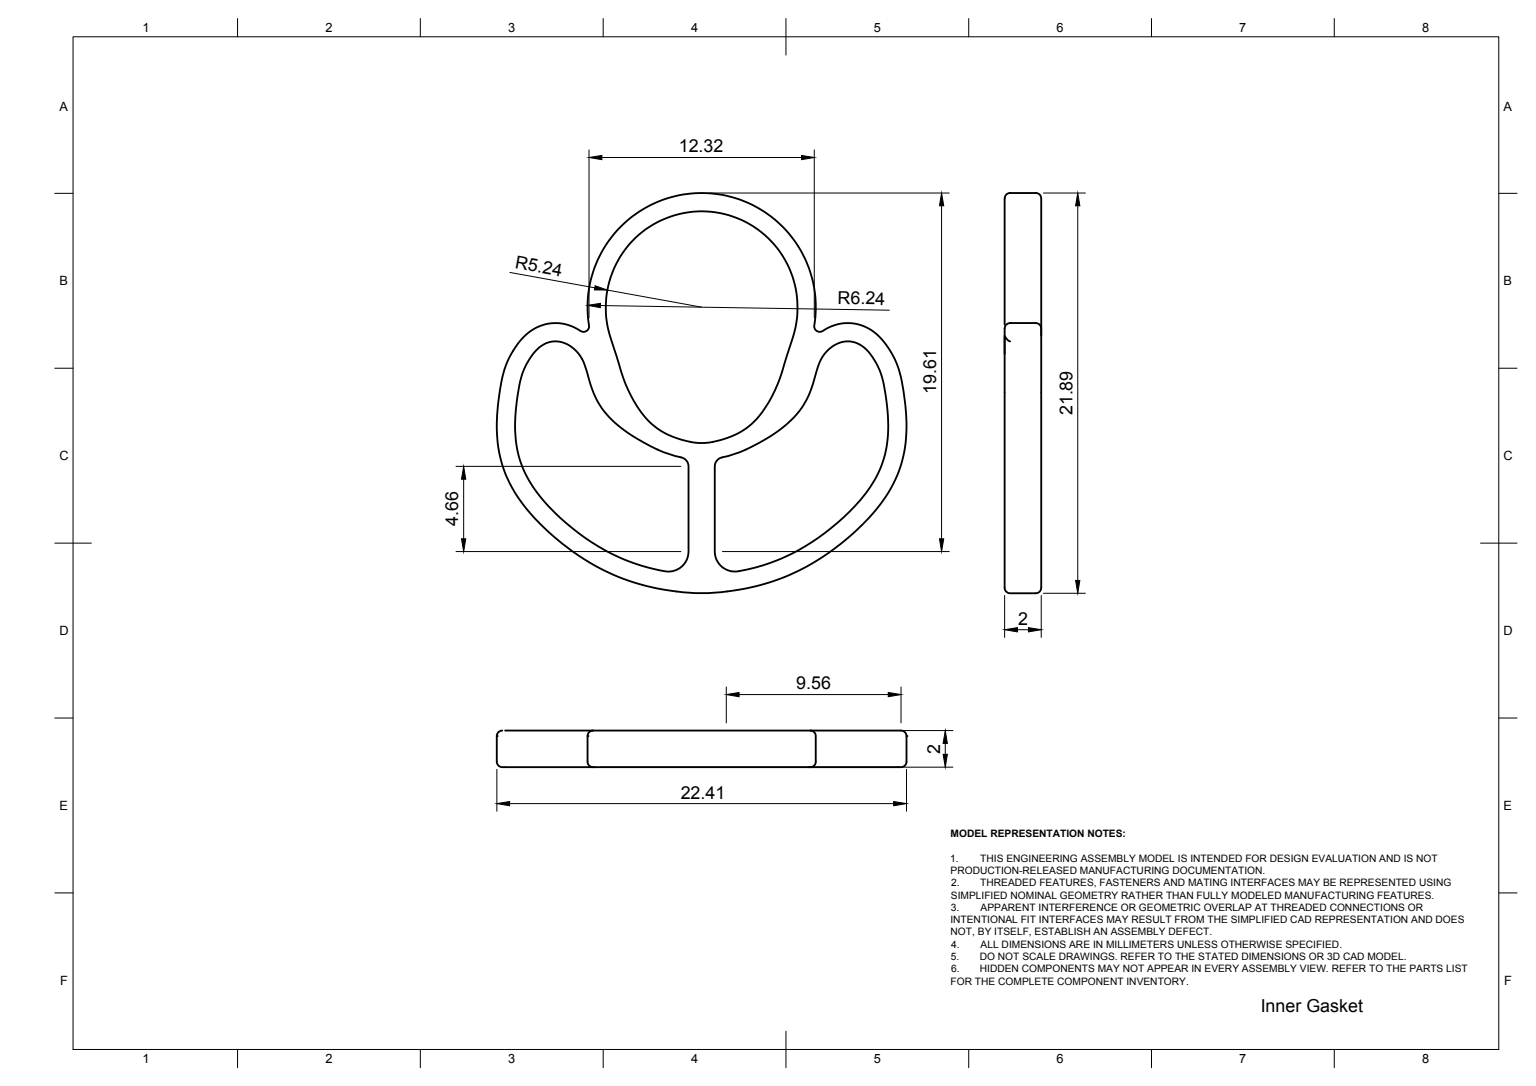
ISO-10303-21;
HEADER;
/* Generated by software containing ST-Developer
 * from STEP Tools, Inc. (www.steptools.com) 
 */

FILE_DESCRIPTION(
/* description */ ('STEP AP214'),
/* implementation_level */ '2;1');

FILE_NAME(
/* name */ 'Inner Gasket.step',
/* time_stamp */ '2026-10-06T00:19:40-07:00',
/* author */ (''),
/* organization */ (''),
/* preprocessor_version */ 'ST-DEVELOPER v20.2',
/* originating_system */ 'Autodesk Translation Framework v15.15.0.0',
/* authorisation */ '');

FILE_SCHEMA (('AUTOMOTIVE_DESIGN { 1 0 10303 214 3 1 1 }'));
ENDSEC;

DATA;
#10=MECHANICAL_DESIGN_GEOMETRIC_PRESENTATION_REPRESENTATION('',(#2065),#98302);
#483=ELLIPSE('',#34825,8.3799208131191,7.21545183497513);
#484=ELLIPSE('',#34826,4.63750951971154,3.97939150633538);
#485=ELLIPSE('',#34827,0.279111750317682,0.0287889222318791);
#486=ELLIPSE('',#34828,0.279155849620574,0.0287979766923596);
#487=ELLIPSE('',#34829,4.63750644581462,3.97938959050038);
#488=ELLIPSE('',#34830,2.90419978119635,2.54008245675797);
#489=ELLIPSE('',#34832,8.37996203818539,7.2155054701837);
#490=ELLIPSE('',#34833,4.6362036535388,3.97712799641558);
#491=ELLIPSE('',#34834,4.63620357301174,3.97712785757339);
#492=ELLIPSE('',#34835,2.90476620332758,2.54108275826229);
#493=ELLIPSE('',#34836,0.298848921430035,0.296905429574988);
#494=ELLIPSE('',#34837,0.298848915091874,0.296905425010623);
#495=ELLIPSE('',#34838,2.60097379562585,2.25500631930886);
#496=ELLIPSE('',#34839,0.298848922240667,0.296905431566661);
#497=ELLIPSE('',#34840,2.60096854257791,2.25499721056391);
#498=ELLIPSE('',#34841,0.298849077415496,0.296905613510738);
#499=ELLIPSE('',#34843,0.298848945791595,0.296905486595381);
#500=ELLIPSE('',#34844,0.298848920821335,0.296905428111335);
#501=ELLIPSE('',#34845,0.298848930247292,0.29690545026939);
#502=ELLIPSE('',#34846,0.29884892225185,0.296905431603897);
#503=ELLIPSE('',#34847,0.298848926446922,0.296905441346893);
#504=ELLIPSE('',#34848,0.298848931059905,0.296905452258441);
#505=ELLIPSE('',#34849,0.298848921910928,0.296905430717524);
#506=ELLIPSE('',#34850,0.298848923110476,0.2969054336145);
#507=ELLIPSE('',#34851,0.298848920968869,0.296905428505602);
#508=ELLIPSE('',#34852,4.93548202851956,4.27020424069084);
#509=ELLIPSE('',#34853,4.93548202854622,4.27020424073721);
#510=ELLIPSE('',#34854,0.298848930560778,0.296905451093701);
#511=ELLIPSE('',#34855,0.298848867142046,0.29690533520481);
#512=ELLIPSE('',#34856,0.29884889306055,0.296905361405062);
#513=ELLIPSE('',#34860,0.298848921989232,0.296905430886302);
#514=ELLIPSE('',#34861,0.298848931849281,0.29690545410484);
#515=ELLIPSE('',#34862,0.298848907172553,0.296905413572369);
#516=ELLIPSE('',#34863,0.298848917642298,0.296905420688533);
#517=ELLIPSE('',#34864,0.298848921443323,0.296905430437503);
#518=ELLIPSE('',#34865,0.298848921699928,0.296905431123917);
#519=ELLIPSE('',#34866,0.298848934453035,0.296905460108951);
#520=ELLIPSE('',#34867,0.298848929099766,0.296905447642822);
#521=ELLIPSE('',#34868,0.298848923421217,0.296905434233442);
#522=ELLIPSE('',#34869,2.60895186279743,2.25339178646564);
#523=ELLIPSE('',#34870,2.60895186279368,2.25339178645907);
#524=ELLIPSE('',#34871,0.298848908378948,0.296905399041772);
#525=ELLIPSE('',#34872,0.298848920956384,0.296905429882047);
#526=ELLIPSE('',#34873,0.298848920542523,0.29690542750572);
#527=ELLIPSE('',#34874,0.298848922234712,0.296905431547994);
#528=ELLIPSE('',#34875,0.298848922247508,0.296905431596198);
#529=ELLIPSE('',#34876,0.298848920242847,0.296905428747462);
#530=ELLIPSE('',#34877,0.298848966327266,0.296905496668989);
#531=ELLIPSE('',#34878,0.298849039002102,0.296905705367311);
#532=ELLIPSE('',#34879,0.29884891584007,0.296905416549116);
#533=ELLIPSE('',#34880,0.29884892201266,0.296905430947192);
#534=ELLIPSE('',#34881,2.60146235146488,2.25585351865204);
#535=ELLIPSE('',#34882,2.60146235146488,2.25585351865204);
#536=ELLIPSE('',#34883,0.298848922283708,0.296905431682282);
#537=ELLIPSE('',#34886,0.298848921993761,0.296905430900167);
#538=ELLIPSE('',#34888,0.298848922246914,0.296905431583466);
#539=ELLIPSE('',#34890,0.298848844698996,0.29690524961801);
#540=ELLIPSE('',#34891,0.298848922270607,0.296905431629623);
#541=ELLIPSE('',#34892,0.298848920959998,0.296905428481053);
#542=ELLIPSE('',#34893,4.93548202854677,4.27020424073817);
#543=ELLIPSE('',#34894,4.93548202854677,4.27020424073817);
#544=ELLIPSE('',#34895,0.298848930553665,0.29690545107324);
#545=ELLIPSE('',#34896,0.298848903185399,0.296905386777569);
#546=ELLIPSE('',#34897,0.298848895686848,0.296905369235784);
#547=ELLIPSE('',#34898,0.298848888559201,0.296905352560715);
#548=ELLIPSE('',#34899,0.298848922192621,0.296905431506102);
#549=ELLIPSE('',#34900,0.298848921998645,0.296905430922456);
#550=ELLIPSE('',#34901,0.298848922257891,0.296905431618786);
#551=ELLIPSE('',#34902,0.298848922085066,0.296905431050029);
#552=ELLIPSE('',#34903,0.298848921299427,0.296905430686572);
#553=ELLIPSE('',#34904,0.298848903202731,0.296905386834583);
#554=ELLIPSE('',#34905,0.298848888580021,0.296905352625924);
#555=ELLIPSE('',#34906,0.298848921981868,0.296905430864804);
#556=ELLIPSE('',#34907,0.298848909286409,0.296905401179665);
#557=ELLIPSE('',#34908,0.298848920591055,0.296905427635518);
#558=ELLIPSE('',#34909,0.298848922344033,0.296905431832649);
#559=ELLIPSE('',#34910,0.298848921961888,0.296905430820688);
#560=ELLIPSE('',#34911,0.298848922215141,0.296905431504259);
#561=ELLIPSE('',#34912,0.298848922001989,0.296905430644444);
#562=ELLIPSE('',#34913,0.298848941683903,0.296905477135918);
#563=ELLIPSE('',#34914,0.29884892196829,0.296905430801925);
#564=ELLIPSE('',#34915,8.67731949920772,7.50537904899086);
#565=ELLIPSE('',#34916,0.298848909045585,0.29690540101209);
#566=ELLIPSE('',#34917,8.67731949917931,7.50537904894157);
#567=ELLIPSE('',#34918,0.298848902335981,0.296905383066002);
#568=ELLIPSE('',#34919,0.298848920767452,0.296905427460604);
#976=B_SPLINE_SURFACE_WITH_KNOTS('',5,5,((#63396,#63397,#63398,#63399,#63400,
#63401),(#63402,#63403,#63404,#63405,#63406,#63407),(#63408,#63409,#63410,
#63411,#63412,#63413),(#63414,#63415,#63416,#63417,#63418,#63419),(#63420,
#63421,#63422,#63423,#63424,#63425),(#63426,#63427,#63428,#63429,#63430,
#63431),(#63432,#63433,#63434,#63435,#63436,#63437),(#63438,#63439,#63440,
#63441,#63442,#63443),(#63444,#63445,#63446,#63447,#63448,#63449)),
 .UNSPECIFIED.,.F.,.F.,.F.,(6,3,6),(6,6),(0.168109267782,0.19381333378,
0.219517399778),(0.,0.3),.UNSPECIFIED.);
#977=B_SPLINE_SURFACE_WITH_KNOTS('',5,5,((#63455,#63456,#63457,#63458,#63459,
#63460),(#63461,#63462,#63463,#63464,#63465,#63466),(#63467,#63468,#63469,
#63470,#63471,#63472),(#63473,#63474,#63475,#63476,#63477,#63478),(#63479,
#63480,#63481,#63482,#63483,#63484),(#63485,#63486,#63487,#63488,#63489,
#63490)),.UNSPECIFIED.,.F.,.F.,.F.,(6,6),(6,6),(0.167763693398,0.219167536347),
(0.,0.3),.UNSPECIFIED.);
#978=B_SPLINE_SURFACE_WITH_KNOTS('',5,5,((#63499,#63500,#63501,#63502,#63503,
#63504),(#63505,#63506,#63507,#63508,#63509,#63510),(#63511,#63512,#63513,
#63514,#63515,#63516),(#63517,#63518,#63519,#63520,#63521,#63522),(#63523,
#63524,#63525,#63526,#63527,#63528),(#63529,#63530,#63531,#63532,#63533,
#63534),(#63535,#63536,#63537,#63538,#63539,#63540),(#63541,#63542,#63543,
#63544,#63545,#63546),(#63547,#63548,#63549,#63550,#63551,#63552),(#63553,
#63554,#63555,#63556,#63557,#63558),(#63559,#63560,#63561,#63562,#63563,
#63564),(#63565,#63566,#63567,#63568,#63569,#63570),(#63571,#63572,#63573,
#63574,#63575,#63576),(#63577,#63578,#63579,#63580,#63581,#63582),(#63583,
#63584,#63585,#63586,#63587,#63588),(#63589,#63590,#63591,#63592,#63593,
#63594),(#63595,#63596,#63597,#63598,#63599,#63600),(#63601,#63602,#63603,
#63604,#63605,#63606)),.UNSPECIFIED.,.F.,.F.,.F.,(6,3,3,3,3,6),(6,6),(16.6199171728,
22.5384106111,30.5763256225,36.3852909182,40.8836102145,50.0065308028),
(0.,0.3),.UNSPECIFIED.);
#979=B_SPLINE_SURFACE_WITH_KNOTS('',5,5,((#63633,#63634,#63635,#63636,#63637,
#63638),(#63639,#63640,#63641,#63642,#63643,#63644),(#63645,#63646,#63647,
#63648,#63649,#63650),(#63651,#63652,#63653,#63654,#63655,#63656),(#63657,
#63658,#63659,#63660,#63661,#63662),(#63663,#63664,#63665,#63666,#63667,
#63668),(#63669,#63670,#63671,#63672,#63673,#63674),(#63675,#63676,#63677,
#63678,#63679,#63680),(#63681,#63682,#63683,#63684,#63685,#63686),(#63687,
#63688,#63689,#63690,#63691,#63692),(#63693,#63694,#63695,#63696,#63697,
#63698),(#63699,#63700,#63701,#63702,#63703,#63704),(#63705,#63706,#63707,
#63708,#63709,#63710),(#63711,#63712,#63713,#63714,#63715,#63716),(#63717,
#63718,#63719,#63720,#63721,#63722),(#63723,#63724,#63725,#63726,#63727,
#63728),(#63729,#63730,#63731,#63732,#63733,#63734),(#63735,#63736,#63737,
#63738,#63739,#63740)),.UNSPECIFIED.,.F.,.F.,.F.,(6,3,3,3,3,6),(6,6),(12.5665153309,
21.1100928391,29.3112279304,33.9967366188,38.6616814006,45.9550550567),
(0.,0.3),.UNSPECIFIED.);
#980=B_SPLINE_SURFACE_WITH_KNOTS('',5,1,((#63864,#63865),(#63866,#63867),
(#63868,#63869),(#63870,#63871),(#63872,#63873),(#63874,#63875),(#63876,
#63877),(#63878,#63879),(#63880,#63881),(#63882,#63883),(#63884,#63885),
(#63886,#63887),(#63888,#63889),(#63890,#63891),(#63892,#63893),(#63894,
#63895),(#63896,#63897),(#63898,#63899),(#63900,#63901),(#63902,#63903),
(#63904,#63905),(#63906,#63907),(#63908,#63909),(#63910,#63911)),
 .UNSPECIFIED.,.F.,.F.,.F.,(6,3,3,3,3,3,3,6),(2,2),(7.96998083279,14.7982954236,
17.0693303053,21.6304346192,24.5117412112,26.3698077055,28.2289298688,30.7490985197),
(0.,0.168000000000001),.UNSPECIFIED.);
#981=B_SPLINE_SURFACE_WITH_KNOTS('',5,5,((#63913,#63914,#63915,#63916,#63917,
#63918),(#63919,#63920,#63921,#63922,#63923,#63924),(#63925,#63926,#63927,
#63928,#63929,#63930),(#63931,#63932,#63933,#63934,#63935,#63936),(#63937,
#63938,#63939,#63940,#63941,#63942),(#63943,#63944,#63945,#63946,#63947,
#63948),(#63949,#63950,#63951,#63952,#63953,#63954),(#63955,#63956,#63957,
#63958,#63959,#63960),(#63961,#63962,#63963,#63964,#63965,#63966)),
 .UNSPECIFIED.,.F.,.F.,.F.,(6,3,6),(6,6),(2.81282962644,5.03686033438,7.40331879449),
(0.,0.3),.UNSPECIFIED.);
#982=B_SPLINE_SURFACE_WITH_KNOTS('',5,5,((#64024,#64025,#64026,#64027,#64028,
#64029),(#64030,#64031,#64032,#64033,#64034,#64035),(#64036,#64037,#64038,
#64039,#64040,#64041),(#64042,#64043,#64044,#64045,#64046,#64047),(#64048,
#64049,#64050,#64051,#64052,#64053),(#64054,#64055,#64056,#64057,#64058,
#64059),(#64060,#64061,#64062,#64063,#64064,#64065),(#64066,#64067,#64068,
#64069,#64070,#64071),(#64072,#64073,#64074,#64075,#64076,#64077)),
 .UNSPECIFIED.,.F.,.F.,.F.,(6,3,6),(6,6),(2.10740882,4.45303692778,6.6978412202),
(0.,0.3),.UNSPECIFIED.);
#983=B_SPLINE_SURFACE_WITH_KNOTS('',5,1,((#64089,#64090),(#64091,#64092),
(#64093,#64094),(#64095,#64096),(#64097,#64098),(#64099,#64100),(#64101,
#64102),(#64103,#64104),(#64105,#64106),(#64107,#64108),(#64109,#64110),
(#64111,#64112)),.UNSPECIFIED.,.F.,.F.,.F.,(6,3,3,6),(2,2),(1.44955812073,
3.05666068068,3.70866677692,4.6795923245),(0.,0.168000000000001),
 .UNSPECIFIED.);
#984=B_SPLINE_SURFACE_WITH_KNOTS('',5,5,((#64114,#64115,#64116,#64117,#64118,
#64119),(#64120,#64121,#64122,#64123,#64124,#64125),(#64126,#64127,#64128,
#64129,#64130,#64131),(#64132,#64133,#64134,#64135,#64136,#64137),(#64138,
#64139,#64140,#64141,#64142,#64143),(#64144,#64145,#64146,#64147,#64148,
#64149),(#64150,#64151,#64152,#64153,#64154,#64155),(#64156,#64157,#64158,
#64159,#64160,#64161),(#64162,#64163,#64164,#64165,#64166,#64167),(#64168,
#64169,#64170,#64171,#64172,#64173),(#64174,#64175,#64176,#64177,#64178,
#64179),(#64180,#64181,#64182,#64183,#64184,#64185),(#64186,#64187,#64188,
#64189,#64190,#64191),(#64192,#64193,#64194,#64195,#64196,#64197),(#64198,
#64199,#64200,#64201,#64202,#64203)),.UNSPECIFIED.,.F.,.F.,.F.,(6,3,3,3,
6),(6,6),(2.88912209896,5.1429678095,7.13061874999,9.13254225469,11.2103678193),
(0.,0.3),.UNSPECIFIED.);
#985=B_SPLINE_SURFACE_WITH_KNOTS('',5,5,((#64315,#64316,#64317,#64318,#64319,
#64320),(#64321,#64322,#64323,#64324,#64325,#64326),(#64327,#64328,#64329,
#64330,#64331,#64332),(#64333,#64334,#64335,#64336,#64337,#64338),(#64339,
#64340,#64341,#64342,#64343,#64344),(#64345,#64346,#64347,#64348,#64349,
#64350),(#64351,#64352,#64353,#64354,#64355,#64356),(#64357,#64358,#64359,
#64360,#64361,#64362),(#64363,#64364,#64365,#64366,#64367,#64368),(#64369,
#64370,#64371,#64372,#64373,#64374),(#64375,#64376,#64377,#64378,#64379,
#64380),(#64381,#64382,#64383,#64384,#64385,#64386),(#64387,#64388,#64389,
#64390,#64391,#64392),(#64393,#64394,#64395,#64396,#64397,#64398),(#64399,
#64400,#64401,#64402,#64403,#64404)),.UNSPECIFIED.,.F.,.F.,.F.,(6,3,3,3,
6),(6,6),(3.85983652914,5.49553262739,7.77935654812,9.92881869084,12.1812673196),
(0.,0.3),.UNSPECIFIED.);
#986=B_SPLINE_SURFACE_WITH_KNOTS('',5,1,((#64422,#64423),(#64424,#64425),
(#64426,#64427),(#64428,#64429),(#64430,#64431),(#64432,#64433),(#64434,
#64435),(#64436,#64437),(#64438,#64439),(#64440,#64441),(#64442,#64443),
(#64444,#64445),(#64446,#64447),(#64448,#64449),(#64450,#64451),(#64452,
#64453),(#64454,#64455),(#64456,#64457),(#64458,#64459),(#64460,#64461),
(#64462,#64463),(#64464,#64465),(#64466,#64467),(#64468,#64469)),
 .UNSPECIFIED.,.F.,.F.,.F.,(6,3,3,3,3,3,3,6),(2,2),(1.38821963106,1.92901664016,
2.47239764086,3.02881582981,3.59314912291,4.73969819441,5.30964375821,6.97732526363),
(0.,0.168000000000001),.UNSPECIFIED.);
#987=B_SPLINE_SURFACE_WITH_KNOTS('',5,5,((#64471,#64472,#64473,#64474,#64475,
#64476),(#64477,#64478,#64479,#64480,#64481,#64482),(#64483,#64484,#64485,
#64486,#64487,#64488),(#64489,#64490,#64491,#64492,#64493,#64494),(#64495,
#64496,#64497,#64498,#64499,#64500),(#64501,#64502,#64503,#64504,#64505,
#64506),(#64507,#64508,#64509,#64510,#64511,#64512),(#64513,#64514,#64515,
#64516,#64517,#64518),(#64519,#64520,#64521,#64522,#64523,#64524),(#64525,
#64526,#64527,#64528,#64529,#64530),(#64531,#64532,#64533,#64534,#64535,
#64536),(#64537,#64538,#64539,#64540,#64541,#64542),(#64543,#64544,#64545,
#64546,#64547,#64548),(#64549,#64550,#64551,#64552,#64553,#64554),(#64555,
#64556,#64557,#64558,#64559,#64560),(#64561,#64562,#64563,#64564,#64565,
#64566),(#64567,#64568,#64569,#64570,#64571,#64572),(#64573,#64574,#64575,
#64576,#64577,#64578),(#64579,#64580,#64581,#64582,#64583,#64584),(#64585,
#64586,#64587,#64588,#64589,#64590),(#64591,#64592,#64593,#64594,#64595,
#64596),(#64597,#64598,#64599,#64600,#64601,#64602),(#64603,#64604,#64605,
#64606,#64607,#64608),(#64609,#64610,#64611,#64612,#64613,#64614)),
 .UNSPECIFIED.,.F.,.F.,.F.,(6,3,3,3,3,3,3,6),(6,6),(2.49496263694,3.75614411414,
4.32934465344,5.25874047989,6.18762608197,8.03803358836,9.88322107258,15.7678954384),
(0.,0.3),.UNSPECIFIED.);
#988=B_SPLINE_SURFACE_WITH_KNOTS('',5,5,((#64753,#64754,#64755,#64756,#64757,
#64758),(#64759,#64760,#64761,#64762,#64763,#64764),(#64765,#64766,#64767,
#64768,#64769,#64770),(#64771,#64772,#64773,#64774,#64775,#64776),(#64777,
#64778,#64779,#64780,#64781,#64782),(#64783,#64784,#64785,#64786,#64787,
#64788),(#64789,#64790,#64791,#64792,#64793,#64794),(#64795,#64796,#64797,
#64798,#64799,#64800),(#64801,#64802,#64803,#64804,#64805,#64806),(#64807,
#64808,#64809,#64810,#64811,#64812),(#64813,#64814,#64815,#64816,#64817,
#64818),(#64819,#64820,#64821,#64822,#64823,#64824),(#64825,#64826,#64827,
#64828,#64829,#64830),(#64831,#64832,#64833,#64834,#64835,#64836),(#64837,
#64838,#64839,#64840,#64841,#64842),(#64843,#64844,#64845,#64846,#64847,
#64848),(#64849,#64850,#64851,#64852,#64853,#64854),(#64855,#64856,#64857,
#64858,#64859,#64860)),.UNSPECIFIED.,.F.,.F.,.F.,(6,3,3,3,3,6),(6,6),(4.00115394842,
11.4721831186,13.451526058,14.4455167529,15.8981054324,17.2738332784),(0.,
0.3),.UNSPECIFIED.);
#989=B_SPLINE_SURFACE_WITH_KNOTS('',5,1,((#64881,#64882),(#64883,#64884),
(#64885,#64886),(#64887,#64888),(#64889,#64890),(#64891,#64892),(#64893,
#64894),(#64895,#64896),(#64897,#64898),(#64899,#64900),(#64901,#64902),
(#64903,#64904),(#64905,#64906),(#64907,#64908),(#64909,#64910),(#64911,
#64912),(#64913,#64914),(#64915,#64916)),.UNSPECIFIED.,.F.,.F.,.F.,(6,3,
3,3,3,6),(2,2),(2.30144058436,3.21523268549,4.17948834992,7.86941426972,
10.6293166988,11.5241632533),(0.,0.168000000000001),.UNSPECIFIED.);
#990=B_SPLINE_SURFACE_WITH_KNOTS('',5,5,((#64918,#64919,#64920,#64921,#64922,
#64923),(#64924,#64925,#64926,#64927,#64928,#64929),(#64930,#64931,#64932,
#64933,#64934,#64935),(#64936,#64937,#64938,#64939,#64940,#64941),(#64942,
#64943,#64944,#64945,#64946,#64947),(#64948,#64949,#64950,#64951,#64952,
#64953),(#64954,#64955,#64956,#64957,#64958,#64959),(#64960,#64961,#64962,
#64963,#64964,#64965),(#64966,#64967,#64968,#64969,#64970,#64971)),
 .UNSPECIFIED.,.F.,.F.,.F.,(6,3,6),(6,6),(1.35769229991,2.30681875984,3.25594521977),
(0.,0.3),.UNSPECIFIED.);
#991=B_SPLINE_SURFACE_WITH_KNOTS('',5,5,((#64975,#64976,#64977,#64978,#64979,
#64980),(#64981,#64982,#64983,#64984,#64985,#64986),(#64987,#64988,#64989,
#64990,#64991,#64992),(#64993,#64994,#64995,#64996,#64997,#64998),(#64999,
#65000,#65001,#65002,#65003,#65004),(#65005,#65006,#65007,#65008,#65009,
#65010),(#65011,#65012,#65013,#65014,#65015,#65016),(#65017,#65018,#65019,
#65020,#65021,#65022),(#65023,#65024,#65025,#65026,#65027,#65028)),
 .UNSPECIFIED.,.F.,.F.,.F.,(6,3,6),(6,6),(1.35799881012,2.30712712606,3.25625544201),
(0.,0.3),.UNSPECIFIED.);
#992=B_SPLINE_SURFACE_WITH_KNOTS('',5,1,((#65032,#65033),(#65034,#65035),
(#65036,#65037),(#65038,#65039),(#65040,#65041),(#65042,#65043)),
 .UNSPECIFIED.,.F.,.F.,.F.,(6,6),(2,2),(0.96552770951,2.34485300881),(0.,
0.168000000000001),.UNSPECIFIED.);
#993=B_SPLINE_SURFACE_WITH_KNOTS('',5,5,((#65045,#65046,#65047,#65048,#65049,
#65050),(#65051,#65052,#65053,#65054,#65055,#65056),(#65057,#65058,#65059,
#65060,#65061,#65062),(#65063,#65064,#65065,#65066,#65067,#65068),(#65069,
#65070,#65071,#65072,#65073,#65074),(#65075,#65076,#65077,#65078,#65079,
#65080),(#65081,#65082,#65083,#65084,#65085,#65086),(#65087,#65088,#65089,
#65090,#65091,#65092),(#65093,#65094,#65095,#65096,#65097,#65098)),
 .UNSPECIFIED.,.F.,.F.,.F.,(6,3,6),(6,6),(0.591273571839,1.32390886326,
1.88642093473),(0.,0.3),.UNSPECIFIED.);
#994=B_SPLINE_SURFACE_WITH_KNOTS('',5,5,((#65107,#65108,#65109,#65110,#65111,
#65112),(#65113,#65114,#65115,#65116,#65117,#65118),(#65119,#65120,#65121,
#65122,#65123,#65124),(#65125,#65126,#65127,#65128,#65129,#65130),(#65131,
#65132,#65133,#65134,#65135,#65136),(#65137,#65138,#65139,#65140,#65141,
#65142),(#65143,#65144,#65145,#65146,#65147,#65148),(#65149,#65150,#65151,
#65152,#65153,#65154),(#65155,#65156,#65157,#65158,#65159,#65160)),
 .UNSPECIFIED.,.F.,.F.,.F.,(6,3,6),(6,6),(0.591154687012,1.24895024918,
1.88603455695),(0.,0.3),.UNSPECIFIED.);
#995=B_SPLINE_SURFACE_WITH_KNOTS('',5,1,((#65172,#65173),(#65174,#65175),
(#65176,#65177),(#65178,#65179),(#65180,#65181),(#65182,#65183)),
 .UNSPECIFIED.,.F.,.F.,.F.,(6,6),(2,2),(0.493788369863,1.19920032681),(0.,
0.168000000000001),.UNSPECIFIED.);
#996=B_SPLINE_SURFACE_WITH_KNOTS('',5,5,((#65255,#65256,#65257,#65258,#65259,
#65260),(#65261,#65262,#65263,#65264,#65265,#65266),(#65267,#65268,#65269,
#65270,#65271,#65272),(#65273,#65274,#65275,#65276,#65277,#65278),(#65279,
#65280,#65281,#65282,#65283,#65284),(#65285,#65286,#65287,#65288,#65289,
#65290),(#65291,#65292,#65293,#65294,#65295,#65296),(#65297,#65298,#65299,
#65300,#65301,#65302),(#65303,#65304,#65305,#65306,#65307,#65308)),
 .UNSPECIFIED.,.F.,.F.,.F.,(6,3,6),(6,6),(1.56059358548,2.9568323585,4.75555213266),
(0.,0.3),.UNSPECIFIED.);
#997=B_SPLINE_SURFACE_WITH_KNOTS('',5,5,((#65361,#65362,#65363,#65364,#65365,
#65366),(#65367,#65368,#65369,#65370,#65371,#65372),(#65373,#65374,#65375,
#65376,#65377,#65378),(#65379,#65380,#65381,#65382,#65383,#65384),(#65385,
#65386,#65387,#65388,#65389,#65390),(#65391,#65392,#65393,#65394,#65395,
#65396),(#65397,#65398,#65399,#65400,#65401,#65402),(#65403,#65404,#65405,
#65406,#65407,#65408),(#65409,#65410,#65411,#65412,#65413,#65414)),
 .UNSPECIFIED.,.F.,.F.,.F.,(6,3,6),(6,6),(1.62520881516,3.23201031665,4.82017891154),
(0.,0.3),.UNSPECIFIED.);
#998=B_SPLINE_SURFACE_WITH_KNOTS('',5,1,((#65421,#65422),(#65423,#65424),
(#65425,#65426),(#65427,#65428),(#65429,#65430),(#65431,#65432)),
 .UNSPECIFIED.,.F.,.F.,.F.,(6,6),(2,2),(1.41662542015,3.44037602036),(0.,
0.168000000000001),.UNSPECIFIED.);
#999=B_SPLINE_SURFACE_WITH_KNOTS('',5,5,((#65433,#65434,#65435,#65436,#65437,
#65438),(#65439,#65440,#65441,#65442,#65443,#65444),(#65445,#65446,#65447,
#65448,#65449,#65450),(#65451,#65452,#65453,#65454,#65455,#65456),(#65457,
#65458,#65459,#65460,#65461,#65462),(#65463,#65464,#65465,#65466,#65467,
#65468),(#65469,#65470,#65471,#65472,#65473,#65474),(#65475,#65476,#65477,
#65478,#65479,#65480),(#65481,#65482,#65483,#65484,#65485,#65486)),
 .UNSPECIFIED.,.F.,.F.,.F.,(6,3,6),(6,6),(3.6079177031,7.76832519582,12.1678629797),
(0.,0.3),.UNSPECIFIED.);
#1000=B_SPLINE_SURFACE_WITH_KNOTS('',5,5,((#65508,#65509,#65510,#65511,
#65512,#65513),(#65514,#65515,#65516,#65517,#65518,#65519),(#65520,#65521,
#65522,#65523,#65524,#65525),(#65526,#65527,#65528,#65529,#65530,#65531),
(#65532,#65533,#65534,#65535,#65536,#65537),(#65538,#65539,#65540,#65541,
#65542,#65543),(#65544,#65545,#65546,#65547,#65548,#65549),(#65550,#65551,
#65552,#65553,#65554,#65555),(#65556,#65557,#65558,#65559,#65560,#65561)),
 .UNSPECIFIED.,.F.,.F.,.F.,(6,3,6),(6,6),(5.26262328413,9.35737491835,13.8219121669),
(0.,0.3),.UNSPECIFIED.);
#1001=B_SPLINE_SURFACE_WITH_KNOTS('',5,1,((#65583,#65584),(#65585,#65586),
(#65587,#65588),(#65589,#65590),(#65591,#65592),(#65593,#65594),(#65595,
#65596),(#65597,#65598),(#65599,#65600),(#65601,#65602),(#65603,#65604),
(#65605,#65606),(#65607,#65608),(#65609,#65610),(#65611,#65612),(#65613,
#65614),(#65615,#65616)),.UNSPECIFIED.,.F.,.F.,.F.,(6,5,3,3,6),(2,2),(1.81082989417716,
1.81130449228,3.02278054545,4.81654635721,7.83913682071),(0.,0.168000000000001),
 .UNSPECIFIED.);
#1002=B_SPLINE_SURFACE_WITH_KNOTS('',5,5,((#65619,#65620,#65621,#65622,
#65623,#65624),(#65625,#65626,#65627,#65628,#65629,#65630),(#65631,#65632,
#65633,#65634,#65635,#65636),(#65637,#65638,#65639,#65640,#65641,#65642),
(#65643,#65644,#65645,#65646,#65647,#65648),(#65649,#65650,#65651,#65652,
#65653,#65654),(#65655,#65656,#65657,#65658,#65659,#65660),(#65661,#65662,
#65663,#65664,#65665,#65666),(#65667,#65668,#65669,#65670,#65671,#65672)),
 .UNSPECIFIED.,.F.,.F.,.F.,(6,3,6),(6,6),(6.65601718416,11.623259991,18.3853430669),
(0.,0.3),.UNSPECIFIED.);
#1003=B_SPLINE_SURFACE_WITH_KNOTS('',5,5,((#65681,#65682,#65683,#65684,
#65685,#65686),(#65687,#65688,#65689,#65690,#65691,#65692),(#65693,#65694,
#65695,#65696,#65697,#65698),(#65699,#65700,#65701,#65702,#65703,#65704),
(#65705,#65706,#65707,#65708,#65709,#65710),(#65711,#65712,#65713,#65714,
#65715,#65716),(#65717,#65718,#65719,#65720,#65721,#65722),(#65723,#65724,
#65725,#65726,#65727,#65728),(#65729,#65730,#65731,#65732,#65733,#65734)),
 .UNSPECIFIED.,.F.,.F.,.F.,(6,3,6),(6,6),(6.65635355468,12.3414051375,18.3857494183),
(0.,0.3),.UNSPECIFIED.);
#1004=B_SPLINE_SURFACE_WITH_KNOTS('',5,1,((#65748,#65749),(#65750,#65751),
(#65752,#65753),(#65754,#65755),(#65756,#65757),(#65758,#65759)),
 .UNSPECIFIED.,.F.,.F.,.F.,(6,6),(2,2),(5.84195403358,14.187602653),(0.,
0.168000000000001),.UNSPECIFIED.);
#1005=B_SPLINE_SURFACE_WITH_KNOTS('',5,5,((#65761,#65762,#65763,#65764,
#65765,#65766),(#65767,#65768,#65769,#65770,#65771,#65772),(#65773,#65774,
#65775,#65776,#65777,#65778),(#65779,#65780,#65781,#65782,#65783,#65784),
(#65785,#65786,#65787,#65788,#65789,#65790),(#65791,#65792,#65793,#65794,
#65795,#65796),(#65797,#65798,#65799,#65800,#65801,#65802),(#65803,#65804,
#65805,#65806,#65807,#65808),(#65809,#65810,#65811,#65812,#65813,#65814)),
 .UNSPECIFIED.,.F.,.F.,.F.,(6,3,6),(6,6),(6.656059514,12.5206580023,18.3855563608),
(0.,0.3),.UNSPECIFIED.);
#1006=B_SPLINE_SURFACE_WITH_KNOTS('',5,5,((#65872,#65873,#65874,#65875,
#65876,#65877),(#65878,#65879,#65880,#65881,#65882,#65883),(#65884,#65885,
#65886,#65887,#65888,#65889),(#65890,#65891,#65892,#65893,#65894,#65895),
(#65896,#65897,#65898,#65899,#65900,#65901),(#65902,#65903,#65904,#65905,
#65906,#65907),(#65908,#65909,#65910,#65911,#65912,#65913),(#65914,#65915,
#65916,#65917,#65918,#65919),(#65920,#65921,#65922,#65923,#65924,#65925)),
 .UNSPECIFIED.,.F.,.F.,.F.,(6,3,6),(6,6),(6.65611545055,12.5207139017,18.3856123466),
(0.,0.3),.UNSPECIFIED.);
#1007=B_SPLINE_SURFACE_WITH_KNOTS('',5,1,((#65983,#65984),(#65985,#65986),
(#65987,#65988),(#65989,#65990),(#65991,#65992),(#65993,#65994)),
 .UNSPECIFIED.,.F.,.F.,.F.,(6,6),(2,2),(5.84195403358,14.187602653),(0.,
0.168000000000001),.UNSPECIFIED.);
#1008=B_SPLINE_SURFACE_WITH_KNOTS('',5,5,((#65996,#65997,#65998,#65999,
#66000,#66001),(#66002,#66003,#66004,#66005,#66006,#66007),(#66008,#66009,
#66010,#66011,#66012,#66013),(#66014,#66015,#66016,#66017,#66018,#66019),
(#66020,#66021,#66022,#66023,#66024,#66025),(#66026,#66027,#66028,#66029,
#66030,#66031),(#66032,#66033,#66034,#66035,#66036,#66037),(#66038,#66039,
#66040,#66041,#66042,#66043),(#66044,#66045,#66046,#66047,#66048,#66049),
(#66050,#66051,#66052,#66053,#66054,#66055),(#66056,#66057,#66058,#66059,
#66060,#66061),(#66062,#66063,#66064,#66065,#66066,#66067),(#66068,#66069,
#66070,#66071,#66072,#66073),(#66074,#66075,#66076,#66077,#66078,#66079)),
 .UNSPECIFIED.,.F.,.F.,.F.,(6,3,5,6),(6,6),(5.26516274934,9.50401785273,
13.8254388584,13.9110416194906),(0.,0.3),.UNSPECIFIED.);
#1009=B_SPLINE_SURFACE_WITH_KNOTS('',5,5,((#66094,#66095,#66096,#66097,
#66098,#66099),(#66100,#66101,#66102,#66103,#66104,#66105),(#66106,#66107,
#66108,#66109,#66110,#66111),(#66112,#66113,#66114,#66115,#66116,#66117),
(#66118,#66119,#66120,#66121,#66122,#66123),(#66124,#66125,#66126,#66127,
#66128,#66129),(#66130,#66131,#66132,#66133,#66134,#66135),(#66136,#66137,
#66138,#66139,#66140,#66141),(#66142,#66143,#66144,#66145,#66146,#66147)),
 .UNSPECIFIED.,.F.,.F.,.F.,(6,3,6),(6,6),(3.60712399577,7.99998279071,12.1666998724),
(0.,0.3),.UNSPECIFIED.);
#1010=B_SPLINE_SURFACE_WITH_KNOTS('',5,1,((#66225,#66226),(#66227,#66228),
(#66229,#66230),(#66231,#66232),(#66233,#66234),(#66235,#66236),(#66237,
#66238),(#66239,#66240),(#66241,#66242),(#66243,#66244),(#66245,#66246),
(#66247,#66248)),.UNSPECIFIED.,.F.,.F.,.F.,(6,3,3,6),(2,2),(2.71670313018,
5.73911718302,7.53277830329,8.74418364899),(0.,0.168000000000001),
 .UNSPECIFIED.);
#1011=B_SPLINE_SURFACE_WITH_KNOTS('',5,5,((#66250,#66251,#66252,#66253,
#66254,#66255),(#66256,#66257,#66258,#66259,#66260,#66261),(#66262,#66263,
#66264,#66265,#66266,#66267),(#66268,#66269,#66270,#66271,#66272,#66273),
(#66274,#66275,#66276,#66277,#66278,#66279),(#66280,#66281,#66282,#66283,
#66284,#66285),(#66286,#66287,#66288,#66289,#66290,#66291),(#66292,#66293,
#66294,#66295,#66296,#66297),(#66298,#66299,#66300,#66301,#66302,#66303),
(#66304,#66305,#66306,#66307,#66308,#66309),(#66310,#66311,#66312,#66313,
#66314,#66315),(#66316,#66317,#66318,#66319,#66320,#66321),(#66322,#66323,
#66324,#66325,#66326,#66327),(#66328,#66329,#66330,#66331,#66332,#66333),
(#66334,#66335,#66336,#66337,#66338,#66339)),.UNSPECIFIED.,.F.,.F.,.F.,
(6,3,3,3,6),(6,6),(5.22957298235,8.73373254507,11.36693316,14.9187174958,
17.8070761317),(0.,0.3),.UNSPECIFIED.);
#1012=B_SPLINE_SURFACE_WITH_KNOTS('',5,5,((#66427,#66428,#66429,#66430,
#66431,#66432),(#66433,#66434,#66435,#66436,#66437,#66438),(#66439,#66440,
#66441,#66442,#66443,#66444),(#66445,#66446,#66447,#66448,#66449,#66450),
(#66451,#66452,#66453,#66454,#66455,#66456),(#66457,#66458,#66459,#66460,
#66461,#66462),(#66463,#66464,#66465,#66466,#66467,#66468),(#66469,#66470,
#66471,#66472,#66473,#66474),(#66475,#66476,#66477,#66478,#66479,#66480),
(#66481,#66482,#66483,#66484,#66485,#66486),(#66487,#66488,#66489,#66490,
#66491,#66492),(#66493,#66494,#66495,#66496,#66497,#66498),(#66499,#66500,
#66501,#66502,#66503,#66504),(#66505,#66506,#66507,#66508,#66509,#66510),
(#66511,#66512,#66513,#66514,#66515,#66516)),.UNSPECIFIED.,.F.,.F.,.F.,
(6,3,3,3,6),(6,6),(5.19541482867,8.7224443269,11.7666783733,14.769293572,
17.772416875),(0.,0.3),.UNSPECIFIED.);
#1013=B_SPLINE_SURFACE_WITH_KNOTS('',5,1,((#66537,#66538),(#66539,#66540),
(#66541,#66542),(#66543,#66544),(#66545,#66546),(#66547,#66548),(#66549,
#66550),(#66551,#66552),(#66553,#66554),(#66555,#66556),(#66557,#66558),
(#66559,#66560),(#66561,#66562),(#66563,#66564),(#66565,#66566),(#66567,
#66568),(#66569,#66570),(#66571,#66572)),.UNSPECIFIED.,.F.,.F.,.F.,(6,3,
3,3,3,6),(2,2),(2.56814442563,4.26587753681,5.98143772792,6.84529958826,
9.44079904688,11.1645337758),(0.,0.168000000000001),.UNSPECIFIED.);
#1014=B_SPLINE_SURFACE_WITH_KNOTS('',5,5,((#66574,#66575,#66576,#66577,
#66578,#66579),(#66580,#66581,#66582,#66583,#66584,#66585),(#66586,#66587,
#66588,#66589,#66590,#66591),(#66592,#66593,#66594,#66595,#66596,#66597),
(#66598,#66599,#66600,#66601,#66602,#66603),(#66604,#66605,#66606,#66607,
#66608,#66609),(#66610,#66611,#66612,#66613,#66614,#66615),(#66616,#66617,
#66618,#66619,#66620,#66621),(#66622,#66623,#66624,#66625,#66626,#66627)),
 .UNSPECIFIED.,.F.,.F.,.F.,(6,3,6),(6,6),(1.00648613473,1.91246268912,2.81843924351),
(0.,0.3),.UNSPECIFIED.);
#1015=B_SPLINE_SURFACE_WITH_KNOTS('',5,5,((#66631,#66632,#66633,#66634,
#66635,#66636),(#66637,#66638,#66639,#66640,#66641,#66642),(#66643,#66644,
#66645,#66646,#66647,#66648),(#66649,#66650,#66651,#66652,#66653,#66654),
(#66655,#66656,#66657,#66658,#66659,#66660),(#66661,#66662,#66663,#66664,
#66665,#66666),(#66667,#66668,#66669,#66670,#66671,#66672),(#66673,#66674,
#66675,#66676,#66677,#66678),(#66679,#66680,#66681,#66682,#66683,#66684)),
 .UNSPECIFIED.,.F.,.F.,.F.,(6,3,6),(6,6),(1.00636935115,1.91235557727,2.81834180338),
(0.,0.3),.UNSPECIFIED.);
#1016=B_SPLINE_SURFACE_WITH_KNOTS('',5,1,((#66688,#66689),(#66690,#66691),
(#66692,#66693),(#66694,#66695),(#66696,#66697),(#66698,#66699)),
 .UNSPECIFIED.,.F.,.F.,.F.,(6,6),(2,2),(0.855391128886,2.07737845587),(0.,
0.168000000000001),.UNSPECIFIED.);
#1017=B_SPLINE_SURFACE_WITH_KNOTS('',5,5,((#66701,#66702,#66703,#66704,
#66705,#66706),(#66707,#66708,#66709,#66710,#66711,#66712),(#66713,#66714,
#66715,#66716,#66717,#66718),(#66719,#66720,#66721,#66722,#66723,#66724),
(#66725,#66726,#66727,#66728,#66729,#66730),(#66731,#66732,#66733,#66734,
#66735,#66736),(#66737,#66738,#66739,#66740,#66741,#66742),(#66743,#66744,
#66745,#66746,#66747,#66748),(#66749,#66750,#66751,#66752,#66753,#66754),
(#66755,#66756,#66757,#66758,#66759,#66760),(#66761,#66762,#66763,#66764,
#66765,#66766),(#66767,#66768,#66769,#66770,#66771,#66772),(#66773,#66774,
#66775,#66776,#66777,#66778),(#66779,#66780,#66781,#66782,#66783,#66784),
(#66785,#66786,#66787,#66788,#66789,#66790)),.UNSPECIFIED.,.F.,.F.,.F.,
(6,3,3,3,6),(6,6),(5.25334327713,8.78087326212,11.4506730327,14.9857329729,
17.830940375),(0.,0.3),.UNSPECIFIED.);
#1018=B_SPLINE_SURFACE_WITH_KNOTS('',5,5,((#66809,#66810,#66811,#66812,
#66813,#66814),(#66815,#66816,#66817,#66818,#66819,#66820),(#66821,#66822,
#66823,#66824,#66825,#66826),(#66827,#66828,#66829,#66830,#66831,#66832),
(#66833,#66834,#66835,#66836,#66837,#66838),(#66839,#66840,#66841,#66842,
#66843,#66844),(#66845,#66846,#66847,#66848,#66849,#66850),(#66851,#66852,
#66853,#66854,#66855,#66856),(#66857,#66858,#66859,#66860,#66861,#66862),
(#66863,#66864,#66865,#66866,#66867,#66868),(#66869,#66870,#66871,#66872,
#66873,#66874),(#66875,#66876,#66877,#66878,#66879,#66880),(#66881,#66882,
#66883,#66884,#66885,#66886),(#66887,#66888,#66889,#66890,#66891,#66892),
(#66893,#66894,#66895,#66896,#66897,#66898)),.UNSPECIFIED.,.F.,.F.,.F.,
(6,3,3,3,6),(6,6),(5.18156607379,7.64878179687,11.6904556298,14.7384492068,
17.7593366521),(0.,0.3),.UNSPECIFIED.);
#1019=B_SPLINE_SURFACE_WITH_KNOTS('',5,1,((#66917,#66918),(#66919,#66920),
(#66921,#66922),(#66923,#66924),(#66925,#66926),(#66927,#66928),(#66929,
#66930),(#66931,#66932),(#66933,#66934),(#66935,#66936),(#66937,#66938),
(#66939,#66940),(#66941,#66942),(#66943,#66944),(#66945,#66946),(#66947,
#66948),(#66949,#66950),(#66951,#66952)),.UNSPECIFIED.,.F.,.F.,.F.,(6,3,
3,3,3,6),(2,2),(2.58143959,4.30538111878,6.90119302094,7.76515862896,9.48090785315,
11.1787837181),(0.,0.168000000000001),.UNSPECIFIED.);
#1020=B_SPLINE_SURFACE_WITH_KNOTS('',5,5,((#66953,#66954,#66955,#66956,
#66957,#66958),(#66959,#66960,#66961,#66962,#66963,#66964),(#66965,#66966,
#66967,#66968,#66969,#66970),(#66971,#66972,#66973,#66974,#66975,#66976),
(#66977,#66978,#66979,#66980,#66981,#66982),(#66983,#66984,#66985,#66986,
#66987,#66988),(#66989,#66990,#66991,#66992,#66993,#66994),(#66995,#66996,
#66997,#66998,#66999,#67000),(#67001,#67002,#67003,#67004,#67005,#67006),
(#67007,#67008,#67009,#67010,#67011,#67012),(#67013,#67014,#67015,#67016,
#67017,#67018),(#67019,#67020,#67021,#67022,#67023,#67024),(#67025,#67026,
#67027,#67028,#67029,#67030),(#67031,#67032,#67033,#67034,#67035,#67036),
(#67037,#67038,#67039,#67040,#67041,#67042)),.UNSPECIFIED.,.F.,.F.,.F.,
(6,3,3,3,6),(6,6),(3.85962234114,6.1874356314,8.16908321302,10.1785749125,
12.1808522654),(0.,0.3),.UNSPECIFIED.);
#1021=B_SPLINE_SURFACE_WITH_KNOTS('',5,5,((#67071,#67072,#67073,#67074,
#67075,#67076),(#67077,#67078,#67079,#67080,#67081,#67082),(#67083,#67084,
#67085,#67086,#67087,#67088),(#67089,#67090,#67091,#67092,#67093,#67094),
(#67095,#67096,#67097,#67098,#67099,#67100),(#67101,#67102,#67103,#67104,
#67105,#67106),(#67107,#67108,#67109,#67110,#67111,#67112),(#67113,#67114,
#67115,#67116,#67117,#67118),(#67119,#67120,#67121,#67122,#67123,#67124),
(#67125,#67126,#67127,#67128,#67129,#67130),(#67131,#67132,#67133,#67134,
#67135,#67136),(#67137,#67138,#67139,#67140,#67141,#67142)),
 .UNSPECIFIED.,.F.,.F.,.F.,(6,3,3,6),(6,6),(2.76827068394,6.61192064383,
8.76054366777,11.0890194561),(0.,0.3),.UNSPECIFIED.);
#1022=B_SPLINE_SURFACE_WITH_KNOTS('',5,1,((#67159,#67160),(#67161,#67162),
(#67163,#67164),(#67165,#67166),(#67167,#67168),(#67169,#67170),(#67171,
#67172),(#67173,#67174),(#67175,#67176),(#67177,#67178),(#67179,#67180),
(#67181,#67182),(#67183,#67184),(#67185,#67186),(#67187,#67188),(#67189,
#67190),(#67191,#67192),(#67193,#67194),(#67195,#67196),(#67197,#67198),
(#67199,#67200),(#67201,#67202),(#67203,#67204),(#67205,#67206)),
 .UNSPECIFIED.,.F.,.F.,.F.,(6,3,3,3,3,3,3,6),(2,2),(1.95166187923,3.61934338467,
4.18928894847,5.33583801997,5.90017131307,6.45658950203,6.99997050268,7.54076751178),
(0.,0.168000000000001),.UNSPECIFIED.);
#1023=B_SPLINE_SURFACE_WITH_KNOTS('',5,5,((#67209,#67210,#67211,#67212,
#67213,#67214),(#67215,#67216,#67217,#67218,#67219,#67220),(#67221,#67222,
#67223,#67224,#67225,#67226),(#67227,#67228,#67229,#67230,#67231,#67232),
(#67233,#67234,#67235,#67236,#67237,#67238),(#67239,#67240,#67241,#67242,
#67243,#67244),(#67245,#67246,#67247,#67248,#67249,#67250),(#67251,#67252,
#67253,#67254,#67255,#67256),(#67257,#67258,#67259,#67260,#67261,#67262)),
 .UNSPECIFIED.,.F.,.F.,.F.,(6,3,6),(6,6),(2.24719882413,4.51381221186,6.83969663211),
(0.,0.3),.UNSPECIFIED.);
#1024=B_SPLINE_SURFACE_WITH_KNOTS('',5,5,((#67317,#67318,#67319,#67320,
#67321,#67322),(#67323,#67324,#67325,#67326,#67327,#67328),(#67329,#67330,
#67331,#67332,#67333,#67334),(#67335,#67336,#67337,#67338,#67339,#67340),
(#67341,#67342,#67343,#67344,#67345,#67346),(#67347,#67348,#67349,#67350,
#67351,#67352),(#67353,#67354,#67355,#67356,#67357,#67358),(#67359,#67360,
#67361,#67362,#67363,#67364),(#67365,#67366,#67367,#67368,#67369,#67370)),
 .UNSPECIFIED.,.F.,.F.,.F.,(6,3,6),(6,6),(2.81287993679,5.11582036754,7.40337618611),
(0.,0.3),.UNSPECIFIED.);
#1025=B_SPLINE_SURFACE_WITH_KNOTS('',5,1,((#67382,#67383),(#67384,#67385),
(#67386,#67387),(#67388,#67389),(#67390,#67391),(#67392,#67393),(#67394,
#67395),(#67396,#67397),(#67398,#67399),(#67400,#67401),(#67402,#67403),
(#67404,#67405)),.UNSPECIFIED.,.F.,.F.,.F.,(6,3,3,6),(2,2),(1.13146961455,
2.10239516213,2.75440125835,4.36150381835),(0.,0.168000000000001),
 .UNSPECIFIED.);
#1026=B_SPLINE_SURFACE_WITH_KNOTS('',5,5,((#67407,#67408,#67409,#67410,
#67411,#67412),(#67413,#67414,#67415,#67416,#67417,#67418),(#67419,#67420,
#67421,#67422,#67423,#67424),(#67425,#67426,#67427,#67428,#67429,#67430),
(#67431,#67432,#67433,#67434,#67435,#67436),(#67437,#67438,#67439,#67440,
#67441,#67442),(#67443,#67444,#67445,#67446,#67447,#67448),(#67449,#67450,
#67451,#67452,#67453,#67454),(#67455,#67456,#67457,#67458,#67459,#67460),
(#67461,#67462,#67463,#67464,#67465,#67466),(#67467,#67468,#67469,#67470,
#67471,#67472),(#67473,#67474,#67475,#67476,#67477,#67478),(#67479,#67480,
#67481,#67482,#67483,#67484),(#67485,#67486,#67487,#67488,#67489,#67490),
(#67491,#67492,#67493,#67494,#67495,#67496),(#67497,#67498,#67499,#67500,
#67501,#67502),(#67503,#67504,#67505,#67506,#67507,#67508),(#67509,#67510,
#67511,#67512,#67513,#67514)),.UNSPECIFIED.,.F.,.F.,.F.,(6,3,3,3,3,6),(6,
6),(12.5665153092,21.1100928175,29.3112276523,33.9967363407,38.6616811225,
45.9550547113),(0.,0.3),.UNSPECIFIED.);
#1027=B_SPLINE_SURFACE_WITH_KNOTS('',5,5,((#67647,#67648,#67649,#67650,
#67651,#67652),(#67653,#67654,#67655,#67656,#67657,#67658),(#67659,#67660,
#67661,#67662,#67663,#67664),(#67665,#67666,#67667,#67668,#67669,#67670),
(#67671,#67672,#67673,#67674,#67675,#67676),(#67677,#67678,#67679,#67680,
#67681,#67682),(#67683,#67684,#67685,#67686,#67687,#67688),(#67689,#67690,
#67691,#67692,#67693,#67694),(#67695,#67696,#67697,#67698,#67699,#67700),
(#67701,#67702,#67703,#67704,#67705,#67706),(#67707,#67708,#67709,#67710,
#67711,#67712),(#67713,#67714,#67715,#67716,#67717,#67718),(#67719,#67720,
#67721,#67722,#67723,#67724),(#67725,#67726,#67727,#67728,#67729,#67730),
(#67731,#67732,#67733,#67734,#67735,#67736),(#67737,#67738,#67739,#67740,
#67741,#67742),(#67743,#67744,#67745,#67746,#67747,#67748),(#67749,#67750,
#67751,#67752,#67753,#67754)),.UNSPECIFIED.,.F.,.F.,.F.,(6,3,3,3,3,6),(6,
6),(16.6199171729,22.5384104949,30.5763255063,36.3852905632,40.8836098595,
50.0065304478),(0.,0.3),.UNSPECIFIED.);
#1028=B_SPLINE_SURFACE_WITH_KNOTS('',5,1,((#67775,#67776),(#67777,#67778),
(#67779,#67780),(#67781,#67782),(#67783,#67784),(#67785,#67786),(#67787,
#67788),(#67789,#67790),(#67791,#67792),(#67793,#67794),(#67795,#67796),
(#67797,#67798),(#67799,#67800),(#67801,#67802),(#67803,#67804),(#67805,
#67806),(#67807,#67808),(#67809,#67810),(#67811,#67812),(#67813,#67814),
(#67815,#67816),(#67817,#67818),(#67819,#67820),(#67821,#67822)),
 .UNSPECIFIED.,.F.,.F.,.F.,(6,3,3,3,3,3,3,6),(2,2),(5.81590786279,8.33607651362,
10.1951986769,12.0532651712,14.9345717632,19.4956760771,21.7667109588,28.5950255496),
(0.,0.168000000000001),.UNSPECIFIED.);
#1029=B_SPLINE_SURFACE_WITH_KNOTS('',5,5,((#67824,#67825,#67826,#67827,
#67828,#67829),(#67830,#67831,#67832,#67833,#67834,#67835),(#67836,#67837,
#67838,#67839,#67840,#67841),(#67842,#67843,#67844,#67845,#67846,#67847),
(#67848,#67849,#67850,#67851,#67852,#67853),(#67854,#67855,#67856,#67857,
#67858,#67859),(#67860,#67861,#67862,#67863,#67864,#67865),(#67866,#67867,
#67868,#67869,#67870,#67871),(#67872,#67873,#67874,#67875,#67876,#67877)),
 .UNSPECIFIED.,.F.,.F.,.F.,(6,3,6),(6,6),(0.168109267782,0.193813333781,
0.219517399779),(0.,0.3),.UNSPECIFIED.);
#1030=B_SPLINE_SURFACE_WITH_KNOTS('',5,5,((#67881,#67882,#67883,#67884,
#67885,#67886),(#67887,#67888,#67889,#67890,#67891,#67892),(#67893,#67894,
#67895,#67896,#67897,#67898),(#67899,#67900,#67901,#67902,#67903,#67904),
(#67905,#67906,#67907,#67908,#67909,#67910),(#67911,#67912,#67913,#67914,
#67915,#67916)),.UNSPECIFIED.,.F.,.F.,.F.,(6,6),(6,6),(0.167763693388,0.219167536337),
(0.,0.3),.UNSPECIFIED.);
#1031=B_SPLINE_SURFACE_WITH_KNOTS('',5,5,((#67922,#67923,#67924,#67925,
#67926,#67927),(#67928,#67929,#67930,#67931,#67932,#67933),(#67934,#67935,
#67936,#67937,#67938,#67939),(#67940,#67941,#67942,#67943,#67944,#67945),
(#67946,#67947,#67948,#67949,#67950,#67951),(#67952,#67953,#67954,#67955,
#67956,#67957),(#67958,#67959,#67960,#67961,#67962,#67963),(#67964,#67965,
#67966,#67967,#67968,#67969),(#67970,#67971,#67972,#67973,#67974,#67975)),
 .UNSPECIFIED.,.F.,.F.,.F.,(6,3,6),(6,6),(1.62532205434,2.95680207855,4.76574024567),
(0.,0.3),.UNSPECIFIED.);
#1032=B_SPLINE_SURFACE_WITH_KNOTS('',5,5,((#68014,#68015,#68016,#68017,
#68018,#68019),(#68020,#68021,#68022,#68023,#68024,#68025),(#68026,#68027,
#68028,#68029,#68030,#68031),(#68032,#68033,#68034,#68035,#68036,#68037),
(#68038,#68039,#68040,#68041,#68042,#68043),(#68044,#68045,#68046,#68047,
#68048,#68049),(#68050,#68051,#68052,#68053,#68054,#68055),(#68056,#68057,
#68058,#68059,#68060,#68061),(#68062,#68063,#68064,#68065,#68066,#68067)),
 .UNSPECIFIED.,.F.,.F.,.F.,(6,3,6),(6,6),(1.62047643556,3.23201205664,4.75541642643),
(0.,0.3),.UNSPECIFIED.);
#1033=B_SPLINE_SURFACE_WITH_KNOTS('',5,1,((#68106,#68107),(#68108,#68109),
(#68110,#68111),(#68112,#68113),(#68114,#68115),(#68116,#68117)),
 .UNSPECIFIED.,.F.,.F.,.F.,(6,6),(2,2),(1.41662542015,3.44037602036),(0.,
0.168000000000001),.UNSPECIFIED.);
#1034=B_SPLINE_SURFACE_WITH_KNOTS('',5,5,((#68129,#68130,#68131,#68132,
#68133,#68134),(#68135,#68136,#68137,#68138,#68139,#68140),(#68141,#68142,
#68143,#68144,#68145,#68146),(#68147,#68148,#68149,#68150,#68151,#68152),
(#68153,#68154,#68155,#68156,#68157,#68158),(#68159,#68160,#68161,#68162,
#68163,#68164),(#68165,#68166,#68167,#68168,#68169,#68170),(#68171,#68172,
#68173,#68174,#68175,#68176),(#68177,#68178,#68179,#68180,#68181,#68182)),
 .UNSPECIFIED.,.F.,.F.,.F.,(6,3,6),(6,6),(0.591274134056,1.32390942548,
1.88642149695),(0.,0.3),.UNSPECIFIED.);
#1035=B_SPLINE_SURFACE_WITH_KNOTS('',5,5,((#68191,#68192,#68193,#68194,
#68195,#68196),(#68197,#68198,#68199,#68200,#68201,#68202),(#68203,#68204,
#68205,#68206,#68207,#68208),(#68209,#68210,#68211,#68212,#68213,#68214),
(#68215,#68216,#68217,#68218,#68219,#68220),(#68221,#68222,#68223,#68224,
#68225,#68226),(#68227,#68228,#68229,#68230,#68231,#68232),(#68233,#68234,
#68235,#68236,#68237,#68238),(#68239,#68240,#68241,#68242,#68243,#68244)),
 .UNSPECIFIED.,.F.,.F.,.F.,(6,3,6),(6,6),(0.591155709264,1.24895127143,
1.8860355782),(0.,0.3),.UNSPECIFIED.);
#1036=B_SPLINE_SURFACE_WITH_KNOTS('',5,1,((#68256,#68257),(#68258,#68259),
(#68260,#68261),(#68262,#68263),(#68264,#68265),(#68266,#68267)),
 .UNSPECIFIED.,.F.,.F.,.F.,(6,6),(2,2),(0.493788369863,1.19920032681),(0.,
0.168000000000001),.UNSPECIFIED.);
#1037=B_SPLINE_SURFACE_WITH_KNOTS('',5,5,((#68269,#68270,#68271,#68272,
#68273,#68274),(#68275,#68276,#68277,#68278,#68279,#68280),(#68281,#68282,
#68283,#68284,#68285,#68286),(#68287,#68288,#68289,#68290,#68291,#68292),
(#68293,#68294,#68295,#68296,#68297,#68298),(#68299,#68300,#68301,#68302,
#68303,#68304),(#68305,#68306,#68307,#68308,#68309,#68310),(#68311,#68312,
#68313,#68314,#68315,#68316),(#68317,#68318,#68319,#68320,#68321,#68322)),
 .UNSPECIFIED.,.F.,.F.,.F.,(6,3,6),(6,6),(1.35769229991,2.30681875985,3.25594521979),
(0.,0.3),.UNSPECIFIED.);
#1038=B_SPLINE_SURFACE_WITH_KNOTS('',5,5,((#68326,#68327,#68328,#68329,
#68330,#68331),(#68332,#68333,#68334,#68335,#68336,#68337),(#68338,#68339,
#68340,#68341,#68342,#68343),(#68344,#68345,#68346,#68347,#68348,#68349),
(#68350,#68351,#68352,#68353,#68354,#68355),(#68356,#68357,#68358,#68359,
#68360,#68361),(#68362,#68363,#68364,#68365,#68366,#68367),(#68368,#68369,
#68370,#68371,#68372,#68373),(#68374,#68375,#68376,#68377,#68378,#68379)),
 .UNSPECIFIED.,.F.,.F.,.F.,(6,3,6),(6,6),(1.35799881012,2.30712712606,3.25625544201),
(0.,0.3),.UNSPECIFIED.);
#1039=B_SPLINE_SURFACE_WITH_KNOTS('',5,1,((#68383,#68384),(#68385,#68386),
(#68387,#68388),(#68389,#68390),(#68391,#68392),(#68393,#68394)),
 .UNSPECIFIED.,.F.,.F.,.F.,(6,6),(2,2),(0.96552770951,2.34485300881),(0.,
0.168000000000001),.UNSPECIFIED.);
#1040=B_SPLINE_SURFACE_WITH_KNOTS('',5,5,((#68396,#68397,#68398,#68399,
#68400,#68401),(#68402,#68403,#68404,#68405,#68406,#68407),(#68408,#68409,
#68410,#68411,#68412,#68413),(#68414,#68415,#68416,#68417,#68418,#68419),
(#68420,#68421,#68422,#68423,#68424,#68425),(#68426,#68427,#68428,#68429,
#68430,#68431),(#68432,#68433,#68434,#68435,#68436,#68437),(#68438,#68439,
#68440,#68441,#68442,#68443),(#68444,#68445,#68446,#68447,#68448,#68449),
(#68450,#68451,#68452,#68453,#68454,#68455),(#68456,#68457,#68458,#68459,
#68460,#68461),(#68462,#68463,#68464,#68465,#68466,#68467),(#68468,#68469,
#68470,#68471,#68472,#68473),(#68474,#68475,#68476,#68477,#68478,#68479),
(#68480,#68481,#68482,#68483,#68484,#68485),(#68486,#68487,#68488,#68489,
#68490,#68491),(#68492,#68493,#68494,#68495,#68496,#68497),(#68498,#68499,
#68500,#68501,#68502,#68503),(#68504,#68505,#68506,#68507,#68508,#68509),
(#68510,#68511,#68512,#68513,#68514,#68515),(#68516,#68517,#68518,#68519,
#68520,#68521)),.UNSPECIFIED.,.F.,.F.,.F.,(6,3,3,3,3,3,6),(6,6),(4.50366397293,
11.9396101613,13.7854271296,14.9414943029,15.6351526747,16.3253424406,17.7760995894),
(0.,0.3),.UNSPECIFIED.);
#1041=B_SPLINE_SURFACE_WITH_KNOTS('',5,5,((#68540,#68541,#68542,#68543,
#68544,#68545),(#68546,#68547,#68548,#68549,#68550,#68551),(#68552,#68553,
#68554,#68555,#68556,#68557),(#68558,#68559,#68560,#68561,#68562,#68563),
(#68564,#68565,#68566,#68567,#68568,#68569),(#68570,#68571,#68572,#68573,
#68574,#68575),(#68576,#68577,#68578,#68579,#68580,#68581),(#68582,#68583,
#68584,#68585,#68586,#68587),(#68588,#68589,#68590,#68591,#68592,#68593),
(#68594,#68595,#68596,#68597,#68598,#68599),(#68600,#68601,#68602,#68603,
#68604,#68605),(#68606,#68607,#68608,#68609,#68610,#68611),(#68612,#68613,
#68614,#68615,#68616,#68617),(#68618,#68619,#68620,#68621,#68622,#68623),
(#68624,#68625,#68626,#68627,#68628,#68629),(#68630,#68631,#68632,#68633,
#68634,#68635),(#68636,#68637,#68638,#68639,#68640,#68641),(#68642,#68643,
#68644,#68645,#68646,#68647),(#68648,#68649,#68650,#68651,#68652,#68653),
(#68654,#68655,#68656,#68657,#68658,#68659),(#68660,#68661,#68662,#68663,
#68664,#68665)),.UNSPECIFIED.,.F.,.F.,.F.,(6,3,3,3,3,3,6),(6,6),(4.57396017214,
5.92885717573,7.41888220249,8.65504128479,9.89120036709,11.8754981945,17.8472140382),
(0.,0.3),.UNSPECIFIED.);
#1042=B_SPLINE_SURFACE_WITH_KNOTS('',5,1,((#68687,#68688),(#68689,#68690),
(#68691,#68692),(#68693,#68694),(#68695,#68696),(#68697,#68698),(#68699,
#68700),(#68701,#68702),(#68703,#68704),(#68705,#68706),(#68707,#68708),
(#68709,#68710),(#68711,#68712),(#68713,#68714),(#68715,#68716),(#68717,
#68718),(#68719,#68720),(#68721,#68722)),.UNSPECIFIED.,.F.,.F.,.F.,(6,3,
3,3,3,6),(2,2),(2.29196781189,3.18681436572,5.94671679294,9.63664271035,
10.6008983863,11.5146904868),(0.,0.168000000000001),.UNSPECIFIED.);
#1043=B_SPLINE_SURFACE_WITH_KNOTS('',5,5,((#68723,#68724,#68725,#68726,
#68727,#68728),(#68729,#68730,#68731,#68732,#68733,#68734),(#68735,#68736,
#68737,#68738,#68739,#68740),(#68741,#68742,#68743,#68744,#68745,#68746),
(#68747,#68748,#68749,#68750,#68751,#68752),(#68753,#68754,#68755,#68756,
#68757,#68758),(#68759,#68760,#68761,#68762,#68763,#68764),(#68765,#68766,
#68767,#68768,#68769,#68770),(#68771,#68772,#68773,#68774,#68775,#68776),
(#68777,#68778,#68779,#68780,#68781,#68782),(#68783,#68784,#68785,#68786,
#68787,#68788),(#68789,#68790,#68791,#68792,#68793,#68794)),
 .UNSPECIFIED.,.F.,.F.,.F.,(6,3,3,6),(6,6),(3.96957835788,8.52280966994,
10.8013830785,13.2112648606),(0.,0.3),.UNSPECIFIED.);
#1044=B_SPLINE_SURFACE_WITH_KNOTS('',5,5,((#68811,#68812,#68813,#68814,
#68815,#68816),(#68817,#68818,#68819,#68820,#68821,#68822),(#68823,#68824,
#68825,#68826,#68827,#68828),(#68829,#68830,#68831,#68832,#68833,#68834),
(#68835,#68836,#68837,#68838,#68839,#68840),(#68841,#68842,#68843,#68844,
#68845,#68846),(#68847,#68848,#68849,#68850,#68851,#68852),(#68853,#68854,
#68855,#68856,#68857,#68858),(#68859,#68860,#68861,#68862,#68863,#68864),
(#68865,#68866,#68867,#68868,#68869,#68870),(#68871,#68872,#68873,#68874,
#68875,#68876),(#68877,#68878,#68879,#68880,#68881,#68882)),
 .UNSPECIFIED.,.F.,.F.,.F.,(6,3,3,6),(6,6),(3.98723768815,6.53884477084,
8.77115009928,13.2289036984),(0.,0.3),.UNSPECIFIED.);
#1045=B_SPLINE_SURFACE_WITH_KNOTS('',5,1,((#68908,#68909),(#68910,#68911),
(#68912,#68913),(#68914,#68915),(#68916,#68917),(#68918,#68919),(#68920,
#68921),(#68922,#68923),(#68924,#68925),(#68926,#68927),(#68928,#68929),
(#68930,#68931),(#68932,#68933),(#68934,#68935),(#68936,#68937),(#68938,
#68939),(#68940,#68941),(#68942,#68943),(#68944,#68945),(#68946,#68947),
(#68948,#68949)),.UNSPECIFIED.,.F.,.F.,.F.,(6,3,3,3,3,3,6),(2,2),(1.95811472427,
3.23566574513,3.88589710876,5.21424414623,6.55599923652,7.22663415565,8.5548107935),
(0.,0.168000000000001),.UNSPECIFIED.);
#1046=B_SPLINE_SURFACE_WITH_KNOTS('',5,5,((#68952,#68953,#68954,#68955,
#68956,#68957),(#68958,#68959,#68960,#68961,#68962,#68963),(#68964,#68965,
#68966,#68967,#68968,#68969),(#68970,#68971,#68972,#68973,#68974,#68975),
(#68976,#68977,#68978,#68979,#68980,#68981),(#68982,#68983,#68984,#68985,
#68986,#68987),(#68988,#68989,#68990,#68991,#68992,#68993),(#68994,#68995,
#68996,#68997,#68998,#68999),(#69000,#69001,#69002,#69003,#69004,#69005)),
 .UNSPECIFIED.,.F.,.F.,.F.,(6,3,6),(6,6),(0.620886007027,1.29421436741,
2.17771162296),(0.,0.3),.UNSPECIFIED.);
#1047=B_SPLINE_SURFACE_WITH_KNOTS('',5,5,((#69014,#69015,#69016,#69017,
#69018,#69019),(#69020,#69021,#69022,#69023,#69024,#69025),(#69026,#69027,
#69028,#69029,#69030,#69031),(#69032,#69033,#69034,#69035,#69036,#69037),
(#69038,#69039,#69040,#69041,#69042,#69043),(#69044,#69045,#69046,#69047,
#69048,#69049),(#69050,#69051,#69052,#69053,#69054,#69055),(#69056,#69057,
#69058,#69059,#69060,#69061),(#69062,#69063,#69064,#69065,#69066,#69067)),
 .UNSPECIFIED.,.F.,.F.,.F.,(6,3,6),(6,6),(0.620875478398,1.40616268126,
2.17764450768),(0.,0.3),.UNSPECIFIED.);
#1048=B_SPLINE_SURFACE_WITH_KNOTS('',5,1,((#69113,#69114),(#69115,#69116),
(#69117,#69118),(#69119,#69120),(#69121,#69122),(#69123,#69124)),
 .UNSPECIFIED.,.F.,.F.,.F.,(6,6),(2,2),(0.52702168644,1.27990980993),(0.,
0.168000000000001),.UNSPECIFIED.);
#1049=B_SPLINE_SURFACE_WITH_KNOTS('',5,5,((#69126,#69127,#69128,#69129,
#69130,#69131),(#69132,#69133,#69134,#69135,#69136,#69137),(#69138,#69139,
#69140,#69141,#69142,#69143),(#69144,#69145,#69146,#69147,#69148,#69149),
(#69150,#69151,#69152,#69153,#69154,#69155),(#69156,#69157,#69158,#69159,
#69160,#69161),(#69162,#69163,#69164,#69165,#69166,#69167),(#69168,#69169,
#69170,#69171,#69172,#69173),(#69174,#69175,#69176,#69177,#69178,#69179)),
 .UNSPECIFIED.,.F.,.F.,.F.,(6,3,6),(6,6),(8.8689446919,17.3139944292,23.7989023215),
(0.,0.3),.UNSPECIFIED.);
#1050=B_SPLINE_SURFACE_WITH_KNOTS('',5,5,((#69191,#69192,#69193,#69194,
#69195,#69196),(#69197,#69198,#69199,#69200,#69201,#69202),(#69203,#69204,
#69205,#69206,#69207,#69208),(#69209,#69210,#69211,#69212,#69213,#69214),
(#69215,#69216,#69217,#69218,#69219,#69220),(#69221,#69222,#69223,#69224,
#69225,#69226),(#69227,#69228,#69229,#69230,#69231,#69232),(#69233,#69234,
#69235,#69236,#69237,#69238),(#69239,#69240,#69241,#69242,#69243,#69244)),
 .UNSPECIFIED.,.F.,.F.,.F.,(6,3,6),(6,6),(8.86843301073,15.565351162,23.7990765439),
(0.,0.3),.UNSPECIFIED.);
#1051=B_SPLINE_SURFACE_WITH_KNOTS('',5,1,((#69253,#69254),(#69255,#69256),
(#69257,#69258),(#69259,#69260),(#69261,#69262),(#69263,#69264)),
 .UNSPECIFIED.,.F.,.F.,.F.,(6,6),(2,2),(7.91037074022,19.2109003691),(0.,
0.168000000000001),.UNSPECIFIED.);
#1052=B_SPLINE_SURFACE_WITH_KNOTS('',5,5,((#69266,#69267,#69268,#69269,
#69270,#69271),(#69272,#69273,#69274,#69275,#69276,#69277),(#69278,#69279,
#69280,#69281,#69282,#69283),(#69284,#69285,#69286,#69287,#69288,#69289),
(#69290,#69291,#69292,#69293,#69294,#69295),(#69296,#69297,#69298,#69299,
#69300,#69301),(#69302,#69303,#69304,#69305,#69306,#69307),(#69308,#69309,
#69310,#69311,#69312,#69313),(#69314,#69315,#69316,#69317,#69318,#69319)),
 .UNSPECIFIED.,.F.,.F.,.F.,(6,3,6),(6,6),(8.86873667877,17.3137864161,23.7986943084),
(0.,0.3),.UNSPECIFIED.);
#1053=B_SPLINE_SURFACE_WITH_KNOTS('',5,5,((#69331,#69332,#69333,#69334,
#69335,#69336),(#69337,#69338,#69339,#69340,#69341,#69342),(#69343,#69344,
#69345,#69346,#69347,#69348),(#69349,#69350,#69351,#69352,#69353,#69354),
(#69355,#69356,#69357,#69358,#69359,#69360),(#69361,#69362,#69363,#69364,
#69365,#69366),(#69367,#69368,#69369,#69370,#69371,#69372),(#69373,#69374,
#69375,#69376,#69377,#69378),(#69379,#69380,#69381,#69382,#69383,#69384)),
 .UNSPECIFIED.,.F.,.F.,.F.,(6,3,6),(6,6),(8.86829015303,15.5652083044,23.7989336863),
(0.,0.3),.UNSPECIFIED.);
#1054=B_SPLINE_SURFACE_WITH_KNOTS('',5,1,((#69393,#69394),(#69395,#69396),
(#69397,#69398),(#69399,#69400),(#69401,#69402),(#69403,#69404)),
 .UNSPECIFIED.,.F.,.F.,.F.,(6,6),(2,2),(7.91037074022,19.2109003691),(0.,
0.168000000000001),.UNSPECIFIED.);
#1055=B_SPLINE_SURFACE_WITH_KNOTS('',5,5,((#69406,#69407,#69408,#69409,
#69410,#69411),(#69412,#69413,#69414,#69415,#69416,#69417),(#69418,#69419,
#69420,#69421,#69422,#69423),(#69424,#69425,#69426,#69427,#69428,#69429),
(#69430,#69431,#69432,#69433,#69434,#69435),(#69436,#69437,#69438,#69439,
#69440,#69441),(#69442,#69443,#69444,#69445,#69446,#69447),(#69448,#69449,
#69450,#69451,#69452,#69453),(#69454,#69455,#69456,#69457,#69458,#69459)),
 .UNSPECIFIED.,.F.,.F.,.F.,(6,3,6),(6,6),(0.620884089829,1.29421245021,
2.17770970576),(0.,0.3),.UNSPECIFIED.);
#1056=B_SPLINE_SURFACE_WITH_KNOTS('',5,5,((#69468,#69469,#69470,#69471,
#69472,#69473),(#69474,#69475,#69476,#69477,#69478,#69479),(#69480,#69481,
#69482,#69483,#69484,#69485),(#69486,#69487,#69488,#69489,#69490,#69491),
(#69492,#69493,#69494,#69495,#69496,#69497),(#69498,#69499,#69500,#69501,
#69502,#69503),(#69504,#69505,#69506,#69507,#69508,#69509),(#69510,#69511,
#69512,#69513,#69514,#69515),(#69516,#69517,#69518,#69519,#69520,#69521)),
 .UNSPECIFIED.,.F.,.F.,.F.,(6,3,6),(6,6),(0.620866600281,1.40615380315,
2.1776356295),(0.,0.3),.UNSPECIFIED.);
#1057=B_SPLINE_SURFACE_WITH_KNOTS('',5,1,((#69567,#69568),(#69569,#69570),
(#69571,#69572),(#69573,#69574),(#69575,#69576),(#69577,#69578)),
 .UNSPECIFIED.,.F.,.F.,.F.,(6,6),(2,2),(0.52702168644,1.27990980993),(0.,
0.168000000000001),.UNSPECIFIED.);
#1058=B_SPLINE_SURFACE_WITH_KNOTS('',5,5,((#69580,#69581,#69582,#69583,
#69584,#69585),(#69586,#69587,#69588,#69589,#69590,#69591),(#69592,#69593,
#69594,#69595,#69596,#69597),(#69598,#69599,#69600,#69601,#69602,#69603),
(#69604,#69605,#69606,#69607,#69608,#69609),(#69610,#69611,#69612,#69613,
#69614,#69615),(#69616,#69617,#69618,#69619,#69620,#69621),(#69622,#69623,
#69624,#69625,#69626,#69627),(#69628,#69629,#69630,#69631,#69632,#69633),
(#69634,#69635,#69636,#69637,#69638,#69639),(#69640,#69641,#69642,#69643,
#69644,#69645),(#69646,#69647,#69648,#69649,#69650,#69651)),
 .UNSPECIFIED.,.F.,.F.,.F.,(6,3,3,6),(6,6),(3.98757792105,6.5613910649,
8.51083290938,13.2292989355),(0.,0.3),.UNSPECIFIED.);
#1059=B_SPLINE_SURFACE_WITH_KNOTS('',5,5,((#69675,#69676,#69677,#69678,
#69679,#69680),(#69681,#69682,#69683,#69684,#69685,#69686),(#69687,#69688,
#69689,#69690,#69691,#69692),(#69693,#69694,#69695,#69696,#69697,#69698),
(#69699,#69700,#69701,#69702,#69703,#69704),(#69705,#69706,#69707,#69708,
#69709,#69710),(#69711,#69712,#69713,#69714,#69715,#69716),(#69717,#69718,
#69719,#69720,#69721,#69722),(#69723,#69724,#69725,#69726,#69727,#69728),
(#69729,#69730,#69731,#69732,#69733,#69734),(#69735,#69736,#69737,#69738,
#69739,#69740),(#69741,#69742,#69743,#69744,#69745,#69746)),
 .UNSPECIFIED.,.F.,.F.,.F.,(6,3,3,6),(6,6),(3.96959709723,8.41545051994,
10.641451928,13.2113291298),(0.,0.3),.UNSPECIFIED.);
#1060=B_SPLINE_SURFACE_WITH_KNOTS('',5,1,((#69770,#69771),(#69772,#69773),
(#69774,#69775),(#69776,#69777),(#69778,#69779),(#69780,#69781),(#69782,
#69783),(#69784,#69785),(#69786,#69787),(#69788,#69789),(#69790,#69791),
(#69792,#69793),(#69794,#69795),(#69796,#69797),(#69798,#69799),(#69800,
#69801),(#69802,#69803),(#69804,#69805),(#69806,#69807),(#69808,#69809),
(#69810,#69811)),.UNSPECIFIED.,.F.,.F.,.F.,(6,3,3,3,3,3,6),(2,2),(1.98342753277,
3.31160417062,3.98223908975,5.32399418003,6.6523412175,7.30257258114,8.58012360199),
(0.,0.168000000000001),.UNSPECIFIED.);
#1061=B_SPLINE_SURFACE_WITH_KNOTS('',5,5,((#69813,#69814,#69815,#69816,
#69817,#69818),(#69819,#69820,#69821,#69822,#69823,#69824),(#69825,#69826,
#69827,#69828,#69829,#69830),(#69831,#69832,#69833,#69834,#69835,#69836),
(#69837,#69838,#69839,#69840,#69841,#69842),(#69843,#69844,#69845,#69846,
#69847,#69848),(#69849,#69850,#69851,#69852,#69853,#69854),(#69855,#69856,
#69857,#69858,#69859,#69860),(#69861,#69862,#69863,#69864,#69865,#69866),
(#69867,#69868,#69869,#69870,#69871,#69872),(#69873,#69874,#69875,#69876,
#69877,#69878),(#69879,#69880,#69881,#69882,#69883,#69884),(#69885,#69886,
#69887,#69888,#69889,#69890),(#69891,#69892,#69893,#69894,#69895,#69896),
(#69897,#69898,#69899,#69900,#69901,#69902)),.UNSPECIFIED.,.F.,.F.,.F.,
(6,3,3,3,6),(6,6),(1.97579103232,2.74141165766,3.51110670868,5.05016737922,
7.48619339243),(0.,0.3),.UNSPECIFIED.);
#1062=B_SPLINE_SURFACE_WITH_KNOTS('',5,5,((#69920,#69921,#69922,#69923,
#69924,#69925),(#69926,#69927,#69928,#69929,#69930,#69931),(#69932,#69933,
#69934,#69935,#69936,#69937),(#69938,#69939,#69940,#69941,#69942,#69943),
(#69944,#69945,#69946,#69947,#69948,#69949),(#69950,#69951,#69952,#69953,
#69954,#69955),(#69956,#69957,#69958,#69959,#69960,#69961),(#69962,#69963,
#69964,#69965,#69966,#69967),(#69968,#69969,#69970,#69971,#69972,#69973),
(#69974,#69975,#69976,#69977,#69978,#69979),(#69980,#69981,#69982,#69983,
#69984,#69985),(#69986,#69987,#69988,#69989,#69990,#69991),(#69992,#69993,
#69994,#69995,#69996,#69997),(#69998,#69999,#70000,#70001,#70002,#70003),
(#70004,#70005,#70006,#70007,#70008,#70009)),.UNSPECIFIED.,.F.,.F.,.F.,
(6,3,3,3,6),(6,6),(2.79838908821,5.60075527683,6.50571033408,7.18248685409,
8.30480917216),(0.,0.3),.UNSPECIFIED.);
#1063=B_SPLINE_SURFACE_WITH_KNOTS('',5,1,((#70103,#70104),(#70105,#70106),
(#70107,#70108),(#70109,#70110),(#70111,#70112),(#70113,#70114),(#70115,
#70116),(#70117,#70118),(#70119,#70120),(#70121,#70122),(#70123,#70124),
(#70125,#70126),(#70127,#70128),(#70129,#70130),(#70131,#70132)),
 .UNSPECIFIED.,.F.,.F.,.F.,(6,3,3,3,6),(2,2),(1.35736905211,2.5282953222,
3.70557211292,4.48067762876,5.21689863741),(0.,0.168000000000001),
 .UNSPECIFIED.);
#1064=B_SPLINE_SURFACE_WITH_KNOTS('',5,5,((#70134,#70135,#70136,#70137,
#70138,#70139),(#70140,#70141,#70142,#70143,#70144,#70145),(#70146,#70147,
#70148,#70149,#70150,#70151),(#70152,#70153,#70154,#70155,#70156,#70157),
(#70158,#70159,#70160,#70161,#70162,#70163),(#70164,#70165,#70166,#70167,
#70168,#70169),(#70170,#70171,#70172,#70173,#70174,#70175),(#70176,#70177,
#70178,#70179,#70180,#70181),(#70182,#70183,#70184,#70185,#70186,#70187),
(#70188,#70189,#70190,#70191,#70192,#70193),(#70194,#70195,#70196,#70197,
#70198,#70199),(#70200,#70201,#70202,#70203,#70204,#70205),(#70206,#70207,
#70208,#70209,#70210,#70211),(#70212,#70213,#70214,#70215,#70216,#70217),
(#70218,#70219,#70220,#70221,#70222,#70223),(#70224,#70225,#70226,#70227,
#70228,#70229),(#70230,#70231,#70232,#70233,#70234,#70235),(#70236,#70237,
#70238,#70239,#70240,#70241),(#70242,#70243,#70244,#70245,#70246,#70247),
(#70248,#70249,#70250,#70251,#70252,#70253),(#70254,#70255,#70256,#70257,
#70258,#70259),(#70260,#70261,#70262,#70263,#70264,#70265),(#70266,#70267,
#70268,#70269,#70270,#70271),(#70272,#70273,#70274,#70275,#70276,#70277),
(#70278,#70279,#70280,#70281,#70282,#70283),(#70284,#70285,#70286,#70287,
#70288,#70289),(#70290,#70291,#70292,#70293,#70294,#70295),(#70296,#70297,
#70298,#70299,#70300,#70301),(#70302,#70303,#70304,#70305,#70306,#70307),
(#70308,#70309,#70310,#70311,#70312,#70313)),.UNSPECIFIED.,.F.,.F.,.F.,
(6,3,3,3,3,3,3,3,3,6),(6,6),(13.0484209298,14.3771824271,15.7058202332,
19.4329797586,22.2257607493,27.8279202183,33.4574539385,41.6679674559,47.6452295392,
53.2420797137),(0.,0.3),.UNSPECIFIED.);
#1065=B_SPLINE_SURFACE_WITH_KNOTS('',5,5,((#70355,#70356,#70357,#70358,
#70359,#70360),(#70361,#70362,#70363,#70364,#70365,#70366),(#70367,#70368,
#70369,#70370,#70371,#70372),(#70373,#70374,#70375,#70376,#70377,#70378),
(#70379,#70380,#70381,#70382,#70383,#70384),(#70385,#70386,#70387,#70388,
#70389,#70390),(#70391,#70392,#70393,#70394,#70395,#70396),(#70397,#70398,
#70399,#70400,#70401,#70402),(#70403,#70404,#70405,#70406,#70407,#70408),
(#70409,#70410,#70411,#70412,#70413,#70414),(#70415,#70416,#70417,#70418,
#70419,#70420),(#70421,#70422,#70423,#70424,#70425,#70426),(#70427,#70428,
#70429,#70430,#70431,#70432),(#70433,#70434,#70435,#70436,#70437,#70438),
(#70439,#70440,#70441,#70442,#70443,#70444),(#70445,#70446,#70447,#70448,
#70449,#70450),(#70451,#70452,#70453,#70454,#70455,#70456),(#70457,#70458,
#70459,#70460,#70461,#70462),(#70463,#70464,#70465,#70466,#70467,#70468),
(#70469,#70470,#70471,#70472,#70473,#70474),(#70475,#70476,#70477,#70478,
#70479,#70480),(#70481,#70482,#70483,#70484,#70485,#70486),(#70487,#70488,
#70489,#70490,#70491,#70492),(#70493,#70494,#70495,#70496,#70497,#70498),
(#70499,#70500,#70501,#70502,#70503,#70504),(#70505,#70506,#70507,#70508,
#70509,#70510),(#70511,#70512,#70513,#70514,#70515,#70516),(#70517,#70518,
#70519,#70520,#70521,#70522),(#70523,#70524,#70525,#70526,#70527,#70528),
(#70529,#70530,#70531,#70532,#70533,#70534)),.UNSPECIFIED.,.F.,.F.,.F.,
(6,3,3,3,3,3,3,3,3,6),(6,6),(13.30850513,22.9473682995,26.1445609307,32.8906058289,
38.6549810462,44.3241190945,47.1169000853,50.8440596107,52.1726974168,53.5008998895),
(0.,0.3),.UNSPECIFIED.);
#1066=B_SPLINE_SURFACE_WITH_KNOTS('',5,1,((#70576,#70577),(#70578,#70579),
(#70580,#70581),(#70582,#70583),(#70584,#70585),(#70586,#70587),(#70588,
#70589),(#70590,#70591),(#70592,#70593),(#70594,#70595),(#70596,#70597),
(#70598,#70599),(#70600,#70601),(#70602,#70603),(#70604,#70605),(#70606,
#70607),(#70608,#70609),(#70610,#70611),(#70612,#70613),(#70614,#70615),
(#70616,#70617),(#70618,#70619),(#70620,#70621),(#70622,#70623),(#70624,
#70625),(#70626,#70627),(#70628,#70629),(#70630,#70631),(#70632,#70633),
(#70634,#70635),(#70636,#70637),(#70638,#70639),(#70640,#70641),(#70642,
#70643),(#70644,#70645),(#70646,#70647),(#70648,#70649),(#70650,#70651),
(#70652,#70653)),.UNSPECIFIED.,.F.,.F.,.F.,(6,3,3,3,3,3,3,3,3,3,3,3,6),
(2,2),(5.58814360433,6.30725257391,8.49590865562,13.7853920845,17.0993514659,
21.0213468886,22.3238009285,24.9287160587,27.5338438134,29.43694187,30.0730233774,
30.7075742798,31.7310892021),(0.,0.168000000000001),.UNSPECIFIED.);
#1067=B_SPLINE_SURFACE_WITH_KNOTS('',5,5,((#70655,#70656,#70657,#70658,
#70659,#70660),(#70661,#70662,#70663,#70664,#70665,#70666),(#70667,#70668,
#70669,#70670,#70671,#70672),(#70673,#70674,#70675,#70676,#70677,#70678),
(#70679,#70680,#70681,#70682,#70683,#70684),(#70685,#70686,#70687,#70688,
#70689,#70690),(#70691,#70692,#70693,#70694,#70695,#70696),(#70697,#70698,
#70699,#70700,#70701,#70702),(#70703,#70704,#70705,#70706,#70707,#70708)),
 .UNSPECIFIED.,.F.,.F.,.F.,(6,3,6),(6,6),(2.27369288769,4.21221438122,6.15073587476),
(0.,0.3),.UNSPECIFIED.);
#1068=B_SPLINE_SURFACE_WITH_KNOTS('',5,5,((#70712,#70713,#70714,#70715,
#70716,#70717),(#70718,#70719,#70720,#70721,#70722,#70723),(#70724,#70725,
#70726,#70727,#70728,#70729),(#70730,#70731,#70732,#70733,#70734,#70735),
(#70736,#70737,#70738,#70739,#70740,#70741),(#70742,#70743,#70744,#70745,
#70746,#70747),(#70748,#70749,#70750,#70751,#70752,#70753),(#70754,#70755,
#70756,#70757,#70758,#70759),(#70760,#70761,#70762,#70763,#70764,#70765)),
 .UNSPECIFIED.,.F.,.F.,.F.,(6,3,6),(6,6),(2.27401419165,4.2125468931,6.15107959455),
(0.,0.3),.UNSPECIFIED.);
#1069=B_SPLINE_SURFACE_WITH_KNOTS('',5,1,((#70769,#70770),(#70771,#70772),
(#70773,#70774),(#70775,#70776),(#70777,#70778),(#70779,#70780)),
 .UNSPECIFIED.,.F.,.F.,.F.,(6,6),(2,2),(1.9503302649,4.73651635762),(0.,
0.168000000000001),.UNSPECIFIED.);
#1070=B_SPLINE_SURFACE_WITH_KNOTS('',5,5,((#70782,#70783,#70784,#70785,
#70786,#70787),(#70788,#70789,#70790,#70791,#70792,#70793),(#70794,#70795,
#70796,#70797,#70798,#70799),(#70800,#70801,#70802,#70803,#70804,#70805),
(#70806,#70807,#70808,#70809,#70810,#70811),(#70812,#70813,#70814,#70815,
#70816,#70817),(#70818,#70819,#70820,#70821,#70822,#70823),(#70824,#70825,
#70826,#70827,#70828,#70829),(#70830,#70831,#70832,#70833,#70834,#70835),
(#70836,#70837,#70838,#70839,#70840,#70841),(#70842,#70843,#70844,#70845,
#70846,#70847),(#70848,#70849,#70850,#70851,#70852,#70853),(#70854,#70855,
#70856,#70857,#70858,#70859),(#70860,#70861,#70862,#70863,#70864,#70865),
(#70866,#70867,#70868,#70869,#70870,#70871),(#70872,#70873,#70874,#70875,
#70876,#70877),(#70878,#70879,#70880,#70881,#70882,#70883),(#70884,#70885,
#70886,#70887,#70888,#70889),(#70890,#70891,#70892,#70893,#70894,#70895),
(#70896,#70897,#70898,#70899,#70900,#70901),(#70902,#70903,#70904,#70905,
#70906,#70907),(#70908,#70909,#70910,#70911,#70912,#70913),(#70914,#70915,
#70916,#70917,#70918,#70919),(#70920,#70921,#70922,#70923,#70924,#70925),
(#70926,#70927,#70928,#70929,#70930,#70931),(#70932,#70933,#70934,#70935,
#70936,#70937),(#70938,#70939,#70940,#70941,#70942,#70943),(#70944,#70945,
#70946,#70947,#70948,#70949),(#70950,#70951,#70952,#70953,#70954,#70955),
(#70956,#70957,#70958,#70959,#70960,#70961)),.UNSPECIFIED.,.F.,.F.,.F.,
(6,3,3,3,3,3,3,3,3,6),(6,6),(13.309352184,22.6115369711,27.6548280379,33.4130337529,
39.0575237739,44.6786014526,47.4881463874,50.2976913221,51.8585343078,53.4991626515),
(0.,0.3),.UNSPECIFIED.);
#1071=B_SPLINE_SURFACE_WITH_KNOTS('',5,5,((#71003,#71004,#71005,#71006,
#71007,#71008),(#71009,#71010,#71011,#71012,#71013,#71014),(#71015,#71016,
#71017,#71018,#71019,#71020),(#71021,#71022,#71023,#71024,#71025,#71026),
(#71027,#71028,#71029,#71030,#71031,#71032),(#71033,#71034,#71035,#71036,
#71037,#71038),(#71039,#71040,#71041,#71042,#71043,#71044),(#71045,#71046,
#71047,#71048,#71049,#71050),(#71051,#71052,#71053,#71054,#71055,#71056),
(#71057,#71058,#71059,#71060,#71061,#71062),(#71063,#71064,#71065,#71066,
#71067,#71068),(#71069,#71070,#71071,#71072,#71073,#71074),(#71075,#71076,
#71077,#71078,#71079,#71080),(#71081,#71082,#71083,#71084,#71085,#71086),
(#71087,#71088,#71089,#71090,#71091,#71092),(#71093,#71094,#71095,#71096,
#71097,#71098),(#71099,#71100,#71101,#71102,#71103,#71104),(#71105,#71106,
#71107,#71108,#71109,#71110),(#71111,#71112,#71113,#71114,#71115,#71116),
(#71117,#71118,#71119,#71120,#71121,#71122),(#71123,#71124,#71125,#71126,
#71127,#71128),(#71129,#71130,#71131,#71132,#71133,#71134),(#71135,#71136,
#71137,#71138,#71139,#71140),(#71141,#71142,#71143,#71144,#71145,#71146),
(#71147,#71148,#71149,#71150,#71151,#71152),(#71153,#71154,#71155,#71156,
#71157,#71158),(#71159,#71160,#71161,#71162,#71163,#71164)),
 .UNSPECIFIED.,.F.,.F.,.F.,(6,3,3,3,3,3,3,3,6),(6,6),(13.1529830415,14.6756170516,
15.9546703779,18.8316459182,24.5861173859,33.242662653,37.0047521746,43.9231881457,
53.3460404053),(0.,0.3),.UNSPECIFIED.);
#1072=B_SPLINE_SURFACE_WITH_KNOTS('',5,1,((#71372,#71373),(#71374,#71375),
(#71376,#71377),(#71378,#71379),(#71380,#71381),(#71382,#71383),(#71384,
#71385),(#71386,#71387),(#71388,#71389),(#71390,#71391),(#71392,#71393),
(#71394,#71395),(#71396,#71397),(#71398,#71399),(#71400,#71401),(#71402,
#71403),(#71404,#71405),(#71406,#71407),(#71408,#71409),(#71410,#71411),
(#71412,#71413),(#71414,#71415),(#71416,#71417),(#71418,#71419),(#71420,
#71421),(#71422,#71423),(#71424,#71425),(#71426,#71427),(#71428,#71429),
(#71430,#71431),(#71432,#71433),(#71434,#71435),(#71436,#71437),(#71438,
#71439),(#71440,#71441),(#71442,#71443),(#71444,#71445),(#71446,#71447),
(#71448,#71449)),.UNSPECIFIED.,.F.,.F.,.F.,(6,3,3,3,3,3,3,3,3,3,3,3,6),
(2,2),(5.7403465807,6.76386150304,7.39841240531,8.03449391269,9.9375919693,
12.5427197241,15.1476348542,16.4500888941,20.3720843168,23.6860436982,28.9755271271,
31.1641832088,31.8832921784),(0.,0.168000000000001),.UNSPECIFIED.);
#1073=B_SPLINE_SURFACE_WITH_KNOTS('',5,5,((#71451,#71452,#71453,#71454,
#71455,#71456),(#71457,#71458,#71459,#71460,#71461,#71462),(#71463,#71464,
#71465,#71466,#71467,#71468),(#71469,#71470,#71471,#71472,#71473,#71474),
(#71475,#71476,#71477,#71478,#71479,#71480),(#71481,#71482,#71483,#71484,
#71485,#71486),(#71487,#71488,#71489,#71490,#71491,#71492),(#71493,#71494,
#71495,#71496,#71497,#71498),(#71499,#71500,#71501,#71502,#71503,#71504),
(#71505,#71506,#71507,#71508,#71509,#71510),(#71511,#71512,#71513,#71514,
#71515,#71516),(#71517,#71518,#71519,#71520,#71521,#71522),(#71523,#71524,
#71525,#71526,#71527,#71528),(#71529,#71530,#71531,#71532,#71533,#71534),
(#71535,#71536,#71537,#71538,#71539,#71540)),.UNSPECIFIED.,.F.,.F.,.F.,
(6,3,3,3,6),(6,6),(2.79870510475,4.34415602331,5.89253492006,7.24045509522,
8.30631830913),(0.,0.3),.UNSPECIFIED.);
#1074=B_SPLINE_SURFACE_WITH_KNOTS('',5,5,((#71556,#71557,#71558,#71559,
#71560,#71561),(#71562,#71563,#71564,#71565,#71566,#71567),(#71568,#71569,
#71570,#71571,#71572,#71573),(#71574,#71575,#71576,#71577,#71578,#71579),
(#71580,#71581,#71582,#71583,#71584,#71585),(#71586,#71587,#71588,#71589,
#71590,#71591),(#71592,#71593,#71594,#71595,#71596,#71597),(#71598,#71599,
#71600,#71601,#71602,#71603),(#71604,#71605,#71606,#71607,#71608,#71609),
(#71610,#71611,#71612,#71613,#71614,#71615),(#71616,#71617,#71618,#71619,
#71620,#71621),(#71622,#71623,#71624,#71625,#71626,#71627)),
 .UNSPECIFIED.,.F.,.F.,.F.,(6,3,3,6),(6,6),(2.28525111063,3.36176031805,
5.06337143522,7.79281869645),(0.,0.3),.UNSPECIFIED.);
#1075=B_SPLINE_SURFACE_WITH_KNOTS('',5,1,((#71710,#71711),(#71712,#71713),
(#71714,#71715),(#71716,#71717),(#71718,#71719),(#71720,#71721),(#71722,
#71723),(#71724,#71725),(#71726,#71727),(#71728,#71729),(#71730,#71731),
(#71732,#71733),(#71734,#71735),(#71736,#71737),(#71738,#71739)),
 .UNSPECIFIED.,.F.,.F.,.F.,(6,3,3,3,6),(2,2),(1.14001641713,1.87623741919,
2.65134293549,3.82861972691,4.99954599766),(0.,0.168000000000001),
 .UNSPECIFIED.);
#1262=FACE_BOUND('',#5724,.T.);
#1263=FACE_BOUND('',#5725,.T.);
#1264=FACE_BOUND('',#5726,.T.);
#1265=FACE_BOUND('',#5728,.T.);
#1266=FACE_BOUND('',#5729,.T.);
#1267=FACE_BOUND('',#5730,.T.);
#1469=B_SPLINE_CURVE_WITH_KNOTS('',3,(#57910,#57911,#57912,#57913,#57914,
#57915,#57916,#57917,#57918,#57919,#57920,#57921,#57922,#57923,#57924,#57925,
#57926,#57927,#57928,#57929,#57930,#57931,#57932,#57933,#57934,#57935,#57936,
#57937,#57938,#57939,#57940,#57941,#57942,#57943,#57944,#57945,#57946,#57947,
#57948,#57949,#57950,#57951,#57952,#57953,#57954,#57955,#57956,#57957,#57958,
#57959,#57960,#57961,#57962,#57963,#57964,#57965,#57966,#57967,#57968,#57969,
#57970,#57971,#57972,#57973,#57974,#57975,#57976,#57977,#57978,#57979,#57980,
#57981,#57982,#57983,#57984,#57985,#57986,#57987,#57988,#57989,#57990,#57991,
#57992,#57993,#57994,#57995,#57996,#57997,#57998,#57999,#58000,#58001,#58002,
#58003,#58004,#58005,#58006,#58007,#58008,#58009,#58010,#58011,#58012,#58013,
#58014,#58015,#58016,#58017,#58018,#58019,#58020,#58021,#58022,#58023,#58024,
#58025,#58026,#58027,#58028,#58029,#58030,#58031,#58032,#58033,#58034,#58035,
#58036,#58037,#58038,#58039,#58040,#58041,#58042,#58043,#58044,#58045,#58046,
#58047,#58048,#58049,#58050,#58051,#58052,#58053,#58054,#58055,#58056,#58057,
#58058,#58059,#58060,#58061,#58062,#58063,#58064,#58065,#58066,#58067,#58068,
#58069,#58070,#58071,#58072,#58073,#58074,#58075,#58076,#58077,#58078,#58079,
#58080,#58081,#58082,#58083,#58084,#58085,#58086,#58087,#58088,#58089,#58090,
#58091,#58092,#58093,#58094,#58095,#58096,#58097,#58098,#58099,#58100,#58101,
#58102,#58103,#58104,#58105,#58106,#58107,#58108,#58109,#58110,#58111,#58112,
#58113,#58114),.UNSPECIFIED.,.F.,.F.,(4,3,3,3,3,3,3,3,3,3,3,3,3,3,3,3,3,
3,3,3,3,3,3,3,3,3,3,3,3,3,3,3,3,3,3,3,3,3,3,3,3,3,3,3,3,3,3,3,3,3,3,3,3,
3,3,3,3,3,3,3,3,3,3,3,3,3,3,3,4),(13.309352184,13.323137025,13.3863594433,
14.12420843155,14.8856731093313,15.6888539595427,15.9597639966,16.8873511174641,
17.1203737742,18.1372619540516,18.2809835519,19.3636219067,20.2587429271837,
21.0960175022786,21.871126775755,22.6115369711,23.3438450692561,24.1167746190937,
24.9325083938468,25.7482421686,26.5792532013888,26.7015351032,27.4472809428227,
27.6548280379,28.374603752275,29.127256650775,29.8622469410304,30.8120080950777,
31.5487524214573,32.4808930871787,33.2657987908602,33.4130337529,34.437297417812,
35.4455607682181,36.2352334697,37.0820276885765,37.6463786218,38.4082532030519,
39.0575237739,40.2132927109806,41.3296198963854,42.1466787398524,43.4466846508938,
44.6786014526,46.0833739199895,47.3981772916748,47.4881463873789,48.0675133951128,
49.1826023586064,49.7401468403532,50.2346525230349,50.2976913221,50.6043371871572,
50.9220054878,51.2478630104204,51.5463196535,51.8055359260692,51.8585343078,
51.9934642813463,52.1351368654365,52.1707489621,52.3315300267018,52.511597748187,
52.7592184635403,52.9463039716658,53.1109033767957,53.2581518689432,53.4032370372,
53.4991626515),.UNSPECIFIED.);
#1470=B_SPLINE_CURVE_WITH_KNOTS('',3,(#58118,#58119,#58120,#58121,#58122,
#58123,#58124,#58125,#58126,#58127,#58128,#58129,#58130,#58131,#58132,#58133,
#58134,#58135,#58136,#58137,#58138,#58139,#58140,#58141,#58142,#58143,#58144,
#58145,#58146,#58147,#58148,#58149,#58150,#58151,#58152,#58153,#58154,#58155,
#58156,#58157,#58158,#58159,#58160,#58161,#58162,#58163,#58164,#58165,#58166,
#58167,#58168,#58169,#58170,#58171,#58172,#58173,#58174,#58175,#58176,#58177,
#58178,#58179,#58180,#58181,#58182,#58183,#58184,#58185,#58186,#58187,#58188,
#58189,#58190,#58191,#58192,#58193,#58194,#58195,#58196,#58197,#58198,#58199,
#58200,#58201,#58202,#58203,#58204,#58205,#58206,#58207,#58208,#58209,#58210,
#58211,#58212,#58213,#58214,#58215,#58216,#58217,#58218,#58219,#58220,#58221,
#58222,#58223,#58224,#58225,#58226,#58227,#58228,#58229,#58230,#58231,#58232,
#58233,#58234,#58235,#58236,#58237,#58238,#58239,#58240,#58241,#58242,#58243,
#58244,#58245,#58246,#58247,#58248,#58249,#58250,#58251,#58252,#58253,#58254,
#58255,#58256,#58257,#58258,#58259,#58260,#58261,#58262,#58263,#58264,#58265,
#58266,#58267,#58268,#58269,#58270,#58271,#58272,#58273,#58274,#58275,#58276,
#58277,#58278,#58279,#58280,#58281,#58282,#58283,#58284,#58285,#58286,#58287,
#58288,#58289,#58290,#58291,#58292,#58293,#58294,#58295,#58296,#58297,#58298,
#58299,#58300,#58301,#58302,#58303,#58304,#58305,#58306,#58307),
 .UNSPECIFIED.,.F.,.F.,(4,3,3,3,3,3,3,3,3,3,3,3,3,3,3,3,3,3,3,3,3,3,3,3,
3,3,3,3,3,3,3,3,3,3,3,3,3,3,3,3,3,3,3,3,3,3,3,3,3,3,3,3,3,3,3,3,3,3,3,3,
3,3,3,4),(13.0484209298,13.1985929592139,13.3595276799308,13.5385979322865,
13.7128016785,13.9893591774131,14.1906327377194,14.3771824271,14.54326308795,
14.7093437488,14.8963499782689,15.0415050705,15.2816537737298,15.5279902136833,
15.7058202332,16.5863775357757,17.5955458670479,18.9061966866262,19.4329797586,
20.311266855424,21.4702806672064,22.2257607493,23.6221512447,24.8448189225224,
25.0185417401,26.1279357243721,26.4232309792,27.450845739338,27.8279202183,
28.6310179366367,29.2326020624,30.0907997879616,30.6372839066,31.5630151799466,
32.5503655253306,33.4574539385,34.2879035210213,35.1589507142178,36.1110388869914,
36.2776239705,37.3654001731742,38.3930371789532,39.2955654086294,40.0450320001,
40.856499728,41.6679674559,42.4694699238593,43.2917945237491,44.136915507971,
45.0204388110303,45.9236134063345,46.84816360524,47.6452295392,48.4005579590137,
48.7814448095,49.8245939850343,49.9176600797,50.7203463862896,51.4551652964948,
52.1093626235535,52.1899842067,52.795745757086,53.2289587759,53.2420797137),
 .UNSPECIFIED.);
#1471=B_SPLINE_CURVE_WITH_KNOTS('',3,(#58309,#58310,#58311,#58312,#58313,
#58314,#58315,#58316,#58317,#58318,#58319,#58320,#58321,#58322,#58323,#58324,
#58325,#58326,#58327,#58328,#58329,#58330,#58331,#58332,#58333,#58334,#58335,
#58336,#58337,#58338,#58339,#58340,#58341,#58342,#58343,#58344,#58345,#58346,
#58347,#58348,#58349,#58350,#58351,#58352,#58353,#58354,#58355,#58356,#58357,
#58358,#58359,#58360,#58361,#58362,#58363,#58364,#58365,#58366,#58367,#58368,
#58369,#58370,#58371,#58372,#58373,#58374,#58375,#58376,#58377,#58378,#58379,
#58380,#58381,#58382,#58383,#58384,#58385,#58386,#58387,#58388,#58389,#58390,
#58391,#58392,#58393,#58394,#58395,#58396,#58397,#58398,#58399),
 .UNSPECIFIED.,.F.,.F.,(4,3,3,3,3,3,3,3,3,3,3,3,3,3,3,3,3,3,3,3,3,3,3,3,
3,3,3,3,3,3,4),(1.97579103232,2.07828074772114,2.18503422566924,2.30151093703245,
2.35860134499,2.50402104555128,2.68267531807239,2.74141165766,2.9137457614164,
2.93383581469,3.09971901414853,3.12625997171,3.28520678839759,3.44068202460021,
3.51110670868,3.93194807809976,4.27919611191,4.63210924602733,4.95850770531841,
5.05016737922,5.36028985569995,5.73870525373494,5.82385208673,6.211020287495,
6.51428680619734,6.59818848826,6.86631471668985,7.1224741520835,7.36521342880379,
7.47414519692,7.48619339243),.UNSPECIFIED.);
#1472=B_SPLINE_CURVE_WITH_KNOTS('',3,(#58401,#58402,#58403,#58404,#58405,
#58406,#58407,#58408,#58409,#58410,#58411,#58412,#58413,#58414,#58415,#58416,
#58417,#58418,#58419,#58420,#58421,#58422,#58423,#58424,#58425,#58426,#58427,
#58428,#58429,#58430,#58431,#58432,#58433,#58434,#58435,#58436,#58437,#58438,
#58439,#58440,#58441,#58442,#58443,#58444,#58445,#58446,#58447,#58448,#58449,
#58450,#58451,#58452,#58453,#58454,#58455,#58456,#58457,#58458,#58459,#58460,
#58461,#58462,#58463,#58464,#58465,#58466,#58467,#58468,#58469,#58470,#58471,
#58472,#58473,#58474,#58475,#58476,#58477,#58478,#58479,#58480,#58481,#58482,
#58483,#58484,#58485,#58486,#58487,#58488),.UNSPECIFIED.,.F.,.F.,(4,3,3,
3,3,3,3,3,3,3,3,3,3,3,3,3,3,3,3,3,3,3,3,3,3,3,3,3,3,4),(3.98757792105,4.37296381107402,
4.83010470053207,5.42700834471868,5.7540471061,5.91552193819,6.24545979117289,
6.5613910649,6.72371295995,6.886034855,7.21067302107,7.63677556282134,8.032077392405,
8.37387398489675,8.51083290938,8.83623063238,9.16162835537,9.58330595607059,
9.81286749338,10.1385220868,10.4641766803,10.8560732769984,11.1157021879,
11.4414966369,11.7672910859,12.2101021764744,12.6468293861861,13.074381154517,
13.1814695027,13.2292989355),.UNSPECIFIED.);
#1473=B_SPLINE_CURVE_WITH_KNOTS('',3,(#58490,#58491,#58492,#58493,#58494,
#58495,#58496,#58497,#58498,#58499,#58500,#58501,#58502,#58503,#58504,#58505,
#58506,#58507,#58508,#58509,#58510,#58511,#58512,#58513,#58514,#58515,#58516,
#58517,#58518,#58519,#58520,#58521,#58522,#58523,#58524,#58525,#58526,#58527,
#58528,#58529,#58530,#58531,#58532,#58533,#58534,#58535,#58536,#58537,#58538,
#58539,#58540,#58541,#58542,#58543,#58544,#58545,#58546,#58547,#58548,#58549,
#58550,#58551,#58552,#58553,#58554,#58555,#58556),.UNSPECIFIED.,.F.,.F.,
(4,3,3,3,3,3,3,3,3,3,3,3,3,3,3,3,3,3,3,3,3,3,4),(0.620884089829,0.716822013874948,
0.814811640695407,0.84119531409,0.940509199950627,1.04043228231547,1.06766803527,
1.16714488691394,1.26514484762101,1.29421245021,1.39419772064502,1.49551599200885,
1.52004026842,1.62238868361275,1.72429183399409,1.7458581253,1.84548984945833,
1.94348709363021,1.972411509,2.0695360714935,2.14245735488,2.17079617383,
2.17770970576),.UNSPECIFIED.);
#1474=B_SPLINE_CURVE_WITH_KNOTS('',3,(#58558,#58559,#58560,#58561,#58562,
#58563,#58564,#58565,#58566,#58567,#58568,#58569,#58570,#58571,#58572,#58573,
#58574,#58575,#58576,#58577,#58578,#58579,#58580,#58581,#58582,#58583,#58584,
#58585,#58586,#58587,#58588,#58589,#58590,#58591,#58592,#58593,#58594,#58595,
#58596,#58597,#58598,#58599,#58600,#58601,#58602,#58603,#58604,#58605,#58606,
#58607,#58608,#58609,#58610,#58611,#58612,#58613,#58614,#58615,#58616,#58617,
#58618,#58619,#58620,#58621,#58622,#58623,#58624),.UNSPECIFIED.,.F.,.F.,
(4,3,3,3,3,3,3,3,3,3,3,3,3,3,3,3,3,3,3,3,3,3,4),(8.86873667877,9.56765456322511,
10.2729436861767,10.9878758752376,11.7077824777404,12.4350615145002,13.0838534898,
13.8192347398744,14.5574383601605,15.2977913928285,16.0381171761183,16.7766041138207,
17.3137864161,18.0504471780062,18.7845067021332,19.5160468171481,20.2444500253411,
20.9691816021643,21.6873308194927,22.4015170165044,23.1087844511325,23.7914150129,
23.7986943084),.UNSPECIFIED.);
#1475=B_SPLINE_CURVE_WITH_KNOTS('',3,(#58626,#58627,#58628,#58629,#58630,
#58631,#58632,#58633,#58634,#58635,#58636,#58637,#58638,#58639,#58640,#58641,
#58642,#58643,#58644,#58645,#58646,#58647,#58648,#58649,#58650,#58651,#58652,
#58653,#58654,#58655,#58656,#58657,#58658,#58659,#58660,#58661,#58662,#58663,
#58664,#58665,#58666,#58667,#58668,#58669,#58670,#58671,#58672,#58673,#58674,
#58675,#58676,#58677,#58678,#58679,#58680,#58681,#58682,#58683,#58684,#58685,
#58686,#58687,#58688,#58689,#58690,#58691,#58692),.UNSPECIFIED.,.F.,.F.,
(4,3,3,3,3,3,3,3,3,3,3,3,3,3,3,3,3,3,3,3,3,3,4),(8.86900274924736,9.56791953010357,
10.2732073750769,10.9881379920343,11.7080429074792,12.4353200096991,13.0840615029,
13.8194427527924,14.5576463730041,15.2979994057468,16.0383251891797,16.7768121271005,
17.3139944292,18.0506551916125,18.7847147159344,19.5162548309688,20.2446580390238,
20.9693896155684,21.6875388324433,22.401725028926,23.1089924629253,23.7916230261,
23.7989023215),.UNSPECIFIED.);
#1476=B_SPLINE_CURVE_WITH_KNOTS('',3,(#58694,#58695,#58696,#58697,#58698,
#58699,#58700,#58701,#58702,#58703,#58704,#58705,#58706,#58707,#58708,#58709,
#58710,#58711,#58712,#58713,#58714,#58715,#58716,#58717,#58718,#58719,#58720,
#58721,#58722,#58723,#58724,#58725,#58726,#58727,#58728,#58729,#58730,#58731,
#58732,#58733,#58734,#58735,#58736,#58737,#58738,#58739,#58740,#58741,#58742,
#58743,#58744,#58745,#58746,#58747,#58748,#58749,#58750,#58751,#58752,#58753,
#58754,#58755,#58756,#58757,#58758,#58759,#58760),.UNSPECIFIED.,.F.,.F.,
(4,3,3,3,3,3,3,3,3,3,3,3,3,3,3,3,3,3,3,3,3,3,4),(0.620886007027,0.716872155729975,
0.814917720645,0.84119723129,0.940511117480007,1.04043420022721,1.06766995247,
1.16714680417379,1.26514676496046,1.29421436741,1.39419963807593,1.49551790965784,
1.52004218562,1.62239060093022,1.72429375142684,1.7458600425,1.84549176711273,
1.94348901169251,1.97241342619,2.06953798933515,2.14245927208,2.17079809103,
2.17771162296),.UNSPECIFIED.);
#1477=B_SPLINE_CURVE_WITH_KNOTS('',3,(#58762,#58763,#58764,#58765,#58766,
#58767,#58768,#58769,#58770,#58771,#58772,#58773,#58774,#58775,#58776,#58777,
#58778,#58779,#58780,#58781,#58782,#58783,#58784,#58785,#58786,#58787,#58788,
#58789,#58790,#58791,#58792,#58793,#58794,#58795,#58796,#58797,#58798,#58799,
#58800,#58801,#58802,#58803,#58804,#58805,#58806,#58807,#58808,#58809,#58810,
#58811,#58812,#58813,#58814,#58815,#58816,#58817,#58818,#58819,#58820,#58821,
#58822,#58823,#58824,#58825,#58826,#58827,#58828,#58829,#58830,#58831,#58832,
#58833,#58834,#58835,#58836,#58837,#58838,#58839,#58840,#58841,#58842,#58843,
#58844,#58845,#58846,#58847,#58848,#58849,#58850,#58851,#58852,#58853,#58854,
#58855,#58856,#58857,#58858),.UNSPECIFIED.,.F.,.F.,(4,3,3,3,3,3,3,3,3,3,
3,3,3,3,3,3,3,3,3,3,3,3,3,3,3,3,3,3,3,3,3,3,4),(3.96957835788,4.39597160341197,
4.83142631025598,5.2668810171,5.57677617355175,5.86532271174004,6.02614087237832,
6.40225920003408,6.59503115748336,6.95548992077255,7.25795107039535,7.67923093688714,
7.87144621262,8.29346059413677,8.52280966994,8.93355714097029,9.17417312726,
9.58477382996718,9.97944876858222,10.3091559889411,10.4557118199803,10.571368793377,
10.6388632093,10.8013830785,11.1075435152645,11.126417564,11.3027365160323,
11.4514500011,11.9118977470061,12.4712067694839,12.8675106802888,13.1811526769,
13.2112648606),.UNSPECIFIED.);
#1478=B_SPLINE_CURVE_WITH_KNOTS('',3,(#58859,#58860,#58861,#58862,#58863,
#58864,#58865,#58866,#58867,#58868,#58869,#58870,#58871,#58872,#58873,#58874,
#58875,#58876,#58877,#58878,#58879,#58880,#58881,#58882,#58883,#58884,#58885,
#58886,#58887,#58888,#58889,#58890,#58891,#58892,#58893,#58894,#58895,#58896,
#58897,#58898,#58899,#58900,#58901,#58902,#58903,#58904,#58905,#58906,#58907,
#58908,#58909,#58910,#58911,#58912,#58913,#58914,#58915,#58916,#58917,#58918,
#58919,#58920,#58921,#58922,#58923,#58924,#58925,#58926,#58927,#58928,#58929,
#58930,#58931,#58932,#58933,#58934,#58935,#58936,#58937,#58938,#58939,#58940,
#58941,#58942,#58943,#58944,#58945,#58946,#58947,#58948,#58949),
 .UNSPECIFIED.,.F.,.F.,(4,3,3,3,3,3,3,3,3,3,3,3,3,3,3,3,3,3,3,3,3,3,3,3,
3,3,3,3,3,3,4),(2.79870510475,3.04393466036784,3.30656708431892,3.56919950827,
3.86702674427847,4.2250471626441,4.34415602331,4.63129409529021,4.73138788155,
5.07553416287892,5.11861973979,5.505577329925,5.82824217543653,5.89253492006,
6.12297607298855,6.2782762368,6.62203670021294,6.66401755354,6.8891214006705,
7.08746626879966,7.24045509522,7.33801757407394,7.43260181799,7.54635634529559,
7.67608056663181,7.84610920044259,7.96861479261622,8.07891483464399,8.17911016106332,
8.26392367279,8.30631830913),.UNSPECIFIED.);
#1479=B_SPLINE_CURVE_WITH_KNOTS('',3,(#58952,#58953,#58954,#58955,#58956,
#58957,#58958,#58959,#58960,#58961,#58962,#58963,#58964,#58965,#58966,#58967,
#58968,#58969,#58970,#58971,#58972,#58973,#58974,#58975,#58976,#58977,#58978,
#58979,#58980,#58981,#58982,#58983,#58984,#58985,#58986,#58987,#58988,#58989,
#58990,#58991,#58992,#58993,#58994,#58995,#58996,#58997,#58998,#58999,#59000,
#59001,#59002,#59003,#59004,#59005,#59006,#59007,#59008,#59009,#59010,#59011,
#59012,#59013,#59014,#59015),.UNSPECIFIED.,.F.,.F.,(4,3,3,3,3,3,3,3,3,3,
3,3,3,3,3,3,3,3,3,3,3,4),(2.24719882413,2.47950959664509,2.7181592241886,
2.88911799452,3.14833691195321,3.42802670540373,3.53895765179,3.70165384248,
3.86435003317,4.18973836725,4.51381221186,4.79860489658347,4.83788605646,
5.12465109548868,5.4094896631728,5.69059563897099,5.96386594048412,6.23240174493241,
6.4936877081412,6.75497367135,6.83535944365,6.83969663211),
 .UNSPECIFIED.);
#1480=B_SPLINE_CURVE_WITH_KNOTS('',3,(#59017,#59018,#59019,#59020,#59021,
#59022,#59023,#59024,#59025,#59026,#59027,#59028,#59029,#59030,#59031,#59032,
#59033,#59034,#59035,#59036,#59037,#59038,#59039,#59040,#59041,#59042,#59043,
#59044,#59045,#59046,#59047,#59048,#59049,#59050,#59051,#59052,#59053,#59054,
#59055,#59056,#59057,#59058,#59059,#59060,#59061,#59062,#59063,#59064,#59065,
#59066,#59067,#59068,#59069,#59070,#59071,#59072,#59073,#59074,#59075,#59076,
#59077,#59078,#59079,#59080,#59081,#59082,#59083,#59084,#59085,#59086,#59087,
#59088,#59089,#59090,#59091,#59092,#59093,#59094,#59095,#59096,#59097,#59098,
#59099,#59100,#59101,#59102,#59103,#59104,#59105,#59106,#59107,#59108,#59109,
#59110,#59111,#59112,#59113,#59114,#59115,#59116,#59117,#59118,#59119,#59120,
#59121,#59122,#59123,#59124,#59125,#59126,#59127,#59128,#59129,#59130,#59131,
#59132,#59133,#59134,#59135,#59136,#59137),.UNSPECIFIED.,.F.,.F.,(4,3,3,
3,3,3,3,3,3,3,3,3,3,3,3,3,3,3,3,3,3,3,3,3,3,3,3,3,3,3,3,3,3,3,3,3,3,3,3,
3,4),(3.85962234114,4.19972391890181,4.53697841171985,4.869784285439,5.02187433899,
5.35760123169367,5.6906544867354,6.02105657040899,6.1874356314,6.45638966870391,
6.48278728797,6.74353369413089,6.90031644081217,7.10197837175744,7.30053328201393,
7.48704833849445,7.75167375530052,8.00411859419973,8.16908321302,8.40987017981997,
8.57068233883,8.77146651417,8.9722506895,9.22816232252967,9.48818563062432,
9.76109275858924,9.87702506481,10.1302745068855,10.1785749125,10.4351702200345,
10.4731717655,10.6204752146,10.7677786637,11.0253091767098,11.2837011973151,
11.3568793877,11.4511218437,11.7091168167062,11.9603884154845,12.1758537261,
12.1808522654),.UNSPECIFIED.);
#1481=B_SPLINE_CURVE_WITH_KNOTS('',3,(#59139,#59140,#59141,#59142,#59143,
#59144,#59145,#59146,#59147,#59148,#59149,#59150,#59151,#59152,#59153,#59154,
#59155,#59156,#59157,#59158,#59159,#59160,#59161,#59162,#59163,#59164,#59165,
#59166,#59167,#59168,#59169,#59170,#59171,#59172,#59173,#59174,#59175,#59176,
#59177,#59178,#59179,#59180,#59181,#59182,#59183,#59184,#59185,#59186,#59187,
#59188,#59189,#59190,#59191,#59192,#59193,#59194,#59195,#59196,#59197,#59198,
#59199,#59200,#59201,#59202,#59203,#59204,#59205,#59206,#59207,#59208,#59209,
#59210,#59211,#59212,#59213,#59214,#59215,#59216,#59217,#59218,#59219,#59220,
#59221,#59222,#59223,#59224,#59225,#59226,#59227,#59228,#59229,#59230,#59231,
#59232,#59233,#59234,#59235,#59236,#59237,#59238,#59239,#59240,#59241,#59242,
#59243,#59244,#59245,#59246,#59247,#59248,#59249,#59250,#59251,#59252,#59253,
#59254,#59255,#59256,#59257,#59258,#59259,#59260,#59261,#59262,#59263,#59264,
#59265,#59266,#59267,#59268,#59269,#59270,#59271,#59272,#59273,#59274,#59275,
#59276,#59277,#59278,#59279,#59280),.UNSPECIFIED.,.F.,.F.,(4,3,3,3,3,3,
3,3,3,3,3,3,3,3,3,3,3,3,3,3,3,3,3,3,3,3,3,3,3,3,3,3,3,3,3,3,3,3,3,3,3,3,
3,3,3,3,3,4),(4.50366397293,4.99124165569177,5.43037471844,5.89373484028,
6.35709496212,6.90400455685533,7.47912691149025,8.11630634984611,8.22021331127,
9.00207087590175,9.73645569725131,10.0610358316502,10.3759242294803,10.9668836400114,
11.5102521272997,11.9396101613,12.4394822515178,12.8992348856666,13.3423310076333,
13.7422758054098,13.7854271296,14.0100730382075,14.3250384976331,14.562738268668,
14.7102740046,14.9084134032829,14.9414943029,15.0571045639,15.1727148249,
15.3067326045136,15.4308105599538,15.5448300326044,15.6351526747,15.8376558220379,
15.9751983688068,16.095274225,16.2103083328,16.3187818774064,16.3253424406,
16.4403769587,16.6325985794226,16.8436821336366,17.1067596509336,17.3700673761745,
17.5731317933866,17.7244288223,17.7659084738,17.7760995894),
 .UNSPECIFIED.);
#1482=B_SPLINE_CURVE_WITH_KNOTS('',3,(#59284,#59285,#59286,#59287,#59288,
#59289,#59290,#59291,#59292,#59293,#59294,#59295,#59296,#59297,#59298,#59299,
#59300,#59301,#59302,#59303,#59304,#59305,#59306,#59307,#59308,#59309,#59310,
#59311,#59312,#59313,#59314,#59315,#59316,#59317,#59318,#59319,#59320,#59321,
#59322,#59323),.UNSPECIFIED.,.F.,.F.,(4,3,3,3,3,3,3,3,3,3,3,3,3,4),(0.591274134056,
0.737771024646977,0.884305624855233,1.0207914158492,1.15221742139287,1.27912445533491,
1.32390942548,1.45709767839612,1.50719219233,1.64441133416022,1.6904452675,
1.83867829106087,1.87380304476,1.88642149695),.UNSPECIFIED.);
#1483=B_SPLINE_CURVE_WITH_KNOTS('',3,(#59327,#59328,#59329,#59330,#59331,
#59332,#59333,#59334,#59335,#59336,#59337,#59338,#59339,#59340,#59341,#59342,
#59343,#59344,#59345,#59346,#59347,#59348,#59349,#59350,#59351,#59352,#59353,
#59354,#59355,#59356,#59357,#59358,#59359,#59360,#59361,#59362,#59363,#59364,
#59365,#59366,#59367,#59368,#59369,#59370,#59371,#59372,#59373,#59374,#59375,
#59376,#59377,#59378,#59379,#59380,#59381),.UNSPECIFIED.,.F.,.F.,(4,3,3,
3,3,3,3,3,3,3,3,3,3,3,3,3,3,3,4),(1.62532205434,1.8292510625355,2.03769001760317,
2.06608094185,2.288761226025,2.50697787928773,2.73188997891886,2.95680207855,
3.18629283499015,3.41149746017445,3.63033389632304,3.84717522696,4.06984785891,
4.27735501742918,4.29252049086,4.52218882627,4.73290113316675,4.75185716168,
4.7566717002),.UNSPECIFIED.);
#1484=B_SPLINE_CURVE_WITH_KNOTS('',3,(#59384,#59385,#59386,#59387,#59388,
#59389,#59390,#59391,#59392,#59393,#59394,#59395,#59396,#59397,#59398,#59399,
#59400,#59401,#59402,#59403,#59404,#59405,#59406,#59407,#59408,#59409,#59410,
#59411,#59412,#59413,#59414,#59415,#59416,#59417,#59418,#59419,#59420,#59421,
#59422,#59423,#59424,#59425,#59426,#59427,#59428,#59429,#59430,#59431,#59432,
#59433,#59434,#59435,#59436,#59437,#59438,#59439,#59440,#59441,#59442,#59443,
#59444,#59445,#59446,#59447,#59448,#59449,#59450,#59451,#59452,#59453,#59454,
#59455,#59456,#59457,#59458,#59459,#59460,#59461,#59462,#59463,#59464,#59465,
#59466,#59467,#59468,#59469,#59470,#59471,#59472,#59473,#59474,#59475,#59476,
#59477,#59478,#59479,#59480,#59481,#59482,#59483,#59484,#59485,#59486,#59487,
#59488,#59489,#59490,#59491,#59492,#59493,#59494,#59495,#59496,#59497,#59498,
#59499,#59500,#59501,#59502,#59503,#59504,#59505,#59506,#59507,#59508,#59509,
#59510,#59511,#59512,#59513,#59514,#59515,#59516,#59517,#59518,#59519,#59520,
#59521,#59522,#59523,#59524,#59525,#59526,#59527,#59528,#59529,#59530,#59531,
#59532,#59533,#59534),.UNSPECIFIED.,.F.,.F.,(4,3,3,3,3,3,3,3,3,3,3,3,3,
3,3,3,3,3,3,3,3,3,3,3,3,3,3,3,3,3,3,3,3,3,3,3,3,3,3,3,3,3,3,3,3,3,3,3,3,
3,4),(12.5665153092,12.69009921,13.2174016095,13.8698869846695,14.5642289168119,
15.3151925132145,16.0388958,16.8581279061159,17.6625886056314,17.9101510626,
18.6238243777442,18.8458744215,19.5096373001485,19.7815977804,20.44584529895,
21.059648595772,21.1100928175,21.7276111632648,22.3653169829574,22.4385878545,
23.124225370433,23.8648590976465,24.6494567737865,25.5236748237381,25.7297732797,
26.6264022970681,27.4702545905334,27.520500466,28.2933349196177,29.0051511936574,
29.3112276523,30.1086473503047,30.901548854693,31.6539457983,32.4171630493237,
32.8253410695,33.5504490487425,33.9967363407,34.9585356035503,36.0043997832878,
37.2106334827439,38.3142574004481,38.6616811225,39.8017790454581,40.9619707819579,
42.1851664159684,43.362585886113,44.531567646397,45.6794320868491,45.854753318,
45.9550547113),.UNSPECIFIED.);
#1485=B_SPLINE_CURVE_WITH_KNOTS('',3,(#59539,#59540,#59541,#59542,#59543,
#59544,#59545,#59546,#59547,#59548,#59549,#59550,#59551,#59552,#59553,#59554,
#59555,#59556,#59557,#59558,#59559,#59560,#59561,#59562,#59563,#59564,#59565,
#59566,#59567,#59568,#59569,#59570,#59571,#59572,#59573,#59574,#59575,#59576,
#59577,#59578,#59579,#59580,#59581,#59582,#59583,#59584,#59585,#59586,#59587,
#59588,#59589,#59590),.UNSPECIFIED.,.F.,.F.,(4,3,3,3,3,3,3,3,3,3,3,3,3,
3,3,3,3,4),(1.6242031795,1.7641955129598,1.91480668054345,2.07466312403716,
2.24808422551421,2.44933142681594,2.68661595806518,2.86896453197481,2.95435751105114,
3.20515307109064,3.44947321600323,3.68472165312646,3.91086811604638,4.12470379479479,
4.33276956159462,4.54416084712731,4.74069692760198,4.75555213266),
 .UNSPECIFIED.);
#1486=B_SPLINE_CURVE_WITH_KNOTS('',3,(#59594,#59595,#59596,#59597,#59598,
#59599,#59600,#59601,#59602,#59603,#59604,#59605,#59606,#59607,#59608,#59609,
#59610,#59611,#59612,#59613,#59614,#59615,#59616,#59617,#59618,#59619,#59620,
#59621,#59622,#59623,#59624,#59625,#59626,#59627,#59628,#59629,#59630,#59631,
#59632,#59633),.UNSPECIFIED.,.F.,.F.,(4,3,3,3,3,3,3,3,3,3,3,3,3,4),(0.591273571839,
0.737752285807162,0.879766304409762,0.957377792997,1.09086433302759,1.21862527059374,
1.32390886326,1.4570971165661,1.50719163011,1.64441077088749,1.69044470528,
1.83867772392408,1.87380248254,1.88642093473),.UNSPECIFIED.);
#1487=B_SPLINE_CURVE_WITH_KNOTS('',3,(#59637,#59638,#59639,#59640,#59641,
#59642,#59643,#59644,#59645,#59646,#59647,#59648,#59649,#59650,#59651,#59652,
#59653,#59654,#59655,#59656,#59657,#59658,#59659,#59660,#59661,#59662,#59663,
#59664,#59665,#59666,#59667,#59668,#59669,#59670,#59671,#59672,#59673,#59674,
#59675,#59676,#59677,#59678,#59679,#59680,#59681,#59682,#59683,#59684,#59685,
#59686,#59687,#59688,#59689,#59690,#59691,#59692,#59693,#59694,#59695,#59696,
#59697,#59698,#59699,#59700,#59701,#59702,#59703,#59704,#59705,#59706,#59707,
#59708,#59709,#59710,#59711,#59712,#59713,#59714,#59715,#59716,#59717,#59718,
#59719,#59720,#59721,#59722,#59723,#59724,#59725,#59726,#59727,#59728,#59729,
#59730,#59731,#59732,#59733,#59734,#59735,#59736,#59737,#59738,#59739,#59740,
#59741,#59742,#59743,#59744,#59745,#59746,#59747,#59748,#59749,#59750,#59751,
#59752,#59753,#59754,#59755,#59756,#59757,#59758,#59759,#59760,#59761,#59762,
#59763,#59764,#59765,#59766,#59767,#59768,#59769,#59770,#59771,#59772,#59773,
#59774,#59775,#59776,#59777,#59778,#59779,#59780,#59781),.UNSPECIFIED.,
 .F.,.F.,(4,3,3,3,3,3,3,3,3,3,3,3,3,3,3,3,3,3,3,3,3,3,3,3,3,3,3,3,3,3,3,
3,3,3,3,3,3,3,3,3,3,3,3,3,3,3,3,3,4),(2.49496263694,2.84179514601607,3.12358351517951,
3.37468226753677,3.6010877740917,3.75614411414,3.87078619317,4.03758016375783,
4.16768516830925,4.28156554397569,4.32934465344,4.49463348465464,4.68595286679397,
4.83083072763417,4.95658124471608,5.02650835018,5.14262441503,5.25238358605751,
5.25874047989,5.43431138791523,5.63242977425596,5.91002792811298,6.11508550569381,
6.18762608197,6.60014373032483,7.02708053772435,7.46356052808173,7.91555826554562,
8.03803358836,8.52379534643387,9.02744534056375,9.56874664025437,9.88322107258,
10.5307262920464,11.2570348591899,11.7377621928,12.397963307906,12.999665458703,
13.561841112136,13.6013676095,14.0675025336,14.3117517759605,14.5073368468212,
14.6122016308443,15.1160041712998,15.4419498048499,15.6049226216249,15.712383115035,
15.7678954384),.UNSPECIFIED.);
#1488=B_SPLINE_CURVE_WITH_KNOTS('',3,(#59783,#59784,#59785,#59786,#59787,
#59788,#59789,#59790,#59791,#59792,#59793,#59794,#59795,#59796,#59797,#59798,
#59799,#59800,#59801,#59802,#59803,#59804,#59805,#59806,#59807,#59808,#59809,
#59810,#59811,#59812,#59813,#59814,#59815,#59816,#59817,#59818,#59819,#59820,
#59821,#59822,#59823,#59824,#59825,#59826,#59827,#59828,#59829,#59830,#59831,
#59832,#59833,#59834,#59835,#59836,#59837,#59838,#59839,#59840,#59841,#59842,
#59843,#59844,#59845,#59846,#59847,#59848,#59849,#59850,#59851,#59852,#59853,
#59854,#59855,#59856,#59857,#59858,#59859,#59860,#59861,#59862,#59863,#59864,
#59865,#59866,#59867,#59868,#59869,#59870,#59871,#59872,#59873,#59874,#59875,
#59876,#59877,#59878,#59879,#59880,#59881,#59882,#59883,#59884,#59885,#59886,
#59887,#59888,#59889,#59890,#59891,#59892,#59893,#59894,#59895,#59896,#59897,
#59898,#59899,#59900,#59901,#59902,#59903,#59904,#59905,#59906,#59907,#59908,
#59909),.UNSPECIFIED.,.F.,.F.,(4,3,3,3,3,3,3,3,3,3,3,3,3,3,3,3,3,3,3,3,
3,3,3,3,3,3,3,3,3,3,3,3,3,3,3,3,3,3,3,3,3,3,4),(2.88912209896,3.13700724824184,
3.39458825543722,3.58392021798,3.72289252211,3.98628880886521,4.24665707065334,
4.28631003767,4.42907507566,4.57184011365,4.83048284543661,5.08100409555486,
5.1429678095,5.36927285077939,5.43868431146,5.67536287733583,5.73440081343,
5.98070533974942,6.0301432909,6.26817267571413,6.32588576837,6.57212979076101,
6.81101010914043,7.0391502779825,7.13061874999,7.36901534116979,7.53178369956,
7.73235096583,7.93291823211,8.20849768691155,8.4752234065794,8.6827158645,
8.83266433909,9.06554834733526,9.13254225469,9.45814484322078,9.78753654370285,
10.1215100985116,10.3109706634,10.6593104900296,10.8934901241,11.1848266494,
11.2103678193),.UNSPECIFIED.);
#1489=B_SPLINE_CURVE_WITH_KNOTS('',3,(#59911,#59912,#59913,#59914,#59915,
#59916,#59917,#59918,#59919,#59920,#59921,#59922,#59923,#59924,#59925,#59926,
#59927,#59928,#59929,#59930,#59931,#59932,#59933,#59934,#59935,#59936,#59937,
#59938,#59939,#59940,#59941,#59942,#59943,#59944,#59945,#59946,#59947,#59948,
#59949,#59950,#59951,#59952,#59953,#59954,#59955,#59956,#59957,#59958,#59959,
#59960,#59961,#59962,#59963,#59964,#59965,#59966,#59967,#59968,#59969,#59970,
#59971,#59972,#59973,#59974),.UNSPECIFIED.,.F.,.F.,(4,3,3,3,3,3,3,3,3,3,
3,3,3,3,3,3,3,3,3,3,3,4),(2.81282962644,3.06266228398076,3.32119792530808,
3.58514609404833,3.85885745601186,4.07803759972,4.36500988289161,4.66065264609048,
4.7151922635,5.01780193227688,5.03686033438,5.35852840527,5.72349096169794,
6.00613333041,6.30142940367959,6.33150425152,6.59883338343208,6.65687517263,
6.90228693396595,7.14631107564298,7.39033521732,7.40331879449),
 .UNSPECIFIED.);
#1490=B_SPLINE_CURVE_WITH_KNOTS('',3,(#59975,#59976,#59977,#59978,#59979,
#59980,#59981,#59982,#59983,#59984,#59985,#59986,#59987,#59988,#59989,#59990,
#59991,#59992,#59993,#59994,#59995,#59996,#59997,#59998,#59999,#60000,#60001,
#60002,#60003,#60004,#60005,#60006,#60007,#60008,#60009,#60010,#60011,#60012,
#60013,#60014,#60015,#60016,#60017,#60018,#60019,#60020,#60021,#60022,#60023,
#60024,#60025,#60026,#60027,#60028,#60029,#60030,#60031,#60032,#60033,#60034,
#60035,#60036,#60037,#60038,#60039,#60040,#60041,#60042,#60043,#60044,#60045,
#60046,#60047,#60048,#60049,#60050,#60051,#60052,#60053,#60054,#60055,#60056,
#60057,#60058,#60059,#60060,#60061,#60062,#60063,#60064,#60065,#60066,#60067,
#60068,#60069,#60070,#60071,#60072,#60073,#60074,#60075,#60076,#60077,#60078,
#60079,#60080,#60081,#60082,#60083,#60084,#60085,#60086,#60087,#60088,#60089,
#60090,#60091,#60092,#60093,#60094,#60095,#60096,#60097,#60098,#60099,#60100,
#60101,#60102,#60103,#60104,#60105,#60106,#60107,#60108,#60109,#60110,#60111,
#60112,#60113,#60114,#60115,#60116,#60117,#60118,#60119,#60120,#60121,#60122,
#60123,#60124,#60125),.UNSPECIFIED.,.F.,.F.,(4,3,3,3,3,3,3,3,3,3,3,3,3,
3,3,3,3,3,3,3,3,3,3,3,3,3,3,3,3,3,3,3,3,3,3,3,3,3,3,3,3,3,3,3,3,3,3,3,3,
3,4),(16.6199171728,16.7882414123,17.9571804763784,19.1237946395419,20.2651542998124,
21.4017824554562,22.4644640733447,22.5384106111,23.4876282272095,24.5248259815948,
25.1714775997893,25.8107789701635,26.8801413971835,27.8895685818,28.7828705984889,
29.2329471021,30.0685598834645,30.5763256225,31.5241408975413,32.4512947133434,
33.3589016805661,34.2400216773601,35.1072373135586,35.9553836369951,36.3852909182,
37.285084787083,37.9200729430749,38.3484054249084,39.078033259152,39.5193311416,
40.20147067805,40.8380785346705,40.8836102145,41.4881989858837,42.1149173319422,
42.2478892874,42.8850357315601,43.1836089333,43.8722843016629,44.1193285792,
44.8873595773554,45.7031826219889,45.990554775,46.7786481307242,47.5045421777594,
48.0421465447,48.7044889746508,49.3350094515254,49.827696459021,49.9655299284,
50.0065308028),.UNSPECIFIED.);
#1491=B_SPLINE_CURVE_WITH_KNOTS('',3,(#60128,#60129,#60130,#60131,#60132,
#60133,#60134,#60135,#60136,#60137,#60138,#60139,#60140,#60141,#60142,#60143,
#60144,#60145,#60146,#60147,#60148,#60149,#60150,#60151,#60152,#60153,#60154,
#60155,#60156,#60157,#60158,#60159,#60160,#60161,#60162,#60163,#60164,#60165,
#60166,#60167,#60168,#60169,#60170,#60171,#60172,#60173,#60174,#60175,#60176,
#60177,#60178,#60179,#60180,#60181,#60182,#60183,#60184,#60185,#60186,#60187,
#60188,#60189,#60190,#60191),.UNSPECIFIED.,.F.,.F.,(4,3,3,3,3,3,3,3,3,3,
3,3,3,3,3,3,3,3,3,3,3,4),(6.65601718416,7.29477936796371,7.93844920877978,
8.58674540795705,9.23928499675784,9.89729202723321,10.5577342961346,11.2208265785063,
11.623259991,12.2918631750371,12.960230968718,13.6273528326774,14.2922731198514,
14.9523209482512,15.6088709464739,16.2594069408208,16.6006372936,17.24679790118,
17.8853748974463,18.259922956,18.3634528429,18.3853430669),
 .UNSPECIFIED.);
#1492=B_SPLINE_CURVE_WITH_KNOTS('',3,(#60193,#60194,#60195,#60196,#60197,
#60198,#60199,#60200,#60201,#60202,#60203,#60204,#60205,#60206,#60207,#60208,
#60209,#60210,#60211,#60212,#60213,#60214,#60215,#60216,#60217,#60218,#60219,
#60220,#60221,#60222,#60223,#60224,#60225,#60226,#60227,#60228,#60229,#60230,
#60231,#60232,#60233,#60234,#60235,#60236,#60237,#60238,#60239,#60240,#60241,
#60242,#60243,#60244,#60245,#60246,#60247,#60248,#60249,#60250,#60251,#60252,
#60253,#60254,#60255,#60256,#60257,#60258,#60259,#60260,#60261,#60262,#60263,
#60264,#60265,#60266,#60267,#60268),.UNSPECIFIED.,.F.,.F.,(4,3,3,3,3,3,
3,3,3,3,3,3,3,3,3,3,3,3,3,3,3,3,3,3,3,4),(3.6079177031,3.90883706865,4.21466906474432,
4.53218264638424,4.8115951653,5.14200129762366,5.40176883821,5.76740314128159,
5.99194251112,6.37896984113116,6.80962623934222,7.28488360963019,7.76832519582,
8.20182855033449,8.64750474936071,9.07591953069402,9.50277466474551,9.79279299676506,
10.1847968843461,10.5613308583687,10.7833400669,11.1389210219272,11.4877159965757,
11.8269767713241,12.1534997188,12.1678629797),.UNSPECIFIED.);
#1493=B_SPLINE_CURVE_WITH_KNOTS('',3,(#60270,#60271,#60272,#60273,#60274,
#60275,#60276,#60277,#60278,#60279,#60280,#60281,#60282,#60283,#60284,#60285,
#60286,#60287,#60288,#60289,#60290,#60291,#60292,#60293,#60294,#60295,#60296,
#60297,#60298,#60299,#60300,#60301,#60302,#60303,#60304,#60305,#60306,#60307,
#60308,#60309,#60310,#60311,#60312,#60313,#60314,#60315,#60316,#60317,#60318,
#60319,#60320,#60321,#60322,#60323,#60324,#60325,#60326,#60327,#60328,#60329,
#60330,#60331,#60332,#60333,#60334,#60335,#60336,#60337,#60338,#60339,#60340,
#60341,#60342,#60343,#60344,#60345,#60346,#60347,#60348,#60349,#60350,#60351,
#60352,#60353,#60354,#60355,#60356,#60357,#60358,#60359,#60360,#60361,#60362,
#60363,#60364,#60365,#60366),.UNSPECIFIED.,.F.,.F.,(4,3,3,3,3,3,3,3,3,3,
3,3,3,3,3,3,3,3,3,3,3,3,3,3,3,3,3,3,3,3,3,3,4),(5.25334327713,5.71507679395458,
6.20067037733485,6.72422646913588,7.01125321047,7.45366970704,7.8960862036,
8.34468053427586,8.78087326212,9.21151474626878,9.65013812963318,10.1010680583122,
10.4599364913492,10.755057501583,11.212799144378,11.4506730327,11.8475195591173,
11.8957944479,12.3017989620678,12.3409158631,12.7831419415,13.2253680199,
13.7009269985786,14.1782614342998,14.6404182712168,14.9857329729,15.4237818735,
15.8618307742,16.3975356683301,16.9873115419291,17.6950030579161,17.8072669002,
17.830940375),.UNSPECIFIED.);
#1494=B_SPLINE_CURVE_WITH_KNOTS('',3,(#60370,#60371,#60372,#60373,#60374,
#60375,#60376,#60377,#60378,#60379,#60380,#60381,#60382,#60383,#60384,#60385,
#60386,#60387,#60388,#60389,#60390,#60391,#60392,#60393,#60394,#60395,#60396,
#60397,#60398,#60399,#60400,#60401,#60402,#60403,#60404,#60405,#60406,#60407,
#60408,#60409,#60410,#60411,#60412,#60413,#60414,#60415,#60416,#60417,#60418,
#60419,#60420,#60421,#60422,#60423,#60424,#60425,#60426,#60427,#60428,#60429,
#60430,#60431,#60432,#60433,#60434,#60435,#60436,#60437,#60438,#60439,#60440,
#60441,#60442,#60443,#60444,#60445,#60446,#60447,#60448,#60449,#60450,#60451,
#60452,#60453,#60454,#60455,#60456,#60457,#60458,#60459,#60460),
 .UNSPECIFIED.,.F.,.F.,(4,3,3,3,3,3,3,3,3,3,3,3,3,3,3,3,3,3,3,3,3,3,3,3,
3,3,3,3,3,3,4),(5.22957298235,5.72515531497929,6.23811612505594,6.78426433626665,
6.98390629531,7.59690004151861,7.87279845484386,8.57124459862821,8.73373254507,
9.17984086957932,9.60907313777,10.0483123491195,10.4844137305,10.8891125019663,
11.2738365701279,11.36693316,11.8065612589934,12.2352202864761,12.6835308024571,
13.1303519739113,13.5794071621556,14.0284623504,14.4735899231,14.9187174958,
15.3638712358,15.8090249758,16.318456840143,16.8416236232704,17.3572087860811,
17.7780978485,17.8070761317),.UNSPECIFIED.);
#1495=B_SPLINE_CURVE_WITH_KNOTS('',3,(#60462,#60463,#60464,#60465,#60466,
#60467,#60468,#60469,#60470,#60471,#60472,#60473,#60474,#60475,#60476,#60477,
#60478,#60479,#60480,#60481,#60482,#60483,#60484,#60485,#60486,#60487,#60488,
#60489,#60490,#60491,#60492,#60493,#60494,#60495,#60496,#60497,#60498,#60499,
#60500,#60501,#60502,#60503,#60504,#60505,#60506,#60507,#60508,#60509,#60510,
#60511,#60512,#60513,#60514,#60515,#60516,#60517,#60518,#60519,#60520,#60521,
#60522,#60523,#60524,#60525,#60526,#60527,#60528,#60529,#60530,#60531,#60532,
#60533,#60534,#60535,#60536,#60537,#60538,#60539,#60540,#60541,#60542,#60543,
#60544,#60545,#60546),.UNSPECIFIED.,.F.,.F.,(4,3,3,3,3,3,3,3,3,3,3,3,3,
3,3,3,3,3,3,3,3,3,3,3,3,3,3,3,4),(5.26516274934,5.60364973919554,5.94750904982777,
6.30061194587198,6.4671523865,6.83676658301042,7.2169534022643,7.60947300431465,
7.95473224321737,8.38000340982057,8.8249037638961,8.9008095338,9.35682876881741,
9.50401785273,9.99646091269704,10.1072261717,10.5612371713347,10.9769823432144,
11.366874414912,11.7306211259203,11.8905697622,12.1860647407,12.4815597193,
12.80236962685,13.1137390597323,13.4165240093164,13.7077321481745,13.7647993495,
13.8254388584),.UNSPECIFIED.);
#1496=B_SPLINE_CURVE_WITH_KNOTS('',3,(#60547,#60548,#60549,#60550,#60551,
#60552,#60553,#60554,#60555,#60556,#60557,#60558,#60559,#60560,#60561,#60562,
#60563,#60564,#60565,#60566,#60567,#60568,#60569,#60570,#60571,#60572,#60573,
#60574,#60575,#60576,#60577,#60578,#60579,#60580,#60581,#60582,#60583,#60584,
#60585,#60586,#60587,#60588,#60589,#60590,#60591,#60592,#60593,#60594,#60595,
#60596,#60597,#60598,#60599,#60600,#60601,#60602,#60603,#60604,#60605,#60606,
#60607),.UNSPECIFIED.,.F.,.F.,(4,3,3,3,3,3,3,3,3,3,3,3,3,3,3,3,3,3,3,3,
4),(6.656059514,6.70649596618,7.34364816588736,7.99077439543894,8.63810938722171,
9.29046036787606,9.94739592104111,10.610290255729,11.2756916426706,11.9437504407556,
12.5206580023,13.1894036939474,13.8555510001994,14.5190534443237,15.1792220023782,
15.8354746046203,16.4847448187666,17.1298267171795,17.7676868626226,18.3692626169,
18.3855563608),.UNSPECIFIED.);
#1497=B_SPLINE_CURVE_WITH_KNOTS('',3,(#60611,#60612,#60613,#60614,#60615,
#60616,#60617,#60618,#60619,#60620,#60621,#60622,#60623,#60624,#60625,#60626,
#60627,#60628,#60629,#60630,#60631,#60632,#60633,#60634,#60635,#60636,#60637,
#60638,#60639,#60640,#60641,#60642,#60643,#60644,#60645,#60646,#60647,#60648,
#60649,#60650,#60651,#60652,#60653,#60654,#60655,#60656,#60657,#60658,#60659,
#60660,#60661,#60662,#60663,#60664,#60665,#60666,#60667,#60668,#60669,#60670,
#60671,#60672,#60673,#60674,#60675,#60676,#60677,#60678,#60679,#60680,#60681,
#60682,#60683,#60684,#60685,#60686,#60687,#60688,#60689,#60690,#60691,#60692,
#60693,#60694,#60695,#60696,#60697,#60698),.UNSPECIFIED.,.F.,.F.,(4,3,3,
3,3,3,3,3,3,3,3,3,3,3,3,3,3,3,3,3,3,3,3,3,3,3,3,3,3,4),(-7.79281869645,
-7.67949942044,-7.42549542156316,-7.15478941327225,-6.88629582273,-6.57314502819122,
-6.43034092471,-6.03663324296969,-5.97438602668,-5.62643815484914,-5.33062385230929,
-5.06337143522,-4.81015944391811,-4.60864824296,-4.1539250507,-3.90194437733201,
-3.67105600336059,-3.46082690077013,-3.36176031805,-3.26575359933744,-3.2485926084,
-3.14531382964268,-3.0286901766774,-2.89235615658345,-2.73090076855235,
-2.60795854221919,-2.49694182442213,-2.39545292073385,-2.35004338101,-2.28525111063),
 .UNSPECIFIED.);
#1498=B_SPLINE_CURVE_WITH_KNOTS('',3,(#60700,#60701,#60702,#60703,#60704,
#60705,#60706,#60707,#60708,#60709,#60710,#60711,#60712,#60713,#60714,#60715,
#60716,#60717,#60718,#60719,#60720,#60721,#60722,#60723,#60724,#60725,#60726,
#60727,#60728,#60729,#60730,#60731,#60732,#60733,#60734,#60735,#60736,#60737,
#60738,#60739,#60740,#60741,#60742,#60743,#60744,#60745,#60746,#60747,#60748,
#60749,#60750,#60751,#60752,#60753,#60754,#60755,#60756,#60757,#60758,#60759,
#60760,#60761,#60762,#60763,#60764,#60765,#60766,#60767,#60768,#60769,#60770,
#60771,#60772,#60773,#60774,#60775,#60776,#60777,#60778,#60779,#60780,#60781,
#60782,#60783,#60784,#60785,#60786,#60787,#60788,#60789,#60790,#60791,#60792,
#60793),.UNSPECIFIED.,.F.,.F.,(4,3,3,3,3,3,3,3,3,3,3,3,3,3,3,3,3,3,3,3,
3,3,3,3,3,3,3,3,3,3,3,4),(-13.2289036984,-13.1363363987,-12.7039146576445,
-12.2656445883932,-11.8203474449897,-11.7478128989,-11.3759683318,-11.0041237647,
-10.6322757438,-10.260427723,-9.81056916950994,-9.36831267876866,-8.93752756344516,
-8.77115009928,-8.38005931279316,-8.02693833198,-7.58627963281806,-7.28260520275,
-6.91072921484,-6.72545154345561,-6.57518451173468,-6.53884477084,-6.20766710310589,
-5.85259632044063,-5.7953515875,-5.61051183579,-5.42567208408,-4.86329344259355,
-4.42659519004677,-4.04870735943222,-3.9898969375,-3.98723768815),
 .UNSPECIFIED.);
#1499=B_SPLINE_CURVE_WITH_KNOTS('',3,(#60795,#60796,#60797,#60798,#60799,
#60800,#60801,#60802,#60803,#60804,#60805,#60806,#60807,#60808,#60809,#60810,
#60811,#60812,#60813,#60814,#60815,#60816,#60817,#60818,#60819,#60820,#60821,
#60822,#60823,#60824,#60825,#60826,#60827,#60828,#60829,#60830,#60831,#60832,
#60833,#60834,#60835,#60836,#60837,#60838,#60839,#60840,#60841,#60842,#60843,
#60844,#60845,#60846,#60847,#60848,#60849,#60850,#60851,#60852,#60853,#60854,
#60855,#60856,#60857,#60858,#60859,#60860,#60861),.UNSPECIFIED.,.F.,.F.,
(4,3,3,3,3,3,3,3,3,3,3,3,3,3,3,3,3,3,3,3,3,3,4),(-2.17764450768,-2.16188924925,
-2.14608131572,-2.04937608347787,-1.95055079824093,-1.92475641533,-1.82569378496154,
-1.72535541822825,-1.66529892429,-1.56394425497464,-1.46322035284832,-1.40616268126,
-1.30612763707831,-1.20512898324395,-1.14773462447,-1.04670145974409,-0.946860935027668,
-0.88869522514,-0.791307897591113,-0.758836137641,-0.661745856495318,-0.628978582368,
-0.620875478398),.UNSPECIFIED.);
#1500=B_SPLINE_CURVE_WITH_KNOTS('',3,(#60863,#60864,#60865,#60866,#60867,
#60868,#60869,#60870,#60871,#60872,#60873,#60874,#60875,#60876,#60877,#60878,
#60879,#60880,#60881,#60882,#60883,#60884,#60885,#60886,#60887,#60888,#60889,
#60890,#60891,#60892,#60893,#60894,#60895,#60896,#60897,#60898,#60899,#60900,
#60901,#60902,#60903,#60904,#60905,#60906,#60907,#60908,#60909,#60910,#60911,
#60912,#60913,#60914,#60915,#60916,#60917,#60918,#60919,#60920,#60921,#60922,
#60923,#60924,#60925,#60926,#60927,#60928,#60929,#60930,#60931,#60932,#60933,
#60934,#60935),.UNSPECIFIED.,.F.,.F.,(4,3,3,3,3,3,3,3,3,3,3,3,3,3,3,3,3,
3,3,3,3,3,3,3,4),(-23.7990191102984,-23.5934535831,-23.1431272519468,-22.4354965963186,
-21.7218289035809,-21.0023651816132,-20.2749223320983,-19.5431341039927,
-18.807619336268,-18.0691154283988,-17.327756682932,-16.5856934993422,-15.8439026841036,
-15.565351162,-14.8278577905087,-14.0888878688926,-13.3557858843766,-12.6257415244233,
-11.8993880235048,-11.1535656220236,-10.4384244024611,-9.72763955180798,
-9.02311822061675,-8.91609841758,-8.86843301073),.UNSPECIFIED.);
#1501=B_SPLINE_CURVE_WITH_KNOTS('',3,(#60937,#60938,#60939,#60940,#60941,
#60942,#60943,#60944,#60945,#60946,#60947,#60948,#60949,#60950,#60951,#60952,
#60953,#60954,#60955,#60956,#60957,#60958,#60959,#60960,#60961,#60962,#60963,
#60964,#60965,#60966,#60967,#60968,#60969,#60970,#60971,#60972,#60973,#60974,
#60975,#60976,#60977,#60978,#60979,#60980,#60981,#60982,#60983,#60984,#60985,
#60986,#60987,#60988,#60989,#60990,#60991,#60992,#60993,#60994,#60995,#60996,
#60997,#60998,#60999,#61000,#61001,#61002,#61003,#61004,#61005,#61006,#61007,
#61008,#61009),.UNSPECIFIED.,.F.,.F.,(4,3,3,3,3,3,3,3,3,3,3,3,3,3,3,3,3,
3,3,3,3,3,3,3,4),(-23.7989336863,-23.5933107254,-23.1429840945252,-22.4353534366108,
-21.7216857415819,-21.0022220173521,-20.2747791658714,-19.5429909359402,
-18.8074761665865,-18.0689722573345,-17.3276135110272,-16.5855503268534,
-15.8437595113402,-15.5652083044,-14.8277149322353,-14.0887450106984,-13.3556430258233,
-12.625598665673,-11.8992451647312,-11.1534227635334,-10.4382815443863,
-9.7274966942919,-9.02297536384898,-8.91595555994,-8.86829015303),
 .UNSPECIFIED.);
#1502=B_SPLINE_CURVE_WITH_KNOTS('',3,(#61011,#61012,#61013,#61014,#61015,
#61016,#61017,#61018,#61019,#61020,#61021,#61022,#61023,#61024,#61025,#61026,
#61027,#61028,#61029,#61030,#61031,#61032,#61033,#61034,#61035,#61036,#61037,
#61038,#61039,#61040,#61041,#61042,#61043,#61044,#61045,#61046,#61047,#61048,
#61049,#61050,#61051,#61052,#61053,#61054,#61055,#61056,#61057,#61058,#61059,
#61060,#61061,#61062,#61063,#61064,#61065,#61066,#61067,#61068,#61069,#61070,
#61071,#61072,#61073,#61074,#61075,#61076,#61077),.UNSPECIFIED.,.F.,.F.,
(4,3,3,3,3,3,3,3,3,3,3,3,3,3,3,3,3,3,3,3,3,3,4),(-2.1776356295,-2.16188037113,
-2.1460724376,-2.04936720453685,-1.95054191829975,-1.92474753722,-1.82568490742854,
-1.7253465411801,-1.66529004618,-1.56393537591893,-1.46321147198222,-1.40615380315,
-1.3061187585445,-1.20512010447212,-1.14772574635,-1.04669258116211,-0.946852056176822,
-0.888686347023,-0.791299019961067,-0.758827259524,-0.661736983769767,-0.628969704251,
-0.620866600281),.UNSPECIFIED.);
#1503=B_SPLINE_CURVE_WITH_KNOTS('',3,(#61079,#61080,#61081,#61082,#61083,
#61084,#61085,#61086,#61087,#61088,#61089,#61090,#61091,#61092,#61093,#61094,
#61095,#61096,#61097,#61098,#61099,#61100,#61101,#61102,#61103,#61104,#61105,
#61106,#61107,#61108,#61109,#61110,#61111,#61112,#61113,#61114,#61115,#61116,
#61117,#61118,#61119,#61120,#61121,#61122,#61123,#61124,#61125,#61126,#61127,
#61128,#61129,#61130,#61131,#61132,#61133,#61134,#61135,#61136,#61137,#61138,
#61139,#61140,#61141,#61142,#61143,#61144,#61145,#61146,#61147,#61148,#61149,
#61150,#61151,#61152,#61153,#61154,#61155,#61156,#61157,#61158,#61159,#61160,
#61161,#61162,#61163,#61164,#61165,#61166,#61167,#61168,#61169,#61170,#61171,
#61172),.UNSPECIFIED.,.F.,.F.,(4,3,3,3,3,3,3,3,3,3,3,3,3,3,3,3,3,3,3,3,
3,3,3,3,3,3,3,3,3,3,3,4),(-13.2113291298,-13.1198592829,-12.7138234948033,
-12.2491997146626,-11.7479634371,-11.5635068486,-11.3790502601,-11.01025109405,
-10.6818996115644,-10.641451928,-10.4569885283,-10.2725251287,-9.89017431483876,
-9.53000452626,-9.09201113677,-8.78735838024,-8.41545051994,-8.04354265963,
-7.6036358701249,-7.14938102351304,-6.84005706681584,-6.48124957061761,
-6.15762630428405,-5.81661960069471,-5.65886522087669,-5.19480454113099,
-4.73527397296271,-4.35243553509635,-4.16101631616318,-4.05459365329759,
-3.98056776548391,-3.96959709723),.UNSPECIFIED.);
#1504=B_SPLINE_CURVE_WITH_KNOTS('',3,(#61174,#61175,#61176,#61177,#61178,
#61179,#61180,#61181,#61182,#61183,#61184,#61185,#61186,#61187,#61188,#61189,
#61190,#61191,#61192,#61193,#61194,#61195,#61196,#61197,#61198,#61199,#61200,
#61201,#61202,#61203,#61204,#61205,#61206,#61207,#61208,#61209,#61210,#61211,
#61212,#61213,#61214,#61215,#61216,#61217,#61218,#61219,#61220,#61221,#61222,
#61223,#61224,#61225,#61226,#61227,#61228,#61229,#61230,#61231,#61232,#61233,
#61234,#61235,#61236,#61237,#61238,#61239,#61240,#61241,#61242,#61243,#61244,
#61245,#61246,#61247,#61248,#61249,#61250,#61251,#61252,#61253,#61254,#61255,
#61256,#61257,#61258,#61259,#61260,#61261,#61262,#61263,#61264,#61265,#61266,
#61267,#61268,#61269,#61270),.UNSPECIFIED.,.F.,.F.,(4,3,3,3,3,3,3,3,3,3,
3,3,3,3,3,3,3,3,3,3,3,3,3,3,3,3,3,3,3,3,3,3,4),(-8.30480917216,-8.20674902705309,
-8.19221653176,-8.0877738063407,-7.97005328754931,-7.83350146987149,-7.66302190217223,
-7.53706337711518,-7.42341581646934,-7.31906007234852,-7.29528378098,-7.19860124179192,
-7.18248685409,-7.06312896319687,-6.93102711737306,-6.7599627390844,-6.61338526833548,
-6.50571033408,-6.1750621993239,-6.05323280545,-5.64559470344954,-5.60075527683,
-5.3106129931726,-4.97998265541636,-4.62489839005107,-4.23622188997,-3.91547288076966,
-3.7807289703,-3.50257938254203,-3.23689747688513,-2.9855623444676,-2.82975945536,
-2.79838908821),.UNSPECIFIED.);
#1505=B_SPLINE_CURVE_WITH_KNOTS('',3,(#61272,#61273,#61274,#61275,#61276,
#61277,#61278,#61279,#61280,#61281,#61282,#61283,#61284,#61285,#61286,#61287,
#61288,#61289,#61290,#61291,#61292,#61293,#61294,#61295,#61296,#61297,#61298,
#61299,#61300,#61301,#61302,#61303,#61304,#61305,#61306,#61307,#61308,#61309,
#61310,#61311,#61312,#61313,#61314,#61315,#61316,#61317,#61318,#61319,#61320,
#61321,#61322,#61323,#61324,#61325,#61326,#61327,#61328,#61329,#61330,#61331,
#61332,#61333,#61334,#61335,#61336,#61337,#61338,#61339,#61340,#61341,#61342,
#61343,#61344,#61345,#61346,#61347,#61348,#61349,#61350,#61351,#61352,#61353,
#61354,#61355,#61356,#61357,#61358,#61359,#61360,#61361,#61362,#61363,#61364,
#61365,#61366,#61367,#61368,#61369,#61370,#61371,#61372,#61373,#61374,#61375,
#61376,#61377,#61378,#61379,#61380,#61381,#61382,#61383,#61384,#61385,#61386,
#61387,#61388,#61389,#61390,#61391,#61392,#61393,#61394,#61395,#61396,#61397,
#61398,#61399,#61400,#61401,#61402,#61403,#61404,#61405,#61406,#61407,#61408,
#61409,#61410,#61411,#61412,#61413,#61414,#61415,#61416,#61417,#61418,#61419,
#61420,#61421,#61422,#61423,#61424,#61425,#61426,#61427,#61428,#61429,#61430,
#61431,#61432,#61433,#61434,#61435,#61436,#61437,#61438,#61439,#61440,#61441,
#61442,#61443,#61444,#61445,#61446),.UNSPECIFIED.,.F.,.F.,(4,3,3,3,3,3,
3,3,3,3,3,3,3,3,3,3,3,3,3,3,3,3,3,3,3,3,3,3,3,3,3,3,3,3,3,3,3,3,3,3,3,3,
3,3,3,3,3,3,3,3,3,3,3,3,3,3,3,3,4),(-53.5008998895,-53.3451916901284,-53.176656319643,
-52.9955204032205,-52.791135379922,-52.481916398361,-52.2794726982479,-52.1726974168,
-52.0066176910375,-51.8359554148276,-51.6537586616127,-51.4519287511538,
-51.1702440627414,-50.9427338453991,-50.8440596107,-49.9636996596638,-48.9547071229077,
-47.643973374075,-47.1169000853,-46.2401091876284,-45.0864798214665,-44.3241190945,
-42.906834582425,-41.7215633027034,-40.6182822590178,-39.6011883397494,
-38.6549810462,-37.8607076357675,-37.036273639443,-36.1743165155458,-35.2335575681182,
-34.233341794715,-33.16058908859,-32.8906058289,-32.0241966713569,-31.1105158015195,
-30.1341511136148,-29.0384970733065,-27.9400127615476,-26.9521397421388,
-26.1445609307,-25.4081132498847,-24.5844671352085,-23.8329347162207,-23.1710589742443,
-22.9473682995,-22.1867384924654,-21.3935014433163,-20.5314587518937,-19.6081583210602,
-18.6075304975,-17.5358782925033,-16.5923577579566,-16.313163739,-15.4464807336901,
-15.1660032466,-14.4038444044393,-14.0188427542,-13.30850513),
 .UNSPECIFIED.);
#1506=B_SPLINE_CURVE_WITH_KNOTS('',3,(#61449,#61450,#61451,#61452,#61453,
#61454,#61455,#61456,#61457,#61458,#61459,#61460,#61461,#61462,#61463,#61464,
#61465,#61466,#61467,#61468,#61469,#61470,#61471,#61472,#61473,#61474,#61475,
#61476,#61477,#61478,#61479,#61480,#61481,#61482,#61483,#61484,#61485,#61486,
#61487,#61488,#61489,#61490,#61491,#61492,#61493,#61494,#61495,#61496,#61497,
#61498,#61499,#61500,#61501,#61502,#61503,#61504,#61505,#61506,#61507,#61508,
#61509,#61510,#61511,#61512,#61513,#61514,#61515,#61516,#61517,#61518,#61519,
#61520,#61521,#61522,#61523,#61524,#61525,#61526,#61527,#61528,#61529,#61530,
#61531,#61532,#61533,#61534,#61535,#61536,#61537,#61538,#61539,#61540,#61541,
#61542,#61543,#61544,#61545,#61546,#61547,#61548,#61549,#61550,#61551,#61552,
#61553,#61554,#61555,#61556,#61557,#61558,#61559,#61560,#61561,#61562,#61563,
#61564,#61565,#61566,#61567,#61568,#61569,#61570,#61571,#61572,#61573,#61574,
#61575,#61576,#61577,#61578,#61579,#61580,#61581,#61582,#61583,#61584,#61585,
#61586,#61587,#61588,#61589,#61590,#61591,#61592,#61593,#61594,#61595,#61596,
#61597,#61598,#61599,#61600,#61601,#61602,#61603,#61604,#61605,#61606,#61607,
#61608,#61609,#61610,#61611,#61612,#61613,#61614,#61615,#61616,#61617,#61618,
#61619,#61620,#61621,#61622,#61623,#61624,#61625,#61626,#61627,#61628,#61629,
#61630,#61631,#61632,#61633,#61634,#61635,#61636,#61637,#61638,#61639,#61640,
#61641,#61642,#61643,#61644,#61645,#61646,#61647,#61648,#61649,#61650),
 .UNSPECIFIED.,.F.,.F.,(4,3,3,3,3,3,3,3,3,3,3,3,3,3,3,3,3,3,3,3,3,3,3,3,
3,3,3,3,3,3,3,3,3,3,3,3,3,3,3,3,3,3,3,3,3,3,3,3,3,3,3,3,3,3,3,3,3,3,3,3,
3,3,3,3,3,3,3,4),(-53.3460404053,-53.3427865087,-52.60822116117,-51.8501309764489,
-51.0468521204321,-50.5673270881,-49.6384172387309,-49.4117332356,-48.370926532647,
-48.256139383,-47.172901573675,-46.290385123257,-45.4631852964085,-44.6931867210543,
-43.9231881457,-43.1910896700299,-42.4326163740021,-41.655386537904,-40.846702077429,
-40.7712546448,-39.9111719491253,-38.9706748712524,-37.9461038688566,-37.0047521746,
-36.1296894289149,-35.1237074138,-34.1831850334,-33.3515209320406,-33.242662653,
-32.4464253978397,-31.622887139341,-30.7177557477536,-29.9241878583544,
-28.9084000075,-27.769668299622,-27.4636133133,-26.1168248606185,-25.0917528993528,
-24.5861173859,-23.0994130651888,-21.7086214585,-20.3835250606754,-19.1543842389577,
-18.8316459182,-18.3404587841209,-17.7232621803309,-17.1542493787613,-16.6759696232846,
-16.2528560288109,-15.9546703779,-15.7653246905542,-15.5401850478735,-15.3151445916,
-15.1222566797647,-14.9953808216,-14.8336231269604,-14.6756170516,-14.5309640342055,
-14.3738737358606,-14.2041627848116,-14.0359901315,-13.7860214709346,-13.6035114623165,
-13.4444369202988,-13.3963632114,-13.2512150095039,-13.2018838044,-13.1529830415),
 .UNSPECIFIED.);
#1507=B_SPLINE_CURVE_WITH_KNOTS('',3,(#61653,#61654,#61655,#61656,#61657,
#61658,#61659,#61660,#61661,#61662,#61663,#61664,#61665,#61666,#61667,#61668,
#61669,#61670,#61671,#61672,#61673,#61674,#61675,#61676,#61677,#61678,#61679,
#61680,#61681,#61682,#61683,#61684,#61685,#61686,#61687,#61688,#61689,#61690,
#61691,#61692,#61693,#61694,#61695,#61696,#61697,#61698,#61699,#61700,#61701,
#61702,#61703,#61704,#61705,#61706,#61707,#61708,#61709,#61710,#61711,#61712,
#61713,#61714,#61715,#61716,#61717,#61718,#61719,#61720,#61721,#61722,#61723,
#61724,#61725,#61726,#61727,#61728,#61729,#61730,#61731,#61732,#61733,#61734,
#61735,#61736,#61737,#61738,#61739,#61740,#61741,#61742,#61743,#61744,#61745,
#61746,#61747,#61748,#61749,#61750,#61751,#61752,#61753,#61754,#61755,#61756,
#61757,#61758,#61759,#61760,#61761,#61762,#61763,#61764,#61765,#61766,#61767,
#61768,#61769,#61770,#61771,#61772,#61773,#61774,#61775,#61776,#61777,#61778,
#61779,#61780,#61781,#61782,#61783,#61784,#61785,#61786,#61787,#61788,#61789,
#61790,#61791,#61792,#61793,#61794,#61795,#61796,#61797,#61798,#61799,#61800),
 .UNSPECIFIED.,.F.,.F.,(4,3,3,3,3,3,3,3,3,3,3,3,3,3,3,3,3,3,3,3,3,3,3,3,
3,3,3,3,3,3,3,3,3,3,3,3,3,3,3,3,3,3,3,3,3,3,3,3,3,4),(-50.0065304478,-49.9655295734,
-49.5003776209995,-48.8647346605083,-48.1990477939634,-48.0421461897,-47.3239922394653,
-46.546059887321,-45.99055442,-45.1729075981979,-44.4006897530799,-44.1193282242,
-43.4306528365354,-43.1836085783,-42.5464621396718,-42.2478889325,-41.6197270866977,
-41.0142731913314,-40.8836098595,-40.2470020031306,-39.5870400266364,-39.5193307866,
-38.8016514026391,-38.0559900546954,-37.6541457182902,-36.7245836424735,
-36.3852905632,-35.535496168716,-34.6711156567913,-33.790939725517,-32.8843725746734,
-31.9615205628221,-31.0128671534724,-30.5763255063,-29.7407127311743,-29.2329469859,
-28.3396449754151,-27.8895684656,-26.8655970551007,-25.7162996271993,-25.1653444925737,
-24.064560055184,-23.1069531953081,-22.5384104949,-21.4697437660747,-20.3631909524721,
-19.2056561621257,-17.9969487872128,-16.7882414123,-16.6199171729),
 .UNSPECIFIED.);
#1508=B_SPLINE_CURVE_WITH_KNOTS('',3,(#61802,#61803,#61804,#61805,#61806,
#61807,#61808,#61809,#61810,#61811,#61812,#61813,#61814,#61815,#61816,#61817,
#61818,#61819,#61820,#61821,#61822,#61823,#61824,#61825,#61826),
 .UNSPECIFIED.,.F.,.F.,(4,3,3,3,3,3,3,3,4),(-0.219167536337,-0.212065411498659,
-0.209869986607,-0.20125552271857,-0.189187478531417,-0.181061523730626,
-0.174173405713463,-0.169607467001,-0.167763693388021),.UNSPECIFIED.);
#1509=B_SPLINE_CURVE_WITH_KNOTS('',3,(#61828,#61829,#61830,#61831,#61832,
#61833,#61834,#61835,#61836,#61837,#61838,#61839,#61840,#61841,#61842,#61843,
#61844,#61845,#61846,#61847,#61848,#61849,#61850,#61851,#61852,#61853,#61854,
#61855,#61856,#61857,#61858,#61859,#61860,#61861,#61862,#61863,#61864,#61865,
#61866,#61867,#61868,#61869,#61870,#61871,#61872,#61873,#61874,#61875,#61876,
#61877,#61878,#61879,#61880,#61881,#61882,#61883,#61884,#61885,#61886,#61887,
#61888,#61889,#61890,#61891),.UNSPECIFIED.,.F.,.F.,(4,3,3,3,3,3,3,3,3,3,
3,3,3,3,3,3,3,3,3,3,3,4),(-4.75541642643,-4.72387222305,-4.69232801967,
-4.62924113332,-4.42053745532439,-4.25070576676,-4.03675783621436,-3.81910899772752,
-3.60004242876329,-3.38004735105967,-3.23201205664,-3.0052780124093,-2.78271542041613,
-2.72286212815,-2.50719500943497,-2.29534783281628,-2.213598844,-1.99844479337847,
-1.78837851696703,-1.66230163141,-1.62673590825417,-1.62406174599),
 .UNSPECIFIED.);
#1510=B_SPLINE_CURVE_WITH_KNOTS('',3,(#61895,#61896,#61897,#61898,#61899,
#61900,#61901,#61902,#61903,#61904,#61905,#61906,#61907,#61908,#61909,#61910,
#61911,#61912,#61913,#61914,#61915,#61916,#61917,#61918,#61919,#61920,#61921,
#61922,#61923,#61924,#61925,#61926,#61927,#61928,#61929,#61930,#61931,#61932,
#61933,#61934,#61935,#61936,#61937,#61938,#61939,#61940,#61941,#61942,#61943,
#61944,#61945,#61946),.UNSPECIFIED.,.F.,.F.,(4,3,3,3,3,3,3,3,3,3,3,3,3,
3,3,3,3,4),(-1.8860355782,-1.876230501475,-1.86804904262136,-1.86361992583938,
-1.8468152713,-1.74222710009253,-1.61996621682398,-1.57026734258,-1.43603198366343,
-1.32099299495717,-1.24895127143,-1.11387865106139,-0.97513337134255,-0.927387660673,
-0.783897981610959,-0.645270772084385,-0.605876247363,-0.591155709264),
 .UNSPECIFIED.);
#1511=B_SPLINE_CURVE_WITH_KNOTS('',3,(#61950,#61951,#61952,#61953,#61954,
#61955,#61956,#61957,#61958,#61959,#61960,#61961,#61962,#61963,#61964,#61965,
#61966,#61967,#61968,#61969,#61970,#61971,#61972,#61973,#61974,#61975,#61976,
#61977,#61978,#61979,#61980,#61981,#61982,#61983,#61984,#61985,#61986,#61987,
#61988,#61989,#61990,#61991,#61992,#61993,#61994,#61995,#61996,#61997,#61998,
#61999,#62000,#62001,#62002,#62003,#62004,#62005,#62006,#62007,#62008,#62009,
#62010,#62011,#62012,#62013,#62014,#62015,#62016,#62017,#62018,#62019,#62020,
#62021,#62022,#62023,#62024,#62025,#62026,#62027,#62028,#62029,#62030,#62031,
#62032,#62033,#62034,#62035,#62036,#62037,#62038,#62039,#62040,#62041,#62042,
#62043,#62044,#62045,#62046,#62047,#62048,#62049,#62050,#62051,#62052,#62053,
#62054,#62055,#62056,#62057,#62058,#62059,#62060,#62061,#62062,#62063,#62064,
#62065,#62066,#62067,#62068,#62069,#62070,#62071,#62072,#62073,#62074,#62075,
#62076,#62077,#62078,#62079,#62080,#62081,#62082,#62083,#62084,#62085,#62086,
#62087,#62088),.UNSPECIFIED.,.F.,.F.,(4,3,3,3,3,3,3,3,3,3,3,3,3,3,3,3,3,
3,3,3,3,3,3,3,3,3,3,3,3,3,3,3,3,3,3,3,3,3,3,3,3,3,3,3,3,3,4),(-17.8472140382,
-17.4019122389937,-17.3512488436,-16.85541857445,-16.617833683475,-16.3595883053,
-15.8637586192,-15.3045462433964,-14.7145756425834,-14.0542923973833,-13.8694359552,
-13.1009730407947,-12.8724670748,-12.2295685253444,-11.8754981945,-11.3790035319467,
-10.8840856317586,-10.3876429994243,-9.89120036709,-9.44497083276126,-9.01864480463145,
-8.655041284792,-8.46312097464113,-8.23964753863528,-7.99371675369271,-7.79717014573183,
-7.61881001009051,-7.45488131018598,-7.41888220249,-7.30472285597012,-7.29472016445,
-7.17409590447506,-7.04405617254464,-6.92223811653,-6.75802974895856,-6.55073660565142,
-6.40541579054849,-6.27111933005145,-6.14490398563562,-6.02723969347144,
-5.92885717573,-5.6476534049758,-5.35705149846824,-5.06034757923729,-4.75273035291205,
-4.57652678804,-4.57396017214),.UNSPECIFIED.);
#1512=B_SPLINE_CURVE_WITH_KNOTS('',3,(#62090,#62091,#62092,#62093,#62094,
#62095,#62096,#62097,#62098,#62099,#62100,#62101,#62102,#62103,#62104,#62105,
#62106,#62107,#62108,#62109,#62110,#62111,#62112,#62113,#62114,#62115,#62116,
#62117,#62118,#62119,#62120,#62121,#62122,#62123,#62124,#62125,#62126,#62127,
#62128,#62129,#62130,#62131,#62132,#62133,#62134,#62135,#62136,#62137,#62138,
#62139,#62140,#62141,#62142,#62143,#62144,#62145,#62146,#62147,#62148,#62149,
#62150,#62151,#62152,#62153,#62154,#62155,#62156,#62157,#62158,#62159,#62160,
#62161,#62162,#62163,#62164,#62165,#62166,#62167,#62168,#62169,#62170,#62171,
#62172,#62173,#62174,#62175,#62176,#62177,#62178,#62179,#62180,#62181,#62182,
#62183,#62184,#62185,#62186,#62187,#62188,#62189,#62190,#62191,#62192,#62193,
#62194,#62195,#62196,#62197,#62198,#62199,#62200,#62201,#62202,#62203,#62204,
#62205,#62206,#62207,#62208,#62209,#62210),.UNSPECIFIED.,.F.,.F.,(4,3,3,
3,3,3,3,3,3,3,3,3,3,3,3,3,3,3,3,3,3,3,3,3,3,3,3,3,3,3,3,3,3,3,3,3,3,3,3,
3,4),(-11.0890194561,-11.0060465091,-10.7571297503,-10.4223140055137,-10.0919171230019,
-9.76152024049,-9.427862963425,-9.09420568636,-8.76054366777,-8.59369978828,
-8.31461399497201,-8.04536355520786,-7.74133423580622,-7.55484692789209,
-7.42492523466838,-7.15925778640574,-6.90041903467715,-6.65046230229727,
-6.61192064383,-6.37656580563646,-6.15243841672,-5.91416092316544,-5.71470268512104,
-5.50378059751066,-5.33165972275241,-5.05173215616808,-4.92630401996643,
-4.65681431069814,-4.42074635735337,-4.33579570846539,-4.28137345509732,
-4.01455173363582,-3.75409956920042,-3.61454292872757,-3.48132690504573,
-3.23632060463136,-3.00229564428568,-2.88528316411284,-2.82677692402642,
-2.78998865932871,-2.76827068394),.UNSPECIFIED.);
#1513=B_SPLINE_CURVE_WITH_KNOTS('',3,(#62211,#62212,#62213,#62214,#62215,
#62216,#62217,#62218,#62219,#62220,#62221,#62222,#62223,#62224,#62225,#62226,
#62227,#62228,#62229,#62230,#62231,#62232,#62233,#62234,#62235,#62236,#62237,
#62238,#62239,#62240,#62241,#62242,#62243,#62244,#62245,#62246,#62247,#62248,
#62249,#62250,#62251,#62252,#62253,#62254,#62255,#62256,#62257,#62258,#62259,
#62260,#62261,#62262,#62263,#62264,#62265,#62266,#62267,#62268,#62269,#62270,
#62271),.UNSPECIFIED.,.F.,.F.,(4,3,3,3,3,3,3,3,3,3,3,3,3,3,3,3,3,3,3,3,
4),(-7.40337618611,-7.30024117289,-7.06600961895104,-6.8209088492883,-6.57835249804,
-6.30332631195281,-6.16026200237,-5.95121247231,-5.74216294226,-5.32460317331,
-5.11582036754,-4.90703756176,-4.604432666243,-4.31203427436253,-4.07794185412,
-3.80052244048256,-3.53509974462071,-3.27566898601775,-3.02440731543462,
-2.85217897174,-2.81287993679),.UNSPECIFIED.);
#1514=B_SPLINE_CURVE_WITH_KNOTS('',3,(#62274,#62275,#62276,#62277,#62278,
#62279,#62280,#62281,#62282,#62283,#62284,#62285,#62286,#62287,#62288,#62289,
#62290,#62291,#62292,#62293,#62294,#62295,#62296,#62297,#62298,#62299,#62300,
#62301,#62302,#62303,#62304,#62305,#62306,#62307,#62308,#62309,#62310,#62311,
#62312,#62313,#62314,#62315,#62316,#62317,#62318,#62319,#62320,#62321,#62322,
#62323,#62324,#62325,#62326,#62327,#62328,#62329,#62330,#62331,#62332,#62333,
#62334,#62335,#62336,#62337,#62338,#62339,#62340,#62341,#62342,#62343,#62344,
#62345,#62346,#62347,#62348,#62349,#62350,#62351,#62352,#62353,#62354,#62355,
#62356,#62357,#62358,#62359,#62360,#62361,#62362,#62363,#62364,#62365,#62366,
#62367,#62368,#62369,#62370,#62371,#62372,#62373,#62374,#62375,#62376,#62377,
#62378,#62379,#62380,#62381,#62382,#62383,#62384,#62385,#62386,#62387,#62388,
#62389,#62390,#62391,#62392,#62393,#62394,#62395,#62396,#62397,#62398,#62399,
#62400,#62401,#62402,#62403,#62404,#62405,#62406,#62407,#62408,#62409,#62410,
#62411,#62412,#62413,#62414,#62415,#62416,#62417,#62418,#62419,#62420,#62421),
 .UNSPECIFIED.,.F.,.F.,(4,3,3,3,3,3,3,3,3,3,3,3,3,3,3,3,3,3,3,3,3,3,3,3,
3,3,3,3,3,3,3,3,3,3,3,3,3,3,3,3,3,3,3,3,3,3,3,3,3,4),(-45.9550550567,-45.8547536634,
-44.7020593272519,-43.5325678037029,-42.3148462029271,-41.1424810446725,
-39.9829249214987,-38.8482537160837,-38.6616814006,-37.5789809595078,-36.3892933779578,
-35.390340457305,-34.4176032593006,-33.9967366188,-33.2716301060854,-32.8656396299714,
-32.4709155643619,-31.6730674084549,-30.882094563278,-30.0838824149726,
-29.3112279304,-28.6030919404868,-27.8382957062825,-27.5205007441,-26.6765064815491,
-25.7297735578,-24.8877396119559,-24.1080276682368,-23.373256104667,-22.6847835942949,
-22.4385878762,-21.77434035765,-21.156822041211,-21.1100928391,-20.4962895824888,
-19.8596314448538,-19.7815978021,-19.117834960177,-18.8458744432,-18.1322011061612,
-17.9101510843,-17.10894748536,-16.2880919017683,-16.0388958217,-15.2857278860319,
-14.5701591557272,-13.8937803934636,-13.2174016312,-12.7652853193346,-12.5665153309),
 .UNSPECIFIED.);
#1515=B_SPLINE_CURVE_WITH_KNOTS('',3,(#62423,#62424,#62425,#62426,#62427,
#62428,#62429,#62430,#62431,#62432,#62433,#62434,#62435,#62436,#62437,#62438,
#62439,#62440,#62441,#62442,#62443,#62444,#62445,#62446,#62447,#62448,#62449,
#62450,#62451,#62452,#62453,#62454,#62455,#62456,#62457,#62458,#62459,#62460,
#62461,#62462,#62463,#62464,#62465,#62466,#62467,#62468,#62469,#62470,#62471,
#62472,#62473,#62474,#62475,#62476,#62477),.UNSPECIFIED.,.F.,.F.,(4,3,3,
3,3,3,3,3,3,3,3,3,3,3,3,3,3,3,4),(-6.6978412202,-6.44998928167263,-6.19272717356715,
-5.92880591063826,-5.65745311051901,-5.37791579855118,-5.08570414740713,
-4.78670366790336,-4.48187066288165,-4.45303700515737,-4.02197464488505,
-3.67567871029374,-3.3757846822016,-3.09960655669372,-2.84547660754957,
-2.5999707008135,-2.35368976040675,-2.12340855147386,-2.10740882),
 .UNSPECIFIED.);
#1516=B_SPLINE_CURVE_WITH_KNOTS('',3,(#62479,#62480,#62481,#62482,#62483,
#62484,#62485,#62486,#62487,#62488,#62489,#62490,#62491,#62492,#62493,#62494,
#62495,#62496,#62497,#62498,#62499,#62500,#62501,#62502,#62503,#62504,#62505,
#62506,#62507,#62508,#62509,#62510,#62511,#62512,#62513,#62514,#62515,#62516,
#62517,#62518,#62519,#62520,#62521,#62522,#62523,#62524,#62525,#62526,#62527,
#62528,#62529,#62530,#62531,#62532,#62533,#62534,#62535,#62536,#62537,#62538,
#62539,#62540,#62541,#62542,#62543,#62544,#62545,#62546,#62547,#62548,#62549,
#62550,#62551,#62552,#62553,#62554,#62555,#62556,#62557,#62558,#62559,#62560,
#62561,#62562,#62563,#62564,#62565,#62566,#62567,#62568,#62569,#62570,#62571,
#62572,#62573,#62574,#62575,#62576,#62577,#62578,#62579,#62580,#62581,#62582,
#62583,#62584,#62585,#62586,#62587,#62588,#62589,#62590,#62591,#62592,#62593,
#62594,#62595,#62596,#62597,#62598,#62599,#62600,#62601,#62602,#62603,#62604,
#62605,#62606,#62607,#62608),.UNSPECIFIED.,.F.,.F.,(4,3,3,3,3,3,3,3,3,3,
3,3,3,3,3,3,3,3,3,3,3,3,3,3,3,3,3,3,3,3,3,3,3,3,3,3,3,3,3,3,3,3,3,4),(-12.1812673196,
-12.1019545715,-11.8530258523618,-11.595215506703,-11.5467858158,-11.3881500798,
-11.2295143438,-10.9699907679588,-10.9122488687,-10.7483463587,-10.5844438487,
-10.3384514976169,-10.2566501431,-10.0043239978651,-9.92881869084,-9.70732206868687,
-9.60098723862,-9.35831838515441,-9.14889513515,-8.93472094875681,-8.77284717678668,
-8.52420937980639,-8.28078037155647,-8.0453638509211,-7.82018311353108,
-7.77935654812,-7.52877970908887,-7.32110317374,-7.09200006145,-6.86289694915,
-6.5945495418842,-6.5210581838,-6.3501250021,-6.17919182041,-5.92442927962418,
-5.68485033386412,-5.49553262739,-5.20623148246893,-4.89872891457204,-4.82510489389,
-4.47179454085463,-4.15468159222,-3.87676906882,-3.85983652914),
 .UNSPECIFIED.);
#1517=B_SPLINE_CURVE_WITH_KNOTS('',3,(#62610,#62611,#62612,#62613,#62614,
#62615,#62616,#62617,#62618,#62619,#62620,#62621,#62622,#62623,#62624,#62625,
#62626,#62627,#62628,#62629,#62630,#62631,#62632,#62633,#62634,#62635,#62636,
#62637,#62638,#62639,#62640,#62641,#62642,#62643,#62644,#62645,#62646,#62647,
#62648,#62649,#62650,#62651,#62652,#62653,#62654,#62655,#62656,#62657,#62658,
#62659,#62660,#62661,#62662,#62663,#62664,#62665,#62666,#62667,#62668,#62669,
#62670,#62671,#62672,#62673,#62674,#62675,#62676,#62677,#62678,#62679,#62680,
#62681,#62682,#62683,#62684,#62685,#62686,#62687,#62688,#62689,#62690,#62691,
#62692,#62693,#62694,#62695,#62696,#62697,#62698,#62699,#62700,#62701,#62702,
#62703,#62704,#62705,#62706,#62707,#62708,#62709,#62710,#62711,#62712,#62713,
#62714,#62715,#62716,#62717,#62718,#62719,#62720,#62721,#62722,#62723,#62724,
#62725,#62726,#62727,#62728,#62729,#62730,#62731,#62732,#62733,#62734,#62735,
#62736,#62737,#62738,#62739,#62740,#62741,#62742,#62743,#62744,#62745,#62746,
#62747,#62748,#62749,#62750,#62751,#62752,#62753,#62754,#62755,#62756,#62757,
#62758,#62759,#62760),.UNSPECIFIED.,.F.,.F.,(4,3,3,3,3,3,3,3,3,3,3,3,3,
3,3,3,3,3,3,3,3,3,3,3,3,3,3,3,3,3,3,3,3,3,3,3,3,3,3,3,3,3,3,3,3,3,3,3,3,
3,4),(-17.2738332784,-17.0284868112151,-16.8153093983,-16.5064930943126,
-16.356669586,-16.0797319308535,-16.0127475115,-15.8981054324,-15.7808445708218,
-15.6585553960829,-15.5249349056484,-15.4395469722,-15.2698932931606,-15.062957071932,
-14.9385147756961,-14.8086216270683,-14.6940263327,-14.5760460181375,-14.5697715428,
-14.4565193782305,-14.4455167529,-14.291815073997,-14.1246199657078,-13.9241091491007,
-13.6878176035504,-13.5130680616142,-13.451526058,-13.0514035156419,-12.6195129795619,
-12.1624081206357,-11.6511703139133,-11.4721831186,-10.9335785602832,-10.3632144505192,
-9.74590695598728,-9.46909727915927,-8.78704121090936,-8.42694683890191,
-7.82822785856962,-7.52764856036114,-7.21067457575859,-6.62584211706413,
-6.0788387154238,-5.56229121985785,-5.4010635343667,-5.05395983406502,-4.84584110817332,
-4.42924492066666,-4.19245652259199,-4.01264873316,-4.00115394842),
 .UNSPECIFIED.);
#1518=B_SPLINE_CURVE_WITH_KNOTS('',3,(#62764,#62765,#62766,#62767,#62768,
#62769,#62770,#62771,#62772,#62773,#62774,#62775,#62776,#62777,#62778,#62779,
#62780,#62781,#62782,#62783,#62784,#62785,#62786,#62787,#62788,#62789,#62790,
#62791,#62792,#62793,#62794,#62795,#62796,#62797,#62798,#62799,#62800,#62801,
#62802,#62803,#62804,#62805,#62806,#62807,#62808,#62809),.UNSPECIFIED.,
 .F.,.F.,(4,3,3,3,3,3,3,3,3,3,3,3,3,3,3,4),(-1.88603455695,-1.86656727617,
-1.84681424904,-1.74222598447339,-1.61996499915831,-1.57026632032,-1.43603095182559,
-1.32099188319155,-1.24895024918,-1.1138776438742,-0.975132380159264,-0.927386638419,
-0.783896961730633,-0.645269714782231,-0.605875225111,-0.591154687012),
 .UNSPECIFIED.);
#1519=B_SPLINE_CURVE_WITH_KNOTS('',3,(#62813,#62814,#62815,#62816,#62817,
#62818,#62819,#62820,#62821,#62822,#62823,#62824,#62825,#62826,#62827,#62828,
#62829,#62830,#62831,#62832,#62833,#62834,#62835,#62836,#62837,#62838,#62839,
#62840,#62841,#62842,#62843,#62844,#62845,#62846,#62847,#62848,#62849,#62850,
#62851,#62852,#62853,#62854,#62855,#62856,#62857,#62858,#62859,#62860,#62861),
 .UNSPECIFIED.,.F.,.F.,(4,3,3,3,3,3,3,3,3,3,3,3,3,3,3,3,4),(-4.75656395656,
-4.60537498785813,-4.44818787789036,-4.27889046442468,-4.09863038425973,
-3.90212119682302,-3.66090058334715,-3.44155265372639,-3.23422551625958,
-2.97612342370908,-2.73021565496724,-2.49737898001046,-2.27933643879784,
-2.07018074570911,-1.86716482720178,-1.67150310968067,-1.62520881516),
 .UNSPECIFIED.);
#1520=B_SPLINE_CURVE_WITH_KNOTS('',3,(#62862,#62863,#62864,#62865,#62866,
#62867,#62868,#62869,#62870,#62871,#62872,#62873,#62874,#62875,#62876,#62877,
#62878,#62879,#62880,#62881,#62882,#62883,#62884,#62885,#62886),
 .UNSPECIFIED.,.F.,.F.,(4,3,3,3,3,3,3,3,4),(-0.219167536347,-0.212059197014113,
-0.209869986617,-0.201255522705921,-0.189187478425977,-0.181061523597616,
-0.1741734055503,-0.169607467011,-0.167763693398),.UNSPECIFIED.);
#1521=B_SPLINE_CURVE_WITH_KNOTS('',3,(#62889,#62890,#62891,#62892,#62893,
#62894,#62895,#62896,#62897,#62898,#62899,#62900,#62901,#62902,#62903,#62904,
#62905,#62906,#62907,#62908,#62909,#62910,#62911,#62912,#62913,#62914,#62915,
#62916,#62917,#62918,#62919,#62920,#62921,#62922,#62923,#62924,#62925,#62926,
#62927,#62928,#62929,#62930,#62931,#62932,#62933,#62934,#62935,#62936,#62937,
#62938,#62939,#62940,#62941,#62942,#62943,#62944,#62945,#62946,#62947,#62948,
#62949),.UNSPECIFIED.,.F.,.F.,(4,3,3,3,3,3,3,3,3,3,3,3,3,3,3,3,3,3,3,3,
4),(-18.3856123466,-18.3693186027,-17.7338457042873,-17.0822042289639,-16.4332948516141,
-15.7797891975128,-15.1220801611204,-14.4588486872985,-13.7932558597198,
-13.1250205669124,-12.5207139017,-11.8522076648893,-11.186292378156,-10.5231984210845,
-9.86372444518384,-9.20853401660924,-8.56222676146939,-7.91873801115672,
-7.27898147126907,-6.70655190271,-6.65611545055),.UNSPECIFIED.);
#1522=B_SPLINE_CURVE_WITH_KNOTS('',3,(#62951,#62952,#62953,#62954,#62955,
#62956,#62957,#62958,#62959,#62960,#62961,#62962,#62963,#62964,#62965,#62966,
#62967,#62968,#62969,#62970,#62971,#62972,#62973,#62974,#62975,#62976,#62977,
#62978,#62979,#62980,#62981,#62982,#62983,#62984,#62985,#62986,#62987,#62988,
#62989,#62990,#62991,#62992,#62993,#62994,#62995,#62996,#62997,#62998,#62999,
#63000,#63001,#63002,#63003,#63004,#63005,#63006,#63007,#63008,#63009,#63010,
#63011,#63012,#63013,#63014,#63015,#63016,#63017,#63018,#63019,#63020,#63021,
#63022,#63023,#63024,#63025,#63026,#63027,#63028,#63029,#63030,#63031,#63032,
#63033,#63034,#63035),.UNSPECIFIED.,.F.,.F.,(4,3,3,3,3,3,3,3,3,3,3,3,3,
3,3,3,3,3,3,3,3,3,3,3,3,3,3,3,4),(-12.1666998724,-11.9786962562,-11.6376009588191,
-11.2884914068467,-10.9310276199667,-10.6143846100047,-10.2318786454351,
-9.83665601387961,-9.42660550414306,-9.04238206530011,-8.59483084924109,
-8.1272682464219,-7.99998279071,-7.62059092272,-7.09680652253779,-6.64956410247717,
-6.25094224690215,-6.12491227162,-5.755282141945,-5.38565201227,-5.05920014817189,
-5.01602130474,-4.68257909391951,-4.6463905972,-4.33332998029539,-4.02503376786804,
-3.72192456507751,-3.66177393989,-3.60712399577),.UNSPECIFIED.);
#1523=B_SPLINE_CURVE_WITH_KNOTS('',3,(#63037,#63038,#63039,#63040,#63041,
#63042,#63043,#63044,#63045,#63046,#63047,#63048,#63049,#63050,#63051,#63052,
#63053,#63054,#63055,#63056,#63057,#63058,#63059,#63060,#63061,#63062,#63063,
#63064,#63065,#63066,#63067,#63068,#63069,#63070,#63071,#63072,#63073,#63074,
#63075,#63076,#63077,#63078,#63079,#63080,#63081,#63082,#63083,#63084,#63085,
#63086,#63087,#63088,#63089,#63090,#63091,#63092,#63093,#63094,#63095,#63096,
#63097,#63098,#63099,#63100,#63101,#63102,#63103,#63104,#63105,#63106,#63107,
#63108,#63109,#63110,#63111,#63112,#63113,#63114,#63115,#63116,#63117,#63118,
#63119,#63120,#63121,#63122,#63123,#63124,#63125,#63126,#63127,#63128,#63129,
#63130,#63131,#63132,#63133,#63134,#63135,#63136),.UNSPECIFIED.,.F.,.F.,
(4,3,3,3,3,3,3,3,3,3,3,3,3,3,3,3,3,3,3,3,3,3,3,3,3,3,3,3,3,3,3,3,3,4),(-17.772416875,
-17.521901514,-16.9335100063655,-16.3509832344328,-15.8162251865757,-15.7684564625,
-15.2647792762872,-14.769293572,-14.2697121268,-13.7701306816,-13.3014442440585,
-12.8657319415181,-12.7684045275,-12.3622943776427,-11.9768947679633,-11.7666783733,
-11.3217875172379,-10.877298655069,-10.7536322473,-10.3070868714199,-9.86925366913895,
-9.57637209730375,-9.14940821210187,-8.7224443269,-8.27106751604139,-7.79254976980533,
-7.70430253262,-7.19083078178567,-6.67906896927376,-6.18723057296208,-5.70660978985604,
-5.26270778945018,-5.22598900675,-5.19541482867),.UNSPECIFIED.);
#1524=B_SPLINE_CURVE_WITH_KNOTS('',3,(#63140,#63141,#63142,#63143,#63144,
#63145,#63146,#63147,#63148,#63149,#63150,#63151,#63152,#63153,#63154,#63155,
#63156,#63157,#63158,#63159,#63160,#63161,#63162,#63163,#63164,#63165,#63166,
#63167,#63168,#63169,#63170,#63171,#63172,#63173,#63174,#63175,#63176,#63177,
#63178,#63179,#63180,#63181,#63182,#63183,#63184,#63185,#63186,#63187,#63188,
#63189,#63190,#63191,#63192,#63193,#63194,#63195,#63196,#63197,#63198,#63199,
#63200,#63201,#63202,#63203,#63204,#63205,#63206,#63207,#63208,#63209,#63210,
#63211,#63212,#63213,#63214,#63215,#63216,#63217,#63218,#63219,#63220,#63221,
#63222,#63223,#63224,#63225,#63226,#63227,#63228,#63229,#63230,#63231,#63232,
#63233,#63234,#63235,#63236,#63237,#63238,#63239,#63240,#63241,#63242,#63243,
#63244,#63245),.UNSPECIFIED.,.F.,.F.,(4,3,3,3,3,3,3,3,3,3,3,3,3,3,3,3,3,
3,3,3,3,3,3,3,3,3,3,3,3,3,3,3,3,3,3,4),(-17.7593366521,-17.5082731747,-16.9919472481348,
-16.4599835808025,-15.9500345616009,-15.750791364,-15.2946015506613,-15.2446202854,
-14.8078388781449,-14.7384492068,-14.3057136278889,-13.8694237050522,-13.5442762157924,
-13.0972971028135,-12.7083210147,-12.2538973274484,-11.7931711149994,-11.6904556298,
-11.2764473929467,-10.8492913402097,-10.6739061369,-10.2365832725764,-10.1657133659,
-9.70970896481276,-9.6575205949,-9.1553358953925,-8.66383335866873,-8.15630757776936,
-7.67795613911451,-7.64878179687,-7.201975613066,-6.72017928606396,-6.1376841854597,
-5.40983099502471,-5.2053512509,-5.18156607379),.UNSPECIFIED.);
#1525=B_SPLINE_CURVE_WITH_KNOTS('',3,(#63247,#63248,#63249,#63250,#63251,
#63252,#63253,#63254,#63255,#63256,#63257,#63258,#63259,#63260,#63261,#63262,
#63263,#63264,#63265,#63266,#63267,#63268,#63269,#63270,#63271,#63272,#63273,
#63274,#63275,#63276,#63277,#63278,#63279,#63280,#63281,#63282,#63283,#63284,
#63285,#63286,#63287,#63288,#63289,#63290,#63291,#63292,#63293,#63294,#63295,
#63296,#63297,#63298,#63299,#63300,#63301,#63302,#63303,#63304,#63305,#63306,
#63307,#63308,#63309,#63310,#63311,#63312,#63313,#63314,#63315,#63316,#63317,
#63318,#63319,#63320,#63321,#63322,#63323,#63324,#63325,#63326,#63327,#63328,
#63329,#63330,#63331),.UNSPECIFIED.,.F.,.F.,(4,3,3,3,3,3,3,3,3,3,3,3,3,
3,3,3,3,3,3,3,3,3,3,3,3,3,3,3,4),(-13.8219121669,-13.5096825236108,-13.1998941240071,
-13.0694393691,-12.7498970842646,-12.4138466225267,-12.3169687025,-11.9842110392268,
-11.947857022,-11.5876140439936,-11.1992238939162,-10.7885323398095,-10.3216400674985,
-10.0989759692,-9.74353972606138,-9.48049443113105,-9.35737491835,-8.89583258585393,
-8.44881248962697,-8.02059283816397,-7.65521955896336,-7.26572917138508,
-6.88685706126507,-6.52131822386237,-6.33411128744,-5.98413683665983,-5.63575530097992,
-5.2873737653,-5.26262328413),.UNSPECIFIED.);
#1526=B_SPLINE_CURVE_WITH_KNOTS('',3,(#63332,#63333,#63334,#63335,#63336,
#63337,#63338,#63339,#63340,#63341,#63342,#63343,#63344,#63345,#63346,#63347,
#63348,#63349,#63350,#63351,#63352,#63353,#63354,#63355,#63356,#63357,#63358,
#63359,#63360,#63361,#63362,#63363,#63364,#63365,#63366,#63367,#63368,#63369,
#63370,#63371,#63372,#63373,#63374,#63375,#63376,#63377,#63378,#63379,#63380,
#63381,#63382,#63383,#63384,#63385,#63386,#63387,#63388,#63389,#63390,#63391,
#63392,#63393,#63394,#63395),.UNSPECIFIED.,.F.,.F.,(4,3,3,3,3,3,3,3,3,3,
3,3,3,3,3,3,3,3,3,3,3,4),(-18.3857494183,-18.1972119365,-18.0086744547,
-17.3704664943546,-16.7238562601433,-16.0724620532357,-15.4166996629135,
-14.7571067950976,-14.0929948370157,-13.4271604823992,-12.759986367352,
-12.3414051375,-11.6749604882608,-11.0099790390611,-10.3474170882745,-9.69024646845821,
-9.0367567914914,-8.39006781004132,-7.80407100094,-7.16502682994695,-6.66450349292,
-6.65635355468),.UNSPECIFIED.);
#1527=B_SPLINE_CURVE_WITH_KNOTS('',5,(#63609,#63610,#63611,#63612,#63613,
#63614,#63615,#63616,#63617,#63618,#63619,#63620,#63621,#63622,#63623,#63624,
#63625,#63626,#63627,#63628,#63629,#63630,#63631,#63632),.UNSPECIFIED.,
 .F.,.F.,(6,3,3,3,3,3,3,6),(0.,0.299762031377268,0.399460137024488,0.599691962356381,
0.726180908574686,0.807749761233441,0.889364957609916,1.),.UNSPECIFIED.);
#1528=B_SPLINE_CURVE_WITH_KNOTS('',3,(#63742,#63743,#63744,#63745,#63746,
#63747,#63748,#63749,#63750,#63751,#63752,#63753,#63754,#63755,#63756,#63757,
#63758,#63759,#63760,#63761,#63762,#63763,#63764,#63765,#63766,#63767,#63768,
#63769,#63770,#63771,#63772,#63773,#63774,#63775,#63776,#63777,#63778,#63779,
#63780,#63781,#63782,#63783,#63784,#63785,#63786,#63787,#63788,#63789,#63790,
#63791,#63792,#63793,#63794,#63795,#63796,#63797,#63798,#63799,#63800,#63801,
#63802,#63803,#63804,#63805,#63806,#63807,#63808,#63809,#63810,#63811,#63812,
#63813,#63814,#63815,#63816,#63817,#63818,#63819,#63820,#63821,#63822,#63823,
#63824,#63825,#63826,#63827,#63828,#63829,#63830,#63831,#63832,#63833,#63834,
#63835,#63836,#63837,#63838,#63839,#63840,#63841,#63842,#63843,#63844,#63845,
#63846,#63847,#63848,#63849,#63850,#63851,#63852,#63853,#63854,#63855,#63856,
#63857,#63858,#63859,#63860,#63861,#63862),.UNSPECIFIED.,.F.,.F.,(4,3,3,
3,3,3,3,3,3,3,3,3,3,3,3,3,3,3,3,3,3,3,3,3,3,3,3,3,3,3,3,3,3,3,3,3,3,3,3,
3,4),(0.,0.0316491751799897,0.0644683257425834,0.0985610461306416,0.134311793025957,
0.170399730229745,0.205743665747598,0.218439432092452,0.251442448401237,
0.291135045136278,0.324645711313536,0.355072767560426,0.358156377490794,
0.379293093761737,0.401196822338476,0.423985190632843,0.448171791950287,
0.473330505996812,0.498489220043337,0.520893370580924,0.544960444527389,
0.572101005410302,0.607462237305133,0.635947079645968,0.660729829937284,
0.682872356055211,0.704075903055738,0.724132541297263,0.744116466956529,
0.763570020027455,0.783812927173851,0.805062568839786,0.827656963226342,
0.853256235792581,0.880748557974103,0.907061466221659,0.930296099666244,
0.951950159507354,0.972658108974692,0.992320363498428,1.),.UNSPECIFIED.);
#1529=B_SPLINE_CURVE_WITH_KNOTS('',3,(#63969,#63970,#63971,#63972,#63973,
#63974,#63975,#63976,#63977,#63978,#63979,#63980,#63981,#63982,#63983,#63984,
#63985,#63986,#63987,#63988,#63989,#63990,#63991,#63992,#63993,#63994,#63995,
#63996,#63997,#63998,#63999,#64000,#64001,#64002,#64003,#64004,#64005,#64006,
#64007,#64008,#64009,#64010,#64011,#64012,#64013,#64014,#64015,#64016,#64017,
#64018,#64019,#64020,#64021,#64022,#64023),.UNSPECIFIED.,.F.,.F.,(4,3,3,
3,3,3,3,3,3,3,3,3,3,3,3,3,3,3,4),(0.,0.0611230585579808,0.124208925935708,
0.189652312423783,0.257713177850023,0.329796007159683,0.403624985796396,
0.477235323463936,0.488984468463847,0.510783466323955,0.599511866779462,
0.649572883432029,0.68078334097055,0.70173765692144,0.766971446251283,0.826706349016451,
0.884578246708151,0.942289123354076,1.),.UNSPECIFIED.);
#1530=B_SPLINE_CURVE_WITH_KNOTS('',5,(#64079,#64080,#64081,#64082,#64083,
#64084,#64085,#64086,#64087),.UNSPECIFIED.,.F.,.F.,(6,3,6),(0.,0.489018048130324,
1.),.UNSPECIFIED.);
#1531=B_SPLINE_CURVE_WITH_KNOTS('',3,(#64206,#64207,#64208,#64209,#64210,
#64211,#64212,#64213,#64214,#64215,#64216,#64217,#64218,#64219,#64220,#64221,
#64222,#64223,#64224,#64225,#64226,#64227,#64228,#64229,#64230,#64231,#64232,
#64233,#64234,#64235,#64236,#64237,#64238,#64239,#64240,#64241,#64242,#64243,
#64244,#64245,#64246,#64247,#64248,#64249,#64250,#64251,#64252,#64253,#64254,
#64255,#64256,#64257,#64258,#64259,#64260,#64261,#64262,#64263,#64264,#64265,
#64266,#64267,#64268,#64269,#64270,#64271,#64272,#64273,#64274,#64275,#64276,
#64277,#64278,#64279,#64280,#64281,#64282,#64283,#64284,#64285,#64286,#64287,
#64288,#64289,#64290,#64291,#64292,#64293,#64294,#64295,#64296,#64297,#64298,
#64299,#64300,#64301,#64302,#64303,#64304,#64305,#64306,#64307,#64308,#64309,
#64310,#64311,#64312,#64313,#64314),.UNSPECIFIED.,.F.,.F.,(4,3,3,3,3,3,
3,3,3,3,3,3,3,3,3,3,3,3,3,3,3,3,3,3,3,3,3,3,3,3,3,3,3,3,3,3,4),(0.,0.0346594543148337,
0.0696322066276516,0.0841787945508995,0.0941200626265949,0.101073116311595,
0.137518372591484,0.17245768807328,0.187690795924043,0.194591671799185,
0.230121129603681,0.263342933978537,0.27727563451867,0.295578236300883,
0.326545626280591,0.358345791467322,0.38118335794188,0.396975714575019,
0.42810993272217,0.458556467545967,0.487764180987173,0.511542683647487,
0.542606600917642,0.575567103336426,0.595309845990461,0.607159733636498,
0.642553986747648,0.676581605738495,0.6997079850505,0.717658166536222,0.748736746081099,
0.790711506309299,0.833723477279877,0.877063043691384,0.919856548091253,
0.960986423575859,1.),.UNSPECIFIED.);
#1532=B_SPLINE_CURVE_WITH_KNOTS('',5,(#64406,#64407,#64408,#64409,#64410,
#64411,#64412,#64413,#64414,#64415,#64416,#64417,#64418,#64419,#64420),
 .UNSPECIFIED.,.F.,.F.,(6,3,3,3,6),(0.,0.270680449730146,0.52898484435231,
0.803435714429636,1.),.UNSPECIFIED.);
#1533=B_SPLINE_CURVE_WITH_KNOTS('',3,(#64617,#64618,#64619,#64620,#64621,
#64622,#64623,#64624,#64625,#64626,#64627,#64628,#64629,#64630,#64631,#64632,
#64633,#64634,#64635,#64636,#64637,#64638,#64639,#64640,#64641,#64642,#64643,
#64644,#64645,#64646,#64647,#64648,#64649,#64650,#64651,#64652,#64653,#64654,
#64655,#64656,#64657,#64658,#64659,#64660,#64661,#64662,#64663,#64664,#64665,
#64666,#64667,#64668,#64669,#64670,#64671,#64672,#64673,#64674,#64675,#64676,
#64677,#64678,#64679,#64680,#64681,#64682,#64683,#64684,#64685,#64686,#64687,
#64688,#64689,#64690,#64691,#64692,#64693,#64694,#64695,#64696,#64697,#64698,
#64699,#64700,#64701,#64702,#64703,#64704,#64705,#64706,#64707,#64708,#64709,
#64710,#64711,#64712,#64713,#64714,#64715,#64716,#64717,#64718,#64719,#64720,
#64721,#64722,#64723,#64724,#64725,#64726,#64727,#64728,#64729,#64730,#64731,
#64732,#64733,#64734,#64735,#64736,#64737,#64738,#64739,#64740,#64741,#64742,
#64743,#64744,#64745,#64746,#64747,#64748,#64749,#64750,#64751,#64752),
 .UNSPECIFIED.,.F.,.F.,(4,3,3,3,3,3,3,3,3,3,3,3,3,3,3,3,3,3,3,3,3,3,3,3,
3,3,3,3,3,3,3,3,3,3,3,3,3,3,3,3,3,3,3,3,3,4),(0.,0.0178818661276581,0.0420046277498154,
0.0619147571895479,0.0784556688955424,0.0921046276778006,0.0982358839915246,
0.101631663647595,0.113481879413641,0.122768694086075,0.130945093051513,
0.13492366361535,0.147692763578984,0.162110991450564,0.17292466235425,0.182570798254554,
0.191640000877476,0.198502837971391,0.203003685351385,0.205365675065305,
0.220227760265693,0.237717341084149,0.257888024044024,0.27554448846269,
0.305320512941014,0.336139545307548,0.367581148155728,0.399998147169167,
0.416261364863618,0.451793169604947,0.489270790032098,0.531608562069829,
0.556652585026387,0.593570264533481,0.62366547684941,0.672288902338737,
0.71878877048483,0.762442054669932,0.803766603189827,0.843326669035891,
0.882495001776919,0.902430471697919,0.911523499995539,0.948130494390717,
0.983903842618441,1.),.UNSPECIFIED.);
#1534=B_SPLINE_CURVE_WITH_KNOTS('',5,(#64862,#64863,#64864,#64865,#64866,
#64867,#64868,#64869,#64870,#64871,#64872,#64873,#64874,#64875,#64876,#64877,
#64878,#64879),.UNSPECIFIED.,.F.,.F.,(6,3,3,3,3,6),(2.30144058436,3.21523268549,
4.17948834992,7.86941426972,10.6293166988,11.5241632533),.UNSPECIFIED.);
#1535=B_SPLINE_CURVE_WITH_KNOTS('',5,(#65101,#65102,#65103,#65104,#65105,
#65106),.UNSPECIFIED.,.F.,.F.,(6,6),(0.,1.),.UNSPECIFIED.);
#1536=B_SPLINE_CURVE_WITH_KNOTS('',5,(#65162,#65163,#65164,#65165,#65166,
#65167,#65168,#65169,#65170),.UNSPECIFIED.,.F.,.F.,(6,3,6),(0.,0.492002634808513,
1.),.UNSPECIFIED.);
#1537=B_SPLINE_CURVE_WITH_KNOTS('',3,(#65187,#65188,#65189,#65190,#65191,
#65192,#65193,#65194,#65195,#65196,#65197,#65198,#65199,#65200,#65201,#65202,
#65203,#65204,#65205,#65206,#65207,#65208,#65209,#65210,#65211,#65212,#65213,
#65214,#65215,#65216,#65217),.UNSPECIFIED.,.F.,.F.,(4,3,3,3,3,3,3,3,3,3,
4),(1.01419307112823E-10,0.114803214366508,0.229652502492259,0.344466449061211,
0.459272421602756,0.5,0.614960144518346,0.72996764431242,0.844937159320942,
0.9598873123093,0.999953286395137),.UNSPECIFIED.);
#1538=B_SPLINE_CURVE_WITH_KNOTS('',3,(#65222,#65223,#65224,#65225,#65226,
#65227,#65228,#65229,#65230,#65231,#65232,#65233,#65234,#65235,#65236,#65237,
#65238,#65239,#65240,#65241,#65242,#65243,#65244,#65245,#65246,#65247,#65248,
#65249,#65250,#65251,#65252),.UNSPECIFIED.,.F.,.F.,(4,3,3,3,3,3,3,3,3,3,
4),(5.04394994972232E-5,0.114997722791671,0.230017633717882,0.345013835241517,
0.460010499449355,0.5,0.614795527323077,0.729648824467911,0.844473441242412,
0.959299484217645,0.999999999986445),.UNSPECIFIED.);
#1539=B_SPLINE_CURVE_WITH_KNOTS('',3,(#65309,#65310,#65311,#65312,#65313,
#65314,#65315,#65316,#65317,#65318,#65319,#65320,#65321,#65322,#65323,#65324,
#65325,#65326,#65327,#65328,#65329,#65330,#65331,#65332,#65333,#65334,#65335,
#65336,#65337,#65338,#65339,#65340,#65341,#65342,#65343,#65344,#65345,#65346,
#65347,#65348,#65349,#65350,#65351,#65352,#65353,#65354,#65355,#65356,#65357,
#65358,#65359,#65360),.UNSPECIFIED.,.F.,.F.,(4,3,3,3,3,3,3,3,3,3,3,3,3,
3,3,3,3,4),(0.,0.0437126558078608,0.0915681494956934,0.142416637980807,
0.199087137007962,0.271354736821453,0.329530402979306,0.37856785682181,
0.426556605310522,0.490747528430981,0.556806799843687,0.624244332149857,
0.693278978525398,0.764166499868672,0.838303763782746,0.914636896986591,
0.994157837628613,1.),.UNSPECIFIED.);
#1540=B_SPLINE_CURVE_WITH_KNOTS('',5,(#65415,#65416,#65417,#65418,#65419,
#65420),.UNSPECIFIED.,.F.,.F.,(6,6),(1.41662542015,3.44037602036),
 .UNSPECIFIED.);
#1541=B_SPLINE_CURVE_WITH_KNOTS('',5,(#65488,#65489,#65490,#65491,#65492,
#65493),.UNSPECIFIED.,.F.,.F.,(6,6),(0.,0.999998872761371),
 .UNSPECIFIED.);
#1542=B_SPLINE_CURVE_WITH_KNOTS('',5,(#65496,#65497,#65498,#65499,#65500,
#65501,#65502,#65503,#65504,#65505,#65506,#65507),.UNSPECIFIED.,.F.,.F.,
(6,3,3,6),(0.,0.200980383521308,0.498560958763885,1.),.UNSPECIFIED.);
#1543=B_SPLINE_CURVE_WITH_KNOTS('',5,(#65563,#65564,#65565,#65566,#65567,
#65568),.UNSPECIFIED.,.F.,.F.,(6,6),(1.12325834678787E-6,1.),
 .UNSPECIFIED.);
#1544=B_SPLINE_CURVE_WITH_KNOTS('',5,(#65570,#65571,#65572,#65573,#65574,
#65575,#65576,#65577,#65578,#65579,#65580,#65581),.UNSPECIFIED.,.F.,.F.,
(6,3,3,6),(1.81130449228,3.02278054545,4.81654635721,7.83913682071),
 .UNSPECIFIED.);
#1545=B_SPLINE_CURVE_WITH_KNOTS('',5,(#65675,#65676,#65677,#65678,#65679,
#65680),.UNSPECIFIED.,.F.,.F.,(6,6),(0.,1.),.UNSPECIFIED.);
#1546=B_SPLINE_CURVE_WITH_KNOTS('',5,(#65736,#65737,#65738,#65739,#65740,
#65741),.UNSPECIFIED.,.F.,.F.,(6,6),(-4.0299576811,4.0299576811),
 .UNSPECIFIED.);
#1547=B_SPLINE_CURVE_WITH_KNOTS('',5,(#65742,#65743,#65744,#65745,#65746,
#65747),.UNSPECIFIED.,.F.,.F.,(6,6),(2.67640720078839E-8,1.),
 .UNSPECIFIED.);
#1548=B_SPLINE_CURVE_WITH_KNOTS('',3,(#65817,#65818,#65819,#65820,#65821,
#65822,#65823,#65824,#65825,#65826,#65827,#65828,#65829,#65830,#65831,#65832,
#65833,#65834,#65835,#65836,#65837,#65838,#65839,#65840,#65841,#65842,#65843,
#65844,#65845,#65846,#65847,#65848,#65849,#65850,#65851,#65852,#65853,#65854,
#65855,#65856,#65857,#65858,#65859,#65860,#65861,#65862,#65863,#65864,#65865,
#65866,#65867,#65868,#65869,#65870,#65871),.UNSPECIFIED.,.F.,.F.,(4,3,3,
3,3,3,3,3,3,3,3,3,3,3,3,3,3,3,4),(15.6461121486,16.0896325713055,16.5393779921266,
16.9924984702736,17.4485466874474,17.9069575593301,18.3676660600592,18.8288389264601,
19.2894880382849,19.6759856009261,20.1371224824956,20.598572133874,21.0593729051655,
21.5189112036208,21.9766242126307,22.4305838505212,22.8820570133801,23.3290841703052,
23.7060275108),.UNSPECIFIED.);
#1549=B_SPLINE_CURVE_WITH_KNOTS('',3,(#65927,#65928,#65929,#65930,#65931,
#65932,#65933,#65934,#65935,#65936,#65937,#65938,#65939,#65940,#65941,#65942,
#65943,#65944,#65945,#65946,#65947,#65948,#65949,#65950,#65951,#65952,#65953,
#65954,#65955,#65956,#65957,#65958,#65959,#65960,#65961,#65962,#65963,#65964,
#65965,#65966,#65967,#65968,#65969,#65970,#65971,#65972,#65973,#65974,#65975,
#65976,#65977,#65978,#65979,#65980,#65981),.UNSPECIFIED.,.F.,.F.,(4,3,3,
3,3,3,3,3,3,3,3,3,3,3,3,3,3,3,4),(-4.0299576811,-3.58432646698948,-3.13333878308903,
-2.67943996443098,-2.22299149481985,-1.76443619200231,-1.30366467078965,
-0.842282930845045,-0.380902091971085,8.4271212237035E-5,0.460259241512958,
0.921454150718638,1.38219890167591,1.84169198412367,2.29919664572966,2.75241920254977,
3.20276098063367,3.6479231507545,4.0299576811),.UNSPECIFIED.);
#1550=B_SPLINE_CURVE_WITH_KNOTS('',5,(#66082,#66083,#66084,#66085,#66086,
#66087,#66088,#66089,#66090,#66091,#66092,#66093),.UNSPECIFIED.,.F.,.F.,
(6,3,3,6),(0.,0.501439041305556,0.799019616584482,1.),.UNSPECIFIED.);
#1551=B_SPLINE_CURVE_WITH_KNOTS('',3,(#66149,#66150,#66151,#66152,#66153,
#66154,#66155,#66156,#66157,#66158,#66159,#66160,#66161,#66162,#66163,#66164,
#66165,#66166,#66167,#66168,#66169,#66170,#66171,#66172,#66173,#66174,#66175,
#66176,#66177,#66178,#66179,#66180,#66181,#66182,#66183,#66184,#66185,#66186,
#66187,#66188,#66189,#66190,#66191,#66192,#66193,#66194,#66195,#66196,#66197,
#66198,#66199,#66200,#66201,#66202,#66203,#66204,#66205,#66206,#66207,#66208,
#66209,#66210,#66211,#66212,#66213,#66214,#66215,#66216,#66217,#66218),
 .UNSPECIFIED.,.F.,.F.,(4,3,3,3,3,3,3,3,3,3,3,3,3,3,3,3,3,3,3,3,3,3,3,4),
(0.,0.0416934585115111,0.0842984248119822,0.127942034658533,0.173513963804105,
0.220527053595778,0.269266295706531,0.320117104895673,0.374981888964963,
0.434659850856473,0.486787066144604,0.531102769430081,0.578465001280323,
0.631156876120282,0.679840052794278,0.725322356099277,0.768143786601305,
0.80890232311754,0.848031527918299,0.886023645938725,0.922292844683316,
0.957806742735771,0.992402997682604,1.),.UNSPECIFIED.);
#1552=B_SPLINE_CURVE_WITH_KNOTS('',5,(#66219,#66220,#66221,#66222,#66223,
#66224),.UNSPECIFIED.,.F.,.F.,(6,6),(0.,1.),.UNSPECIFIED.);
#1553=B_SPLINE_CURVE_WITH_KNOTS('',3,(#66342,#66343,#66344,#66345,#66346,
#66347,#66348,#66349,#66350,#66351,#66352,#66353,#66354,#66355,#66356,#66357,
#66358,#66359,#66360,#66361,#66362,#66363,#66364,#66365,#66366,#66367,#66368,
#66369,#66370,#66371,#66372,#66373,#66374,#66375,#66376,#66377,#66378,#66379,
#66380,#66381,#66382,#66383,#66384,#66385,#66386,#66387,#66388,#66389,#66390,
#66391,#66392,#66393,#66394,#66395,#66396,#66397,#66398,#66399,#66400,#66401,
#66402,#66403,#66404,#66405,#66406,#66407,#66408,#66409,#66410,#66411,#66412,
#66413,#66414,#66415,#66416,#66417,#66418,#66419,#66420,#66421,#66422,#66423,
#66424,#66425,#66426),.UNSPECIFIED.,.F.,.F.,(4,3,3,3,3,3,3,3,3,3,3,3,3,
3,3,3,3,3,3,3,3,3,3,3,3,3,3,3,4),(0.,0.0365197170986561,0.0750561518641488,
0.116481352134669,0.157480958781737,0.195741855213761,0.21819216147024,
0.267279631016782,0.28047977872294,0.314494034692517,0.349363219215245,
0.384561538339423,0.416779364169955,0.458265327941776,0.490156495711959,
0.518807853109117,0.555862643296138,0.593061189935473,0.630400857109214,
0.66794626872993,0.705592102349747,0.743377716091016,0.770781707666146,
0.799011186296452,0.822310369292715,0.866732776969536,0.9103813251214,0.9551906625607,
1.),.UNSPECIFIED.);
#1554=B_SPLINE_CURVE_WITH_KNOTS('',5,(#66518,#66519,#66520,#66521,#66522,
#66523,#66524,#66525,#66526,#66527,#66528,#66529,#66530,#66531,#66532,#66533,
#66534,#66535),.UNSPECIFIED.,.F.,.F.,(6,3,3,3,3,6),(2.56814442563,4.26587753681,
5.98143772792,6.84529958826,9.44079904688,11.1645337758),.UNSPECIFIED.);
#1555=B_SPLINE_CURVE_WITH_KNOTS('',5,(#66791,#66792,#66793,#66794,#66795,
#66796,#66797,#66798,#66799,#66800,#66801,#66802,#66803,#66804,#66805,#66806,
#66807,#66808),.UNSPECIFIED.,.F.,.F.,(6,3,3,3,3,6),(2.58143959,4.30538111878,
6.90119302094,7.76515862896,9.48090785315,11.1787837181),.UNSPECIFIED.);
#1556=B_SPLINE_CURVE_WITH_KNOTS('',5,(#66899,#66900,#66901,#66902,#66903,
#66904,#66905,#66906,#66907,#66908,#66909,#66910,#66911,#66912,#66913,#66914,
#66915,#66916),.UNSPECIFIED.,.F.,.F.,(6,3,3,3,3,6),(2.58143959,4.30538111878,
6.90119302094,7.76515862896,9.48090785315,11.1787837181),.UNSPECIFIED.);
#1557=B_SPLINE_CURVE_WITH_KNOTS('',5,(#67047,#67048,#67049,#67050,#67051,
#67052,#67053,#67054,#67055,#67056,#67057,#67058,#67059,#67060,#67061,#67062,
#67063,#67064,#67065,#67066,#67067,#67068,#67069,#67070),.UNSPECIFIED.,
 .F.,.F.,(6,3,3,3,3,3,3,6),(0.,0.298380745521735,0.400355122330922,0.605495111960514,
0.706465344087353,0.806019409718089,0.903240868100526,1.),.UNSPECIFIED.);
#1558=B_SPLINE_CURVE_WITH_KNOTS('',5,(#67146,#67147,#67148,#67149,#67150,
#67151,#67152,#67153,#67154,#67155,#67156,#67157),.UNSPECIFIED.,.F.,.F.,
(6,3,3,6),(0.,0.279839693768996,0.538064414016406,1.),.UNSPECIFIED.);
#1559=B_SPLINE_CURVE_WITH_KNOTS('',3,(#67265,#67266,#67267,#67268,#67269,
#67270,#67271,#67272,#67273,#67274,#67275,#67276,#67277,#67278,#67279,#67280,
#67281,#67282,#67283,#67284,#67285,#67286,#67287,#67288,#67289,#67290,#67291,
#67292,#67293,#67294,#67295,#67296,#67297,#67298,#67299,#67300,#67301,#67302,
#67303,#67304,#67305,#67306,#67307,#67308,#67309,#67310,#67311,#67312,#67313,
#67314,#67315,#67316),.UNSPECIFIED.,.F.,.F.,(4,3,3,3,3,3,3,3,3,3,3,3,3,
3,3,3,3,4),(0.,0.0556187312399707,0.112993438321228,0.172143724257659,0.23389539128623,
0.297764219459196,0.321436234888974,0.41536792214111,0.489370703978092,
0.518718286518054,0.586784525784047,0.656446595575187,0.726367781106817,
0.794775835830112,0.860858656629832,0.925135456699957,0.986994389830349,
1.),.UNSPECIFIED.);
#1560=B_SPLINE_CURVE_WITH_KNOTS('',5,(#67372,#67373,#67374,#67375,#67376,
#67377,#67378,#67379,#67380),.UNSPECIFIED.,.F.,.F.,(6,3,6),(0.,0.498324297489375,
1.),.UNSPECIFIED.);
#1561=B_SPLINE_CURVE_WITH_KNOTS('',3,(#67517,#67518,#67519,#67520,#67521,
#67522,#67523,#67524,#67525,#67526,#67527,#67528,#67529,#67530,#67531,#67532,
#67533,#67534,#67535,#67536,#67537,#67538,#67539,#67540,#67541,#67542,#67543,
#67544,#67545,#67546,#67547,#67548,#67549,#67550,#67551,#67552,#67553,#67554,
#67555,#67556,#67557,#67558,#67559,#67560,#67561,#67562,#67563,#67564,#67565,
#67566,#67567,#67568,#67569,#67570,#67571,#67572,#67573,#67574,#67575,#67576,
#67577,#67578,#67579,#67580,#67581,#67582,#67583,#67584,#67585,#67586,#67587,
#67588,#67589,#67590,#67591,#67592,#67593,#67594,#67595,#67596,#67597,#67598,
#67599,#67600,#67601,#67602,#67603,#67604,#67605,#67606,#67607,#67608,#67609,
#67610,#67611,#67612,#67613,#67614,#67615,#67616,#67617,#67618,#67619,#67620,
#67621,#67622,#67623,#67624,#67625,#67626,#67627,#67628,#67629,#67630,#67631,
#67632,#67633,#67634,#67635,#67636,#67637,#67638,#67639,#67640,#67641,#67642,
#67643,#67644,#67645,#67646),.UNSPECIFIED.,.F.,.F.,(4,3,3,3,3,3,3,3,3,3,
3,3,3,3,3,3,3,3,3,3,3,3,3,3,3,3,3,3,3,3,3,3,3,3,3,3,3,3,3,3,3,3,3,4),(0.,
0.0198013619717458,0.0404159238918976,0.0620723153674499,0.086247822024199,
0.10843867563033,0.125899721004124,0.152218301219973,0.176179069456496,
0.196035357920758,0.216490434219102,0.235983401420272,0.255476368621443,
0.271170775069074,0.282640095018162,0.303570033406706,0.32561749981579,
0.350282440909494,0.377972561891687,0.399923595232346,0.415662554971816,
0.443004349547964,0.467591673748802,0.489986113834325,0.499978765489982,
0.524945472319113,0.549687996167472,0.573101538289844,0.59297413237794,
0.616741323308855,0.637748727055981,0.64050851423977,0.671117738474467,
0.693353256839199,0.714783014437229,0.750668884649306,0.780812121073995,
0.816630656902144,0.853091747051759,0.889818810288819,0.92403816438968,
0.957052970761367,0.988505420883898,1.),.UNSPECIFIED.);
#1562=B_SPLINE_CURVE_WITH_KNOTS('',5,(#67756,#67757,#67758,#67759,#67760,
#67761,#67762,#67763,#67764,#67765,#67766,#67767,#67768,#67769,#67770,#67771,
#67772,#67773),.UNSPECIFIED.,.F.,.F.,(6,3,3,3,3,6),(0.,0.273250853963034,
0.407985073911058,0.581975918956344,0.822728550713782,1.),.UNSPECIFIED.);
#1563=B_SPLINE_CURVE_WITH_KNOTS('',3,(#67977,#67978,#67979,#67980,#67981,
#67982,#67983,#67984,#67985,#67986,#67987,#67988,#67989,#67990,#67991,#67992,
#67993,#67994,#67995,#67996,#67997,#67998,#67999,#68000,#68001,#68002,#68003,
#68004,#68005,#68006,#68007),.UNSPECIFIED.,.F.,.F.,(4,3,3,3,3,3,3,3,3,3,
4),(0.,0.110287887209419,0.223345183110051,0.337717962698899,0.45335852785974,
0.5,0.615745954604195,0.730067416796077,0.84303840753261,0.953657228919592,
1.),.UNSPECIFIED.);
#1564=B_SPLINE_CURVE_WITH_KNOTS('',5,(#68008,#68009,#68010,#68011,#68012,
#68013),.UNSPECIFIED.,.F.,.F.,(6,6),(0.,1.),.UNSPECIFIED.);
#1565=B_SPLINE_CURVE_WITH_KNOTS('',5,(#68069,#68070,#68071,#68072,#68073,
#68074),.UNSPECIFIED.,.F.,.F.,(6,6),(1.41662542015,3.44037602036),
 .UNSPECIFIED.);
#1566=B_SPLINE_CURVE_WITH_KNOTS('',3,(#68075,#68076,#68077,#68078,#68079,
#68080,#68081,#68082,#68083,#68084,#68085,#68086,#68087,#68088,#68089,#68090,
#68091,#68092,#68093,#68094,#68095,#68096,#68097,#68098,#68099,#68100,#68101,
#68102,#68103,#68104,#68105),.UNSPECIFIED.,.F.,.F.,(4,3,3,3,3,3,3,3,3,3,
4),(0.,0.110294928224807,0.223359835487429,0.337740411810181,0.453388630710344,
0.5,0.615739698165253,0.730054755953022,0.843019355200479,0.953631919301136,
1.),.UNSPECIFIED.);
#1567=B_SPLINE_CURVE_WITH_KNOTS('',5,(#68185,#68186,#68187,#68188,#68189,
#68190),.UNSPECIFIED.,.F.,.F.,(6,6),(0.,1.),.UNSPECIFIED.);
#1568=B_SPLINE_CURVE_WITH_KNOTS('',5,(#68246,#68247,#68248,#68249,#68250,
#68251,#68252,#68253,#68254),.UNSPECIFIED.,.F.,.F.,(6,3,6),(0.,0.49200263441696,
1.),.UNSPECIFIED.);
#1569=B_SPLINE_CURVE_WITH_KNOTS('',5,(#68522,#68523,#68524,#68525,#68526,
#68527,#68528,#68529,#68530,#68531,#68532,#68533,#68534,#68535,#68536,#68537,
#68538,#68539),.UNSPECIFIED.,.F.,.F.,(6,3,3,3,3,6),(0.,0.0970262888056245,
0.396276577955941,0.796367315526125,0.900919486282946,0.99999999472897),
 .UNSPECIFIED.);
#1570=B_SPLINE_CURVE_WITH_KNOTS('',5,(#68666,#68667,#68668,#68669,#68670,
#68671,#68672,#68673,#68674,#68675,#68676,#68677,#68678,#68679,#68680,#68681,
#68682,#68683,#68684,#68685,#68686),.UNSPECIFIED.,.F.,.F.,(6,3,3,3,3,3,
6),(0.,0.449905946496647,0.59940190637457,0.692533484718061,0.785665063061551,
0.897922768805432,1.),.UNSPECIFIED.);
#1571=B_SPLINE_CURVE_WITH_KNOTS('',5,(#68798,#68799,#68800,#68801,#68802,
#68803,#68804,#68805,#68806,#68807,#68808,#68809),.UNSPECIFIED.,.F.,.F.,
(6,3,3,6),(0.,0.492684025877734,0.739237878130715,1.),.UNSPECIFIED.);
#1572=B_SPLINE_CURVE_WITH_KNOTS('',5,(#68887,#68888,#68889,#68890,#68891,
#68892,#68893,#68894,#68895,#68896,#68897,#68898,#68899,#68900,#68901,#68902,
#68903,#68904,#68905,#68906,#68907),.UNSPECIFIED.,.F.,.F.,(6,3,3,3,3,3,
6),(0.,0.201339674271977,0.303001917323942,0.506399963286459,0.70776546861359,
0.806334715522354,1.),.UNSPECIFIED.);
#1573=B_SPLINE_CURVE_WITH_KNOTS('',5,(#69008,#69009,#69010,#69011,#69012,
#69013),.UNSPECIFIED.,.F.,.F.,(6,6),(-1.27990980993,-0.52702168644),
 .UNSPECIFIED.);
#1574=B_SPLINE_CURVE_WITH_KNOTS('',3,(#69070,#69071,#69072,#69073,#69074,
#69075,#69076,#69077,#69078,#69079,#69080,#69081,#69082,#69083,#69084,#69085,
#69086,#69087,#69088,#69089,#69090,#69091,#69092,#69093,#69094,#69095,#69096,
#69097,#69098,#69099,#69100,#69101,#69102,#69103,#69104,#69105,#69106,#69107,
#69108,#69109,#69110,#69111,#69112),.UNSPECIFIED.,.F.,.F.,(4,3,3,3,3,3,
3,3,3,3,3,3,3,3,4),(0.,0.0776083637283321,0.155118249326187,0.232531965013796,
0.30981031864142,0.387003342323335,0.46407865662313,0.495424428724466,0.571227612704095,
0.648031014951877,0.725644046554455,0.803923133483166,0.882212778464548,
0.960052978009603,1.),.UNSPECIFIED.);
#1575=B_SPLINE_CURVE_WITH_KNOTS('',5,(#69182,#69183,#69184,#69185,#69186,
#69187,#69188,#69189,#69190),.UNSPECIFIED.,.F.,.F.,(6,3,6),(0.,0.565644588338075,
1.),.UNSPECIFIED.);
#1576=B_SPLINE_CURVE_WITH_KNOTS('',5,(#69247,#69248,#69249,#69250,#69251,
#69252),.UNSPECIFIED.,.F.,.F.,(6,6),(-19.8869526656,-9.07387951837),
 .UNSPECIFIED.);
#1577=B_SPLINE_CURVE_WITH_KNOTS('',5,(#69322,#69323,#69324,#69325,#69326,
#69327,#69328,#69329,#69330),.UNSPECIFIED.,.F.,.F.,(6,3,6),(0.,0.565644588338948,
1.),.UNSPECIFIED.);
#1578=B_SPLINE_CURVE_WITH_KNOTS('',5,(#69387,#69388,#69389,#69390,#69391,
#69392),.UNSPECIFIED.,.F.,.F.,(6,6),(-30.7000258128,-19.8869526656),
 .UNSPECIFIED.);
#1579=B_SPLINE_CURVE_WITH_KNOTS('',5,(#69462,#69463,#69464,#69465,#69466,
#69467),.UNSPECIFIED.,.F.,.F.,(6,6),(-1.27990980993,-0.52702168644),
 .UNSPECIFIED.);
#1580=B_SPLINE_CURVE_WITH_KNOTS('',3,(#69524,#69525,#69526,#69527,#69528,
#69529,#69530,#69531,#69532,#69533,#69534,#69535,#69536,#69537,#69538,#69539,
#69540,#69541,#69542,#69543,#69544,#69545,#69546,#69547,#69548,#69549,#69550,
#69551,#69552,#69553,#69554,#69555,#69556,#69557,#69558,#69559,#69560,#69561,
#69562,#69563,#69564,#69565,#69566),.UNSPECIFIED.,.F.,.F.,(4,3,3,3,3,3,
3,3,3,3,3,3,3,3,4),(0.,0.0776083635899578,0.155118249004403,0.232531964542428,
0.309810318214625,0.38700334212762,0.464078657022176,0.495424428696483,
0.571227612929565,0.648031015392319,0.725644047151879,0.803923134122699,
0.882212779078427,0.960052978513656,1.),.UNSPECIFIED.);
#1581=B_SPLINE_CURVE_WITH_KNOTS('',5,(#69654,#69655,#69656,#69657,#69658,
#69659,#69660,#69661,#69662,#69663,#69664,#69665,#69666,#69667,#69668,#69669,
#69670,#69671,#69672,#69673,#69674),.UNSPECIFIED.,.F.,.F.,(6,3,3,3,3,3,
6),(-8.58012360199,-7.30257258114,-6.6523412175,-5.32399418003,-3.98223908975,
-3.31160417062,-1.98342753277),.UNSPECIFIED.);
#1582=B_SPLINE_CURVE_WITH_KNOTS('',5,(#69749,#69750,#69751,#69752,#69753,
#69754,#69755,#69756,#69757,#69758,#69759,#69760,#69761,#69762,#69763,#69764,
#69765,#69766,#69767,#69768,#69769),.UNSPECIFIED.,.F.,.F.,(6,3,3,3,3,3,
6),(0.,0.193665284476424,0.292234531386853,0.493600036714289,0.696998082675599,
0.798660325727718,1.),.UNSPECIFIED.);
#1583=B_SPLINE_CURVE_WITH_KNOTS('',5,(#69905,#69906,#69907,#69908,#69909,
#69910,#69911,#69912,#69913,#69914,#69915,#69916,#69917,#69918,#69919),
 .UNSPECIFIED.,.F.,.F.,(6,3,3,3,6),(-5.21689863741,-4.48067762876,-3.70557211292,
-2.5282953222,-1.35736905211),.UNSPECIFIED.);
#1584=B_SPLINE_CURVE_WITH_KNOTS('',3,(#70012,#70013,#70014,#70015,#70016,
#70017,#70018,#70019,#70020,#70021,#70022,#70023,#70024,#70025,#70026,#70027,
#70028,#70029,#70030,#70031,#70032,#70033,#70034,#70035,#70036,#70037,#70038,
#70039,#70040,#70041,#70042,#70043,#70044,#70045,#70046,#70047,#70048,#70049,
#70050,#70051,#70052,#70053,#70054,#70055,#70056,#70057,#70058,#70059,#70060,
#70061,#70062,#70063,#70064,#70065,#70066,#70067,#70068,#70069,#70070,#70071,
#70072,#70073,#70074,#70075,#70076,#70077,#70078,#70079,#70080,#70081,#70082,
#70083,#70084,#70085,#70086,#70087,#70088,#70089,#70090,#70091,#70092,#70093,
#70094,#70095,#70096,#70097,#70098,#70099,#70100,#70101,#70102),
 .UNSPECIFIED.,.F.,.F.,(4,3,3,3,3,3,3,3,3,3,3,3,3,3,3,3,3,3,3,3,3,3,3,3,
3,3,3,3,3,3,4),(0.,0.0182662446037865,0.0375259675978898,0.0582758529991181,
0.0820848215164342,0.112848248846866,0.135920819344689,0.156749193614456,
0.17626986474751,0.191579331315563,0.205138530838161,0.22773672177315,0.253447922437721,
0.291000249561992,0.317357678976258,0.328552576686263,0.383012581099915,
0.412561924344558,0.486591650696816,0.492903941799935,0.546128883342705,
0.605058868866327,0.655577068132116,0.688250424539024,0.715729075586451,
0.773576659496423,0.826211419859548,0.874471298494987,0.921087205821898,
0.965827553474194,1.),.UNSPECIFIED.);
#1585=B_SPLINE_CURVE_WITH_KNOTS('',5,(#70316,#70317,#70318,#70319,#70320,
#70321,#70322,#70323,#70324,#70325,#70326,#70327,#70328,#70329,#70330,#70331,
#70332,#70333,#70334,#70335,#70336,#70337,#70338,#70339,#70340,#70341,#70342,
#70343,#70344,#70345,#70346,#70347,#70348,#70349,#70350,#70351,#70352,#70353,
#70354),.UNSPECIFIED.,.F.,.F.,(6,3,3,3,3,3,3,3,3,3,3,3,6),(-31.7310892021,
-30.7075742798,-30.0730233774,-29.43694187,-27.5338438134,-24.9287160587,
-22.3238009285,-21.0213468886,-17.0993514659,-13.7853920845,-8.49590865562,
-6.30725257391,-5.58814360433),.UNSPECIFIED.);
#1586=B_SPLINE_CURVE_WITH_KNOTS('',5,(#70537,#70538,#70539,#70540,#70541,
#70542,#70543,#70544,#70545,#70546,#70547,#70548,#70549,#70550,#70551,#70552,
#70553,#70554,#70555,#70556,#70557,#70558,#70559,#70560,#70561,#70562,#70563,
#70564,#70565,#70566,#70567,#70568,#70569,#70570,#70571,#70572,#70573,#70574,
#70575),.UNSPECIFIED.,.F.,.F.,(6,3,3,3,3,3,3,3,3,3,3,3,6),(0.,0.0391507115551396,
0.063423068318722,0.0877539726164481,0.160549826835811,0.260199185205061,
0.359840410424235,0.409660888190562,0.559682063426246,0.686445108126254,
0.888774390765743,0.97249319259413,1.),.UNSPECIFIED.);
#1587=B_SPLINE_CURVE_WITH_KNOTS('',5,(#70964,#70965,#70966,#70967,#70968,
#70969,#70970,#70971,#70972,#70973,#70974,#70975,#70976,#70977,#70978,#70979,
#70980,#70981,#70982,#70983,#70984,#70985,#70986,#70987,#70988,#70989,#70990,
#70991,#70992,#70993,#70994,#70995,#70996,#70997,#70998,#70999,#71000,#71001,
#71002),.UNSPECIFIED.,.F.,.F.,(6,3,3,3,3,3,3,3,3,3,3,3,6),(-31.8832921784,
-31.1641832088,-28.9755271271,-23.6860436982,-20.3720843168,-16.4500888941,
-15.1476348542,-12.5427197241,-9.9375919693,-8.03449391269,-7.39841240531,
-6.76386150304,-5.7403465807),.UNSPECIFIED.);
#1588=B_SPLINE_CURVE_WITH_KNOTS('',3,(#71167,#71168,#71169,#71170,#71171,
#71172,#71173,#71174,#71175,#71176,#71177,#71178,#71179,#71180,#71181,#71182,
#71183,#71184,#71185,#71186,#71187,#71188,#71189,#71190,#71191,#71192,#71193,
#71194,#71195,#71196,#71197,#71198,#71199,#71200,#71201,#71202,#71203,#71204,
#71205,#71206,#71207,#71208,#71209,#71210,#71211,#71212,#71213,#71214,#71215,
#71216,#71217,#71218,#71219,#71220,#71221,#71222,#71223,#71224,#71225,#71226,
#71227,#71228,#71229,#71230,#71231,#71232,#71233,#71234,#71235,#71236,#71237,
#71238,#71239,#71240,#71241,#71242,#71243,#71244,#71245,#71246,#71247,#71248,
#71249,#71250,#71251,#71252,#71253,#71254,#71255,#71256,#71257,#71258,#71259,
#71260,#71261,#71262,#71263,#71264,#71265,#71266,#71267,#71268,#71269,#71270,
#71271,#71272,#71273,#71274,#71275,#71276,#71277,#71278,#71279,#71280,#71281,
#71282,#71283,#71284,#71285,#71286,#71287,#71288,#71289,#71290,#71291,#71292,
#71293,#71294,#71295,#71296,#71297,#71298,#71299,#71300,#71301,#71302,#71303,
#71304,#71305,#71306,#71307,#71308,#71309,#71310,#71311,#71312,#71313,#71314,
#71315,#71316,#71317,#71318,#71319,#71320,#71321,#71322,#71323,#71324,#71325,
#71326,#71327,#71328,#71329,#71330,#71331,#71332,#71333,#71334,#71335,#71336,
#71337,#71338,#71339,#71340,#71341,#71342,#71343,#71344,#71345,#71346,#71347,
#71348,#71349,#71350,#71351,#71352,#71353,#71354,#71355,#71356,#71357,#71358,
#71359,#71360,#71361,#71362,#71363,#71364,#71365,#71366,#71367,#71368,#71369,
#71370,#71371),.UNSPECIFIED.,.F.,.F.,(4,3,3,3,3,3,3,3,3,3,3,3,3,3,3,3,3,
3,3,3,3,3,3,3,3,3,3,3,3,3,3,3,3,3,3,3,3,3,3,3,3,3,3,3,3,3,3,3,3,3,3,3,3,
3,3,3,3,3,3,3,3,3,3,3,3,3,3,3,4),(0.,0.0154108833739815,0.024396260675666,
0.0322672376773886,0.0509867983195788,0.070655365291477,0.091955212111218,
0.105014263643365,0.118071336189016,0.143019468820527,0.16594610599059,
0.186734949763442,0.206432882601081,0.224937065226494,0.234726017500779,
0.252391337653417,0.270528133993635,0.28952273821895,0.308536692801582,
0.324241359276896,0.345863793558721,0.368477343842195,0.392380882102757,
0.406636273014148,0.429460363972643,0.441722866558087,0.466249444060802,
0.487012897201986,0.499998942837968,0.519585389504108,0.539965369435351,
0.562135064298468,0.585423106641615,0.595055043844164,0.621056567089681,
0.639186449720391,0.670100538908602,0.693969077346171,0.715642974917153,
0.751561803628593,0.78639517991619,0.819094250974915,0.834422620522875,
0.844868688329344,0.859318289762911,0.871664748244572,0.887334416156321,
0.901524270073433,0.911323754293252,0.916718949293115,0.92722086707506,
0.931097752998277,0.935699661236655,0.939658545918256,0.946503170030517,
0.951478794929174,0.955953947599919,0.959463525531288,0.962295311108283,
0.962973103462657,0.96667709714004,0.970584348317267,0.975061015415103,
0.980444468128151,0.985362564279898,0.989550180366893,0.993386213762534,
0.996885676959665,1.),.UNSPECIFIED.);
#1589=B_SPLINE_CURVE_WITH_KNOTS('',5,(#71541,#71542,#71543,#71544,#71545,
#71546,#71547,#71548,#71549,#71550,#71551,#71552,#71553,#71554,#71555),
 .UNSPECIFIED.,.F.,.F.,(6,3,3,3,6),(-4.99954599766,-3.82861972691,-2.65134293549,
-1.87623741919,-1.14001641713),.UNSPECIFIED.);
#1590=B_SPLINE_CURVE_WITH_KNOTS('',3,(#71628,#71629,#71630,#71631,#71632,
#71633,#71634,#71635,#71636,#71637,#71638,#71639,#71640,#71641,#71642,#71643,
#71644,#71645,#71646,#71647,#71648,#71649,#71650,#71651,#71652,#71653,#71654,
#71655,#71656,#71657,#71658,#71659,#71660,#71661,#71662,#71663,#71664,#71665,
#71666,#71667,#71668,#71669,#71670,#71671,#71672,#71673,#71674,#71675,#71676,
#71677,#71678,#71679,#71680,#71681,#71682,#71683,#71684,#71685,#71686,#71687,
#71688,#71689,#71690,#71691,#71692,#71693,#71694,#71695,#71696,#71697,#71698,
#71699,#71700,#71701,#71702,#71703,#71704,#71705,#71706,#71707,#71708,#71709),
 .UNSPECIFIED.,.F.,.F.,(4,3,3,3,3,3,3,3,3,3,3,3,3,3,3,3,3,3,3,3,3,3,3,3,
3,3,3,4),(0.,0.0439316094348881,0.0891820224051535,0.136202678319011,0.187279339885987,
0.24254633142745,0.28611550350907,0.326361772648343,0.391110344479467,0.44490716763704,
0.493862617423488,0.542497006607632,0.600081606137234,0.621499512521632,
0.678028299826536,0.7265832841389,0.769693226668195,0.803454089159351,0.819848941519525,
0.838676687278942,0.859941456517357,0.884377849295373,0.914307868095059,
0.936993329670823,0.957477728773413,0.976663422649514,0.994636879500515,
1.),.UNSPECIFIED.);
#2045=SHAPE_REPRESENTATION_RELATIONSHIP('SRR','None',#98342,#2055);
#2055=ADVANCED_BREP_SHAPE_REPRESENTATION('',(#2075),#98294);
#2065=STYLED_ITEM('',(#98399),#2075);
#2075=MANIFOLD_SOLID_BREP('Body1',#34169);
#2121=PLANE('',#34824);
#2122=PLANE('',#34831);
#2123=PLANE('',#34859);
#2124=PLANE('',#34889);
#2608=CYLINDRICAL_SURFACE('',#34842,3.00001776604858);
#2609=CYLINDRICAL_SURFACE('',#34857,0.3);
#2610=CYLINDRICAL_SURFACE('',#34858,0.300000000000002);
#2611=CYLINDRICAL_SURFACE('',#34884,3.00001778010126);
#2612=CYLINDRICAL_SURFACE('',#34885,0.3);
#2613=CYLINDRICAL_SURFACE('',#34887,0.300000000000002);
#3575=FACE_OUTER_BOUND('',#5723,.T.);
#3576=FACE_OUTER_BOUND('',#5727,.T.);
#3577=FACE_OUTER_BOUND('',#5731,.T.);
#3578=FACE_OUTER_BOUND('',#5732,.T.);
#3579=FACE_OUTER_BOUND('',#5733,.T.);
#3580=FACE_OUTER_BOUND('',#5734,.T.);
#3581=FACE_OUTER_BOUND('',#5735,.T.);
#3582=FACE_OUTER_BOUND('',#5736,.T.);
#3583=FACE_OUTER_BOUND('',#5737,.T.);
#3584=FACE_OUTER_BOUND('',#5738,.T.);
#3585=FACE_OUTER_BOUND('',#5739,.T.);
#3586=FACE_OUTER_BOUND('',#5740,.T.);
#3587=FACE_OUTER_BOUND('',#5741,.T.);
#3588=FACE_OUTER_BOUND('',#5742,.T.);
#3589=FACE_OUTER_BOUND('',#5743,.T.);
#3590=FACE_OUTER_BOUND('',#5744,.T.);
#3591=FACE_OUTER_BOUND('',#5745,.T.);
#3592=FACE_OUTER_BOUND('',#5746,.T.);
#3593=FACE_OUTER_BOUND('',#5747,.T.);
#3594=FACE_OUTER_BOUND('',#5748,.T.);
#3595=FACE_OUTER_BOUND('',#5749,.T.);
#3596=FACE_OUTER_BOUND('',#5750,.T.);
#3597=FACE_OUTER_BOUND('',#5751,.T.);
#3598=FACE_OUTER_BOUND('',#5752,.T.);
#3599=FACE_OUTER_BOUND('',#5753,.T.);
#3600=FACE_OUTER_BOUND('',#5754,.T.);
#3601=FACE_OUTER_BOUND('',#5755,.T.);
#3602=FACE_OUTER_BOUND('',#5756,.T.);
#3603=FACE_OUTER_BOUND('',#5757,.T.);
#3604=FACE_OUTER_BOUND('',#5758,.T.);
#3605=FACE_OUTER_BOUND('',#5759,.T.);
#3606=FACE_OUTER_BOUND('',#5760,.T.);
#3607=FACE_OUTER_BOUND('',#5761,.T.);
#3608=FACE_OUTER_BOUND('',#5762,.T.);
#3609=FACE_OUTER_BOUND('',#5763,.T.);
#3610=FACE_OUTER_BOUND('',#5764,.T.);
#3611=FACE_OUTER_BOUND('',#5765,.T.);
#3612=FACE_OUTER_BOUND('',#5766,.T.);
#3613=FACE_OUTER_BOUND('',#5767,.T.);
#3614=FACE_OUTER_BOUND('',#5768,.T.);
#3615=FACE_OUTER_BOUND('',#5769,.T.);
#3616=FACE_OUTER_BOUND('',#5770,.T.);
#3617=FACE_OUTER_BOUND('',#5771,.T.);
#3618=FACE_OUTER_BOUND('',#5772,.T.);
#3619=FACE_OUTER_BOUND('',#5773,.T.);
#3620=FACE_OUTER_BOUND('',#5774,.T.);
#3621=FACE_OUTER_BOUND('',#5775,.T.);
#3622=FACE_OUTER_BOUND('',#5776,.T.);
#3623=FACE_OUTER_BOUND('',#5777,.T.);
#3624=FACE_OUTER_BOUND('',#5778,.T.);
#3625=FACE_OUTER_BOUND('',#5779,.T.);
#3626=FACE_OUTER_BOUND('',#5780,.T.);
#3627=FACE_OUTER_BOUND('',#5781,.T.);
#3628=FACE_OUTER_BOUND('',#5782,.T.);
#3629=FACE_OUTER_BOUND('',#5783,.T.);
#3630=FACE_OUTER_BOUND('',#5784,.T.);
#3631=FACE_OUTER_BOUND('',#5785,.T.);
#3632=FACE_OUTER_BOUND('',#5786,.T.);
#3633=FACE_OUTER_BOUND('',#5787,.T.);
#3634=FACE_OUTER_BOUND('',#5788,.T.);
#3635=FACE_OUTER_BOUND('',#5789,.T.);
#3636=FACE_OUTER_BOUND('',#5790,.T.);
#3637=FACE_OUTER_BOUND('',#5791,.T.);
#3638=FACE_OUTER_BOUND('',#5792,.T.);
#3639=FACE_OUTER_BOUND('',#5793,.T.);
#3640=FACE_OUTER_BOUND('',#5794,.T.);
#3641=FACE_OUTER_BOUND('',#5795,.T.);
#3642=FACE_OUTER_BOUND('',#5796,.T.);
#3643=FACE_OUTER_BOUND('',#5797,.T.);
#3644=FACE_OUTER_BOUND('',#5798,.T.);
#3645=FACE_OUTER_BOUND('',#5799,.T.);
#3646=FACE_OUTER_BOUND('',#5800,.T.);
#3647=FACE_OUTER_BOUND('',#5801,.T.);
#3648=FACE_OUTER_BOUND('',#5802,.T.);
#3649=FACE_OUTER_BOUND('',#5803,.T.);
#3650=FACE_OUTER_BOUND('',#5804,.T.);
#3651=FACE_OUTER_BOUND('',#5805,.T.);
#3652=FACE_OUTER_BOUND('',#5806,.T.);
#3653=FACE_OUTER_BOUND('',#5807,.T.);
#3654=FACE_OUTER_BOUND('',#5808,.T.);
#3655=FACE_OUTER_BOUND('',#5809,.T.);
#3656=FACE_OUTER_BOUND('',#5810,.T.);
#3657=FACE_OUTER_BOUND('',#5811,.T.);
#3658=FACE_OUTER_BOUND('',#5812,.T.);
#3659=FACE_OUTER_BOUND('',#5813,.T.);
#3660=FACE_OUTER_BOUND('',#5814,.T.);
#3661=FACE_OUTER_BOUND('',#5815,.T.);
#3662=FACE_OUTER_BOUND('',#5816,.T.);
#3663=FACE_OUTER_BOUND('',#5817,.T.);
#3664=FACE_OUTER_BOUND('',#5818,.T.);
#3665=FACE_OUTER_BOUND('',#5819,.T.);
#3666=FACE_OUTER_BOUND('',#5820,.T.);
#3667=FACE_OUTER_BOUND('',#5821,.T.);
#3668=FACE_OUTER_BOUND('',#5822,.T.);
#3669=FACE_OUTER_BOUND('',#5823,.T.);
#3670=FACE_OUTER_BOUND('',#5824,.T.);
#3671=FACE_OUTER_BOUND('',#5825,.T.);
#3672=FACE_OUTER_BOUND('',#5826,.T.);
#3673=FACE_OUTER_BOUND('',#5827,.T.);
#3674=FACE_OUTER_BOUND('',#5828,.T.);
#3675=FACE_OUTER_BOUND('',#5829,.T.);
#3676=FACE_OUTER_BOUND('',#5830,.T.);
#3677=FACE_OUTER_BOUND('',#5831,.T.);
#3678=FACE_OUTER_BOUND('',#5832,.T.);
#3679=FACE_OUTER_BOUND('',#5833,.T.);
#3680=FACE_OUTER_BOUND('',#5834,.T.);
#3681=FACE_OUTER_BOUND('',#5835,.T.);
#3682=FACE_OUTER_BOUND('',#5836,.T.);
#3683=FACE_OUTER_BOUND('',#5837,.T.);
#3684=FACE_OUTER_BOUND('',#5838,.T.);
#5723=EDGE_LOOP('',(#23223,#23224,#23225,#23226,#23227,#23228,#23229,#23230,
#23231,#23232,#23233));
#5724=EDGE_LOOP('',(#23234,#23235,#23236,#23237,#23238,#23239,#23240,#23241,
#23242));
#5725=EDGE_LOOP('',(#23243,#23244,#23245,#23246,#23247,#23248,#23249,#23250,
#23251));
#5726=EDGE_LOOP('',(#23252,#23253,#23254,#23255,#23256,#23257,#23258));
#5727=EDGE_LOOP('',(#23259,#23260,#23261,#23262,#23263,#23264,#23265,#23266,
#23267,#23268,#23269));
#5728=EDGE_LOOP('',(#23270,#23271,#23272,#23273,#23274,#23275,#23276,#23277,
#23278));
#5729=EDGE_LOOP('',(#23279,#23280,#23281,#23282,#23283,#23284,#23285,#23286,
#23287));
#5730=EDGE_LOOP('',(#23288,#23289,#23290,#23291,#23292,#23293,#23294));
#5731=EDGE_LOOP('',(#23295,#23296,#23297,#23298));
#5732=EDGE_LOOP('',(#23299,#23300,#23301,#23302));
#5733=EDGE_LOOP('',(#23303,#23304,#23305,#23306));
#5734=EDGE_LOOP('',(#23307,#23308,#23309,#23310));
#5735=EDGE_LOOP('',(#23311,#23312,#23313,#23314));
#5736=EDGE_LOOP('',(#23315,#23316,#23317,#23318));
#5737=EDGE_LOOP('',(#23319,#23320,#23321,#23322));
#5738=EDGE_LOOP('',(#23323,#23324,#23325,#23326));
#5739=EDGE_LOOP('',(#23327,#23328,#23329,#23330));
#5740=EDGE_LOOP('',(#23331,#23332,#23333,#23334));
#5741=EDGE_LOOP('',(#23335,#23336,#23337,#23338));
#5742=EDGE_LOOP('',(#23339,#23340,#23341,#23342));
#5743=EDGE_LOOP('',(#23343,#23344,#23345,#23346));
#5744=EDGE_LOOP('',(#23347,#23348,#23349,#23350));
#5745=EDGE_LOOP('',(#23351,#23352,#23353,#23354));
#5746=EDGE_LOOP('',(#23355,#23356,#23357,#23358));
#5747=EDGE_LOOP('',(#23359,#23360,#23361,#23362));
#5748=EDGE_LOOP('',(#23363,#23364,#23365,#23366));
#5749=EDGE_LOOP('',(#23367,#23368,#23369,#23370));
#5750=EDGE_LOOP('',(#23371,#23372,#23373,#23374));
#5751=EDGE_LOOP('',(#23375,#23376,#23377,#23378));
#5752=EDGE_LOOP('',(#23379,#23380,#23381,#23382));
#5753=EDGE_LOOP('',(#23383,#23384,#23385,#23386));
#5754=EDGE_LOOP('',(#23387,#23388,#23389,#23390));
#5755=EDGE_LOOP('',(#23391,#23392,#23393,#23394));
#5756=EDGE_LOOP('',(#23395,#23396,#23397,#23398));
#5757=EDGE_LOOP('',(#23399,#23400,#23401,#23402));
#5758=EDGE_LOOP('',(#23403,#23404,#23405,#23406));
#5759=EDGE_LOOP('',(#23407,#23408,#23409,#23410));
#5760=EDGE_LOOP('',(#23411,#23412,#23413,#23414));
#5761=EDGE_LOOP('',(#23415,#23416,#23417,#23418));
#5762=EDGE_LOOP('',(#23419,#23420,#23421,#23422));
#5763=EDGE_LOOP('',(#23423,#23424,#23425,#23426));
#5764=EDGE_LOOP('',(#23427,#23428,#23429,#23430));
#5765=EDGE_LOOP('',(#23431,#23432,#23433,#23434));
#5766=EDGE_LOOP('',(#23435,#23436,#23437,#23438));
#5767=EDGE_LOOP('',(#23439,#23440,#23441,#23442));
#5768=EDGE_LOOP('',(#23443,#23444,#23445,#23446));
#5769=EDGE_LOOP('',(#23447,#23448,#23449,#23450));
#5770=EDGE_LOOP('',(#23451,#23452,#23453,#23454));
#5771=EDGE_LOOP('',(#23455,#23456,#23457,#23458));
#5772=EDGE_LOOP('',(#23459,#23460,#23461,#23462));
#5773=EDGE_LOOP('',(#23463,#23464,#23465,#23466));
#5774=EDGE_LOOP('',(#23467,#23468,#23469,#23470));
#5775=EDGE_LOOP('',(#23471,#23472,#23473,#23474));
#5776=EDGE_LOOP('',(#23475,#23476,#23477,#23478));
#5777=EDGE_LOOP('',(#23479,#23480,#23481,#23482));
#5778=EDGE_LOOP('',(#23483,#23484,#23485,#23486));
#5779=EDGE_LOOP('',(#23487,#23488,#23489,#23490));
#5780=EDGE_LOOP('',(#23491,#23492,#23493,#23494));
#5781=EDGE_LOOP('',(#23495,#23496,#23497,#23498));
#5782=EDGE_LOOP('',(#23499,#23500,#23501,#23502));
#5783=EDGE_LOOP('',(#23503,#23504,#23505,#23506));
#5784=EDGE_LOOP('',(#23507,#23508,#23509,#23510));
#5785=EDGE_LOOP('',(#23511,#23512,#23513,#23514));
#5786=EDGE_LOOP('',(#23515,#23516,#23517,#23518));
#5787=EDGE_LOOP('',(#23519,#23520,#23521,#23522));
#5788=EDGE_LOOP('',(#23523,#23524,#23525,#23526));
#5789=EDGE_LOOP('',(#23527,#23528,#23529,#23530));
#5790=EDGE_LOOP('',(#23531,#23532,#23533,#23534));
#5791=EDGE_LOOP('',(#23535,#23536,#23537,#23538));
#5792=EDGE_LOOP('',(#23539,#23540,#23541,#23542));
#5793=EDGE_LOOP('',(#23543,#23544,#23545,#23546));
#5794=EDGE_LOOP('',(#23547,#23548,#23549,#23550));
#5795=EDGE_LOOP('',(#23551,#23552,#23553,#23554));
#5796=EDGE_LOOP('',(#23555,#23556,#23557,#23558));
#5797=EDGE_LOOP('',(#23559,#23560,#23561,#23562));
#5798=EDGE_LOOP('',(#23563,#23564,#23565,#23566));
#5799=EDGE_LOOP('',(#23567,#23568,#23569,#23570));
#5800=EDGE_LOOP('',(#23571,#23572,#23573,#23574));
#5801=EDGE_LOOP('',(#23575,#23576,#23577,#23578));
#5802=EDGE_LOOP('',(#23579,#23580,#23581,#23582));
#5803=EDGE_LOOP('',(#23583,#23584,#23585,#23586));
#5804=EDGE_LOOP('',(#23587,#23588,#23589,#23590));
#5805=EDGE_LOOP('',(#23591,#23592,#23593,#23594));
#5806=EDGE_LOOP('',(#23595,#23596,#23597,#23598));
#5807=EDGE_LOOP('',(#23599,#23600,#23601,#23602));
#5808=EDGE_LOOP('',(#23603,#23604,#23605,#23606));
#5809=EDGE_LOOP('',(#23607,#23608,#23609,#23610));
#5810=EDGE_LOOP('',(#23611,#23612,#23613,#23614));
#5811=EDGE_LOOP('',(#23615,#23616,#23617,#23618));
#5812=EDGE_LOOP('',(#23619,#23620,#23621,#23622));
#5813=EDGE_LOOP('',(#23623,#23624,#23625,#23626));
#5814=EDGE_LOOP('',(#23627,#23628,#23629,#23630));
#5815=EDGE_LOOP('',(#23631,#23632,#23633,#23634));
#5816=EDGE_LOOP('',(#23635,#23636,#23637,#23638));
#5817=EDGE_LOOP('',(#23639,#23640,#23641,#23642));
#5818=EDGE_LOOP('',(#23643,#23644,#23645,#23646));
#5819=EDGE_LOOP('',(#23647,#23648,#23649,#23650));
#5820=EDGE_LOOP('',(#23651,#23652,#23653,#23654));
#5821=EDGE_LOOP('',(#23655,#23656,#23657,#23658));
#5822=EDGE_LOOP('',(#23659,#23660,#23661,#23662));
#5823=EDGE_LOOP('',(#23663,#23664,#23665,#23666));
#5824=EDGE_LOOP('',(#23667,#23668,#23669,#23670));
#5825=EDGE_LOOP('',(#23671,#23672,#23673,#23674));
#5826=EDGE_LOOP('',(#23675,#23676,#23677,#23678));
#5827=EDGE_LOOP('',(#23679,#23680,#23681,#23682));
#5828=EDGE_LOOP('',(#23683,#23684,#23685,#23686));
#5829=EDGE_LOOP('',(#23687,#23688,#23689,#23690));
#5830=EDGE_LOOP('',(#23691,#23692,#23693,#23694));
#5831=EDGE_LOOP('',(#23695,#23696,#23697,#23698));
#5832=EDGE_LOOP('',(#23699,#23700,#23701,#23702));
#5833=EDGE_LOOP('',(#23703,#23704,#23705,#23706));
#5834=EDGE_LOOP('',(#23707,#23708,#23709,#23710));
#5835=EDGE_LOOP('',(#23711,#23712,#23713,#23714));
#5836=EDGE_LOOP('',(#23715,#23716,#23717,#23718));
#5837=EDGE_LOOP('',(#23719,#23720,#23721,#23722));
#5838=EDGE_LOOP('',(#23723,#23724,#23725,#23726));
#7872=LINE('',#59325,#9712);
#7873=LINE('',#59592,#9713);
#7874=LINE('',#61893,#9714);
#7875=LINE('',#62811,#9715);
#7876=LINE('',#63497,#9716);
#7877=LINE('',#63498,#9717);
#7878=LINE('',#63912,#9718);
#7879=LINE('',#64113,#9719);
#7880=LINE('',#64470,#9720);
#7881=LINE('',#64917,#9721);
#7882=LINE('',#65044,#9722);
#7883=LINE('',#65184,#9723);
#7884=LINE('',#65218,#9724);
#7885=LINE('',#65221,#9725);
#7886=LINE('',#65254,#9726);
#7887=LINE('',#65617,#9727);
#7888=LINE('',#65618,#9728);
#7889=LINE('',#65760,#9729);
#7890=LINE('',#65995,#9730);
#7891=LINE('',#66249,#9731);
#7892=LINE('',#66573,#9732);
#7893=LINE('',#66700,#9733);
#7894=LINE('',#67207,#9734);
#7895=LINE('',#67208,#9735);
#7896=LINE('',#67406,#9736);
#7897=LINE('',#67823,#9737);
#7898=LINE('',#67921,#9738);
#7899=LINE('',#68118,#9739);
#7900=LINE('',#68122,#9740);
#7901=LINE('',#68125,#9741);
#7902=LINE('',#68128,#9742);
#7903=LINE('',#68268,#9743);
#7904=LINE('',#68395,#9744);
#7905=LINE('',#68950,#9745);
#7906=LINE('',#68951,#9746);
#7907=LINE('',#69125,#9747);
#7908=LINE('',#69265,#9748);
#7909=LINE('',#69405,#9749);
#7910=LINE('',#69579,#9750);
#7911=LINE('',#69812,#9751);
#7912=LINE('',#70133,#9752);
#7913=LINE('',#70654,#9753);
#7914=LINE('',#70781,#9754);
#7915=LINE('',#71450,#9755);
#9712=VECTOR('',#39925,1000.);
#9713=VECTOR('',#39930,1000.);
#9714=VECTOR('',#39939,1000.);
#9715=VECTOR('',#39944,1000.);
#9716=VECTOR('',#39961,1000.);
#9717=VECTOR('',#39962,1000.);
#9718=VECTOR('',#39967,1000.);
#9719=VECTOR('',#39972,1000.);
#9720=VECTOR('',#39977,1000.);
#9721=VECTOR('',#39982,1000.);
#9722=VECTOR('',#39991,1000.);
#9723=VECTOR('',#39996,1000.);
#9724=VECTOR('',#39999,1000.);
#9725=VECTOR('',#40002,1000.);
#9726=VECTOR('',#40005,1000.);
#9727=VECTOR('',#40010,1000.);
#9728=VECTOR('',#40011,1000.);
#9729=VECTOR('',#40014,1000.);
#9730=VECTOR('',#40019,1000.);
#9731=VECTOR('',#40022,1000.);
#9732=VECTOR('',#40027,1000.);
#9733=VECTOR('',#40036,1000.);
#9734=VECTOR('',#40045,1000.);
#9735=VECTOR('',#40046,1000.);
#9736=VECTOR('',#40051,1000.);
#9737=VECTOR('',#40056,1000.);
#9738=VECTOR('',#40067,1000.);
#9739=VECTOR('',#40068,1000.);
#9740=VECTOR('',#40073,1000.);
#9741=VECTOR('',#40076,1000.);
#9742=VECTOR('',#40081,1000.);
#9743=VECTOR('',#40086,1000.);
#9744=VECTOR('',#40095,1000.);
#9745=VECTOR('',#40104,1000.);
#9746=VECTOR('',#40105,1000.);
#9747=VECTOR('',#40110,1000.);
#9748=VECTOR('',#40115,1000.);
#9749=VECTOR('',#40120,1000.);
#9750=VECTOR('',#40125,1000.);
#9751=VECTOR('',#40130,1000.);
#9752=VECTOR('',#40135,1000.);
#9753=VECTOR('',#40140,1000.);
#9754=VECTOR('',#40149,1000.);
#9755=VECTOR('',#40154,1000.);
#14055=VERTEX_POINT('',#57908);
#14056=VERTEX_POINT('',#57909);
#14057=VERTEX_POINT('',#58115);
#14058=VERTEX_POINT('',#58117);
#14059=VERTEX_POINT('',#58308);
#14060=VERTEX_POINT('',#58400);
#14061=VERTEX_POINT('',#58489);
#14062=VERTEX_POINT('',#58557);
#14063=VERTEX_POINT('',#58625);
#14064=VERTEX_POINT('',#58693);
#14065=VERTEX_POINT('',#58761);
#14066=VERTEX_POINT('',#58950);
#14067=VERTEX_POINT('',#58951);
#14068=VERTEX_POINT('',#59016);
#14069=VERTEX_POINT('',#59138);
#14070=VERTEX_POINT('',#59281);
#14071=VERTEX_POINT('',#59283);
#14072=VERTEX_POINT('',#59324);
#14073=VERTEX_POINT('',#59326);
#14074=VERTEX_POINT('',#59382);
#14075=VERTEX_POINT('',#59535);
#14076=VERTEX_POINT('',#59536);
#14077=VERTEX_POINT('',#59538);
#14078=VERTEX_POINT('',#59591);
#14079=VERTEX_POINT('',#59593);
#14080=VERTEX_POINT('',#59634);
#14081=VERTEX_POINT('',#59636);
#14082=VERTEX_POINT('',#59782);
#14083=VERTEX_POINT('',#59910);
#14084=VERTEX_POINT('',#60126);
#14085=VERTEX_POINT('',#60127);
#14086=VERTEX_POINT('',#60192);
#14087=VERTEX_POINT('',#60269);
#14088=VERTEX_POINT('',#60367);
#14089=VERTEX_POINT('',#60369);
#14090=VERTEX_POINT('',#60461);
#14091=VERTEX_POINT('',#60609);
#14092=VERTEX_POINT('',#60610);
#14093=VERTEX_POINT('',#60699);
#14094=VERTEX_POINT('',#60794);
#14095=VERTEX_POINT('',#60862);
#14096=VERTEX_POINT('',#60936);
#14097=VERTEX_POINT('',#61010);
#14098=VERTEX_POINT('',#61078);
#14099=VERTEX_POINT('',#61173);
#14100=VERTEX_POINT('',#61271);
#14101=VERTEX_POINT('',#61447);
#14102=VERTEX_POINT('',#61651);
#14103=VERTEX_POINT('',#61652);
#14104=VERTEX_POINT('',#61801);
#14105=VERTEX_POINT('',#61827);
#14106=VERTEX_POINT('',#61892);
#14107=VERTEX_POINT('',#61894);
#14108=VERTEX_POINT('',#61947);
#14109=VERTEX_POINT('',#61949);
#14110=VERTEX_POINT('',#62089);
#14111=VERTEX_POINT('',#62272);
#14112=VERTEX_POINT('',#62273);
#14113=VERTEX_POINT('',#62422);
#14114=VERTEX_POINT('',#62478);
#14115=VERTEX_POINT('',#62609);
#14116=VERTEX_POINT('',#62761);
#14117=VERTEX_POINT('',#62763);
#14118=VERTEX_POINT('',#62810);
#14119=VERTEX_POINT('',#62812);
#14120=VERTEX_POINT('',#62887);
#14121=VERTEX_POINT('',#62888);
#14122=VERTEX_POINT('',#62950);
#14123=VERTEX_POINT('',#63036);
#14124=VERTEX_POINT('',#63137);
#14125=VERTEX_POINT('',#63139);
#14126=VERTEX_POINT('',#63246);
#14127=VERTEX_POINT('',#63450);
#14128=VERTEX_POINT('',#63452);
#14129=VERTEX_POINT('',#63491);
#14130=VERTEX_POINT('',#63493);
#14131=VERTEX_POINT('',#63607);
#14132=VERTEX_POINT('',#63741);
#14133=VERTEX_POINT('',#63967);
#14134=VERTEX_POINT('',#64078);
#14135=VERTEX_POINT('',#64204);
#14136=VERTEX_POINT('',#64405);
#14137=VERTEX_POINT('',#64615);
#14138=VERTEX_POINT('',#64861);
#14139=VERTEX_POINT('',#64972);
#14140=VERTEX_POINT('',#65029);
#14141=VERTEX_POINT('',#65099);
#14142=VERTEX_POINT('',#65161);
#14143=VERTEX_POINT('',#65186);
#14144=VERTEX_POINT('',#65220);
#14145=VERTEX_POINT('',#65487);
#14146=VERTEX_POINT('',#65494);
#14147=VERTEX_POINT('',#65562);
#14148=VERTEX_POINT('',#65569);
#14149=VERTEX_POINT('',#65673);
#14150=VERTEX_POINT('',#65735);
#14151=VERTEX_POINT('',#65815);
#14152=VERTEX_POINT('',#65926);
#14153=VERTEX_POINT('',#66080);
#14154=VERTEX_POINT('',#66148);
#14155=VERTEX_POINT('',#66340);
#14156=VERTEX_POINT('',#66517);
#14157=VERTEX_POINT('',#66628);
#14158=VERTEX_POINT('',#66685);
#14159=VERTEX_POINT('',#67043);
#14160=VERTEX_POINT('',#67045);
#14161=VERTEX_POINT('',#67143);
#14162=VERTEX_POINT('',#67145);
#14163=VERTEX_POINT('',#67263);
#14164=VERTEX_POINT('',#67371);
#14165=VERTEX_POINT('',#67515);
#14166=VERTEX_POINT('',#67755);
#14167=VERTEX_POINT('',#67878);
#14168=VERTEX_POINT('',#67917);
#14169=VERTEX_POINT('',#67976);
#14170=VERTEX_POINT('',#68068);
#14171=VERTEX_POINT('',#68120);
#14172=VERTEX_POINT('',#68124);
#14173=VERTEX_POINT('',#68183);
#14174=VERTEX_POINT('',#68245);
#14175=VERTEX_POINT('',#68323);
#14176=VERTEX_POINT('',#68380);
#14177=VERTEX_POINT('',#68795);
#14178=VERTEX_POINT('',#68797);
#14179=VERTEX_POINT('',#68883);
#14180=VERTEX_POINT('',#68885);
#14181=VERTEX_POINT('',#69006);
#14182=VERTEX_POINT('',#69068);
#14183=VERTEX_POINT('',#69180);
#14184=VERTEX_POINT('',#69245);
#14185=VERTEX_POINT('',#69320);
#14186=VERTEX_POINT('',#69385);
#14187=VERTEX_POINT('',#69460);
#14188=VERTEX_POINT('',#69522);
#14189=VERTEX_POINT('',#69652);
#14190=VERTEX_POINT('',#69747);
#14191=VERTEX_POINT('',#69903);
#14192=VERTEX_POINT('',#70010);
#14193=VERTEX_POINT('',#70314);
#14194=VERTEX_POINT('',#70535);
#14195=VERTEX_POINT('',#70709);
#14196=VERTEX_POINT('',#70766);
#14197=VERTEX_POINT('',#70962);
#14198=VERTEX_POINT('',#71165);
#17383=EDGE_CURVE('',#14055,#14056,#1469,.T.);
#17384=EDGE_CURVE('',#14056,#14057,#483,.T.);
#17385=EDGE_CURVE('',#14057,#14058,#1470,.T.);
#17386=EDGE_CURVE('',#14058,#14059,#1471,.T.);
#17387=EDGE_CURVE('',#14059,#14060,#1472,.T.);
#17388=EDGE_CURVE('',#14060,#14061,#1473,.T.);
#17389=EDGE_CURVE('',#14061,#14062,#1474,.T.);
#17390=EDGE_CURVE('',#14062,#14063,#1475,.T.);
#17391=EDGE_CURVE('',#14063,#14064,#1476,.T.);
#17392=EDGE_CURVE('',#14064,#14065,#1477,.T.);
#17393=EDGE_CURVE('',#14065,#14055,#1478,.T.);
#17394=EDGE_CURVE('',#14066,#14067,#1479,.T.);
#17395=EDGE_CURVE('',#14068,#14066,#1480,.T.);
#17396=EDGE_CURVE('',#14069,#14068,#1481,.T.);
#17397=EDGE_CURVE('',#14070,#14069,#484,.T.);
#17398=EDGE_CURVE('',#14071,#14070,#1482,.T.);
#17399=EDGE_CURVE('',#14072,#14071,#7872,.T.);
#17400=EDGE_CURVE('',#14073,#14072,#1483,.T.);
#17401=EDGE_CURVE('',#14074,#14073,#485,.T.);
#17402=EDGE_CURVE('',#14067,#14074,#1484,.T.);
#17403=EDGE_CURVE('',#14075,#14076,#486,.T.);
#17404=EDGE_CURVE('',#14077,#14075,#1485,.T.);
#17405=EDGE_CURVE('',#14078,#14077,#7873,.T.);
#17406=EDGE_CURVE('',#14079,#14078,#1486,.T.);
#17407=EDGE_CURVE('',#14080,#14079,#487,.T.);
#17408=EDGE_CURVE('',#14081,#14080,#1487,.T.);
#17409=EDGE_CURVE('',#14082,#14081,#1488,.T.);
#17410=EDGE_CURVE('',#14083,#14082,#1489,.T.);
#17411=EDGE_CURVE('',#14076,#14083,#1490,.T.);
#17412=EDGE_CURVE('',#14084,#14085,#1491,.T.);
#17413=EDGE_CURVE('',#14086,#14084,#1492,.T.);
#17414=EDGE_CURVE('',#14087,#14086,#1493,.T.);
#17415=EDGE_CURVE('',#14088,#14087,#488,.T.);
#17416=EDGE_CURVE('',#14089,#14088,#1494,.T.);
#17417=EDGE_CURVE('',#14090,#14089,#1495,.T.);
#17418=EDGE_CURVE('',#14085,#14090,#1496,.T.);
#17419=EDGE_CURVE('',#14091,#14092,#1497,.T.);
#17420=EDGE_CURVE('',#14093,#14091,#1498,.T.);
#17421=EDGE_CURVE('',#14094,#14093,#1499,.T.);
#17422=EDGE_CURVE('',#14095,#14094,#1500,.T.);
#17423=EDGE_CURVE('',#14096,#14095,#1501,.T.);
#17424=EDGE_CURVE('',#14097,#14096,#1502,.T.);
#17425=EDGE_CURVE('',#14098,#14097,#1503,.T.);
#17426=EDGE_CURVE('',#14099,#14098,#1504,.T.);
#17427=EDGE_CURVE('',#14100,#14099,#1505,.T.);
#17428=EDGE_CURVE('',#14101,#14100,#489,.T.);
#17429=EDGE_CURVE('',#14092,#14101,#1506,.T.);
#17430=EDGE_CURVE('',#14102,#14103,#1507,.T.);
#17431=EDGE_CURVE('',#14103,#14104,#1508,.T.);
#17432=EDGE_CURVE('',#14104,#14105,#1509,.T.);
#17433=EDGE_CURVE('',#14105,#14106,#7874,.T.);
#17434=EDGE_CURVE('',#14106,#14107,#1510,.T.);
#17435=EDGE_CURVE('',#14107,#14108,#490,.T.);
#17436=EDGE_CURVE('',#14108,#14109,#1511,.T.);
#17437=EDGE_CURVE('',#14109,#14110,#1512,.T.);
#17438=EDGE_CURVE('',#14110,#14102,#1513,.T.);
#17439=EDGE_CURVE('',#14111,#14112,#1514,.T.);
#17440=EDGE_CURVE('',#14112,#14113,#1515,.T.);
#17441=EDGE_CURVE('',#14113,#14114,#1516,.T.);
#17442=EDGE_CURVE('',#14114,#14115,#1517,.T.);
#17443=EDGE_CURVE('',#14115,#14116,#491,.T.);
#17444=EDGE_CURVE('',#14116,#14117,#1518,.T.);
#17445=EDGE_CURVE('',#14117,#14118,#7875,.T.);
#17446=EDGE_CURVE('',#14118,#14119,#1519,.T.);
#17447=EDGE_CURVE('',#14119,#14111,#1520,.T.);
#17448=EDGE_CURVE('',#14120,#14121,#1521,.T.);
#17449=EDGE_CURVE('',#14121,#14122,#1522,.T.);
#17450=EDGE_CURVE('',#14122,#14123,#1523,.T.);
#17451=EDGE_CURVE('',#14123,#14124,#492,.T.);
#17452=EDGE_CURVE('',#14124,#14125,#1524,.T.);
#17453=EDGE_CURVE('',#14125,#14126,#1525,.T.);
#17454=EDGE_CURVE('',#14126,#14120,#1526,.T.);
#17455=EDGE_CURVE('',#14127,#14075,#493,.T.);
#17456=EDGE_CURVE('',#14128,#14076,#494,.T.);
#17457=EDGE_CURVE('',#14127,#14128,#495,.T.);
#17458=EDGE_CURVE('',#14119,#14129,#496,.T.);
#17459=EDGE_CURVE('',#14129,#14130,#497,.T.);
#17460=EDGE_CURVE('',#14111,#14130,#498,.T.);
#17461=EDGE_CURVE('',#14129,#14127,#7876,.T.);
#17462=EDGE_CURVE('',#14130,#14128,#7877,.T.);
#17463=EDGE_CURVE('',#14131,#14083,#499,.T.);
#17464=EDGE_CURVE('',#14128,#14131,#1527,.T.);
#17465=EDGE_CURVE('',#14130,#14132,#1528,.T.);
#17466=EDGE_CURVE('',#14112,#14132,#500,.T.);
#17467=EDGE_CURVE('',#14132,#14131,#7878,.T.);
#17468=EDGE_CURVE('',#14133,#14082,#501,.T.);
#17469=EDGE_CURVE('',#14131,#14133,#1529,.T.);
#17470=EDGE_CURVE('',#14132,#14134,#1530,.T.);
#17471=EDGE_CURVE('',#14113,#14134,#502,.T.);
#17472=EDGE_CURVE('',#14134,#14133,#7879,.T.);
#17473=EDGE_CURVE('',#14135,#14081,#503,.T.);
#17474=EDGE_CURVE('',#14133,#14135,#1531,.T.);
#17475=EDGE_CURVE('',#14134,#14136,#1532,.T.);
#17476=EDGE_CURVE('',#14114,#14136,#504,.T.);
#17477=EDGE_CURVE('',#14136,#14135,#7880,.T.);
#17478=EDGE_CURVE('',#14137,#14080,#505,.T.);
#17479=EDGE_CURVE('',#14135,#14137,#1533,.T.);
#17480=EDGE_CURVE('',#14136,#14138,#1534,.T.);
#17481=EDGE_CURVE('',#14115,#14138,#506,.T.);
#17482=EDGE_CURVE('',#14138,#14137,#7881,.T.);
#17483=EDGE_CURVE('',#14139,#14079,#507,.T.);
#17484=EDGE_CURVE('',#14137,#14139,#508,.T.);
#17485=EDGE_CURVE('',#14138,#14140,#509,.T.);
#17486=EDGE_CURVE('',#14116,#14140,#510,.T.);
#17487=EDGE_CURVE('',#14140,#14139,#7882,.T.);
#17488=EDGE_CURVE('',#14141,#14078,#511,.T.);
#17489=EDGE_CURVE('',#14139,#14141,#1535,.T.);
#17490=EDGE_CURVE('',#14140,#14142,#1536,.T.);
#17491=EDGE_CURVE('',#14117,#14142,#512,.T.);
#17492=EDGE_CURVE('',#14142,#14141,#7883,.T.);
#17493=EDGE_CURVE('',#14143,#14077,#1537,.T.);
#17494=EDGE_CURVE('',#14141,#14143,#7884,.T.);
#17495=EDGE_CURVE('',#14142,#14144,#7885,.T.);
#17496=EDGE_CURVE('',#14118,#14144,#1538,.T.);
#17497=EDGE_CURVE('',#14144,#14143,#7886,.T.);
#17498=EDGE_CURVE('',#14143,#14127,#1539,.T.);
#17499=EDGE_CURVE('',#14144,#14129,#1540,.T.);
#17500=EDGE_CURVE('',#14145,#14086,#1541,.T.);
#17501=EDGE_CURVE('',#14146,#14084,#513,.T.);
#17502=EDGE_CURVE('',#14145,#14146,#1542,.T.);
#17503=EDGE_CURVE('',#14125,#14147,#1543,.T.);
#17504=EDGE_CURVE('',#14147,#14148,#1544,.T.);
#17505=EDGE_CURVE('',#14126,#14148,#514,.T.);
#17506=EDGE_CURVE('',#14147,#14145,#7887,.T.);
#17507=EDGE_CURVE('',#14148,#14146,#7888,.T.);
#17508=EDGE_CURVE('',#14149,#14085,#515,.T.);
#17509=EDGE_CURVE('',#14146,#14149,#1545,.T.);
#17510=EDGE_CURVE('',#14148,#14150,#1546,.T.);
#17511=EDGE_CURVE('',#14120,#14150,#1547,.T.);
#17512=EDGE_CURVE('',#14150,#14149,#7889,.T.);
#17513=EDGE_CURVE('',#14151,#14090,#516,.T.);
#17514=EDGE_CURVE('',#14149,#14151,#1548,.T.);
#17515=EDGE_CURVE('',#14150,#14152,#1549,.T.);
#17516=EDGE_CURVE('',#14121,#14152,#517,.T.);
#17517=EDGE_CURVE('',#14152,#14151,#7890,.T.);
#17518=EDGE_CURVE('',#14153,#14089,#518,.T.);
#17519=EDGE_CURVE('',#14151,#14153,#1550,.T.);
#17520=EDGE_CURVE('',#14152,#14154,#1551,.T.);
#17521=EDGE_CURVE('',#14122,#14154,#1552,.T.);
#17522=EDGE_CURVE('',#14154,#14153,#7891,.T.);
#17523=EDGE_CURVE('',#14155,#14088,#519,.T.);
#17524=EDGE_CURVE('',#14153,#14155,#1553,.T.);
#17525=EDGE_CURVE('',#14154,#14156,#1554,.T.);
#17526=EDGE_CURVE('',#14123,#14156,#520,.T.);
#17527=EDGE_CURVE('',#14156,#14155,#7892,.T.);
#17528=EDGE_CURVE('',#14157,#14087,#521,.T.);
#17529=EDGE_CURVE('',#14155,#14157,#522,.T.);
#17530=EDGE_CURVE('',#14156,#14158,#523,.T.);
#17531=EDGE_CURVE('',#14124,#14158,#524,.T.);
#17532=EDGE_CURVE('',#14158,#14157,#7893,.T.);
#17533=EDGE_CURVE('',#14157,#14145,#1555,.T.);
#17534=EDGE_CURVE('',#14158,#14147,#1556,.T.);
#17535=EDGE_CURVE('',#14159,#14068,#525,.T.);
#17536=EDGE_CURVE('',#14160,#14066,#526,.T.);
#17537=EDGE_CURVE('',#14159,#14160,#1557,.T.);
#17538=EDGE_CURVE('',#14109,#14161,#527,.T.);
#17539=EDGE_CURVE('',#14161,#14162,#1558,.T.);
#17540=EDGE_CURVE('',#14110,#14162,#528,.T.);
#17541=EDGE_CURVE('',#14161,#14159,#7894,.T.);
#17542=EDGE_CURVE('',#14162,#14160,#7895,.T.);
#17543=EDGE_CURVE('',#14163,#14067,#529,.T.);
#17544=EDGE_CURVE('',#14160,#14163,#1559,.T.);
#17545=EDGE_CURVE('',#14162,#14164,#1560,.T.);
#17546=EDGE_CURVE('',#14102,#14164,#530,.T.);
#17547=EDGE_CURVE('',#14164,#14163,#7896,.T.);
#17548=EDGE_CURVE('',#14165,#14074,#531,.T.);
#17549=EDGE_CURVE('',#14163,#14165,#1561,.T.);
#17550=EDGE_CURVE('',#14164,#14166,#1562,.T.);
#17551=EDGE_CURVE('',#14103,#14166,#532,.T.);
#17552=EDGE_CURVE('',#14166,#14165,#7897,.T.);
#17553=EDGE_CURVE('',#14167,#14073,#533,.T.);
#17554=EDGE_CURVE('',#14165,#14167,#534,.T.);
#17555=EDGE_CURVE('',#14166,#14168,#535,.T.);
#17556=EDGE_CURVE('',#14104,#14168,#536,.T.);
#17557=EDGE_CURVE('',#14168,#14167,#7898,.T.);
#17558=EDGE_CURVE('',#14169,#14072,#1563,.T.);
#17559=EDGE_CURVE('',#14167,#14169,#1564,.T.);
#17560=EDGE_CURVE('',#14168,#14170,#1565,.T.);
#17561=EDGE_CURVE('',#14105,#14170,#1566,.T.);
#17562=EDGE_CURVE('',#14170,#14169,#7899,.T.);
#17563=EDGE_CURVE('',#14171,#14071,#537,.T.);
#17564=EDGE_CURVE('',#14169,#14171,#7900,.T.);
#17565=EDGE_CURVE('',#14170,#14172,#7901,.T.);
#17566=EDGE_CURVE('',#14106,#14172,#538,.T.);
#17567=EDGE_CURVE('',#14172,#14171,#7902,.T.);
#17568=EDGE_CURVE('',#14173,#14070,#539,.T.);
#17569=EDGE_CURVE('',#14171,#14173,#1567,.T.);
#17570=EDGE_CURVE('',#14172,#14174,#1568,.T.);
#17571=EDGE_CURVE('',#14107,#14174,#540,.T.);
#17572=EDGE_CURVE('',#14174,#14173,#7903,.T.);
#17573=EDGE_CURVE('',#14175,#14069,#541,.T.);
#17574=EDGE_CURVE('',#14173,#14175,#542,.T.);
#17575=EDGE_CURVE('',#14174,#14176,#543,.T.);
#17576=EDGE_CURVE('',#14108,#14176,#544,.T.);
#17577=EDGE_CURVE('',#14176,#14175,#7904,.T.);
#17578=EDGE_CURVE('',#14175,#14159,#1569,.T.);
#17579=EDGE_CURVE('',#14176,#14161,#1570,.T.);
#17580=EDGE_CURVE('',#14064,#14177,#545,.T.);
#17581=EDGE_CURVE('',#14177,#14178,#1571,.T.);
#17582=EDGE_CURVE('',#14065,#14178,#546,.T.);
#17583=EDGE_CURVE('',#14179,#14093,#547,.T.);
#17584=EDGE_CURVE('',#14180,#14091,#548,.T.);
#17585=EDGE_CURVE('',#14179,#14180,#1572,.T.);
#17586=EDGE_CURVE('',#14180,#14178,#7905,.T.);
#17587=EDGE_CURVE('',#14179,#14177,#7906,.T.);
#17588=EDGE_CURVE('',#14063,#14181,#549,.T.);
#17589=EDGE_CURVE('',#14181,#14177,#1573,.T.);
#17590=EDGE_CURVE('',#14182,#14094,#550,.T.);
#17591=EDGE_CURVE('',#14182,#14179,#1574,.T.);
#17592=EDGE_CURVE('',#14182,#14181,#7907,.T.);
#17593=EDGE_CURVE('',#14062,#14183,#551,.T.);
#17594=EDGE_CURVE('',#14183,#14181,#1575,.T.);
#17595=EDGE_CURVE('',#14184,#14095,#552,.T.);
#17596=EDGE_CURVE('',#14184,#14182,#1576,.T.);
#17597=EDGE_CURVE('',#14184,#14183,#7908,.T.);
#17598=EDGE_CURVE('',#14061,#14185,#553,.T.);
#17599=EDGE_CURVE('',#14185,#14183,#1577,.T.);
#17600=EDGE_CURVE('',#14186,#14096,#554,.T.);
#17601=EDGE_CURVE('',#14186,#14184,#1578,.T.);
#17602=EDGE_CURVE('',#14186,#14185,#7909,.T.);
#17603=EDGE_CURVE('',#14060,#14187,#555,.T.);
#17604=EDGE_CURVE('',#14187,#14185,#1579,.T.);
#17605=EDGE_CURVE('',#14188,#14097,#556,.T.);
#17606=EDGE_CURVE('',#14188,#14186,#1580,.T.);
#17607=EDGE_CURVE('',#14188,#14187,#7910,.T.);
#17608=EDGE_CURVE('',#14059,#14189,#557,.T.);
#17609=EDGE_CURVE('',#14189,#14187,#1581,.T.);
#17610=EDGE_CURVE('',#14190,#14098,#558,.T.);
#17611=EDGE_CURVE('',#14190,#14188,#1582,.T.);
#17612=EDGE_CURVE('',#14190,#14189,#7911,.T.);
#17613=EDGE_CURVE('',#14058,#14191,#559,.T.);
#17614=EDGE_CURVE('',#14191,#14189,#1583,.T.);
#17615=EDGE_CURVE('',#14192,#14099,#560,.T.);
#17616=EDGE_CURVE('',#14192,#14190,#1584,.T.);
#17617=EDGE_CURVE('',#14192,#14191,#7912,.T.);
#17618=EDGE_CURVE('',#14057,#14193,#561,.T.);
#17619=EDGE_CURVE('',#14193,#14191,#1585,.T.);
#17620=EDGE_CURVE('',#14194,#14100,#562,.T.);
#17621=EDGE_CURVE('',#14194,#14192,#1586,.T.);
#17622=EDGE_CURVE('',#14194,#14193,#7913,.T.);
#17623=EDGE_CURVE('',#14056,#14195,#563,.T.);
#17624=EDGE_CURVE('',#14195,#14193,#564,.T.);
#17625=EDGE_CURVE('',#14196,#14101,#565,.T.);
#17626=EDGE_CURVE('',#14196,#14194,#566,.T.);
#17627=EDGE_CURVE('',#14196,#14195,#7914,.T.);
#17628=EDGE_CURVE('',#14055,#14197,#567,.T.);
#17629=EDGE_CURVE('',#14197,#14195,#1587,.T.);
#17630=EDGE_CURVE('',#14198,#14092,#568,.T.);
#17631=EDGE_CURVE('',#14198,#14196,#1588,.T.);
#17632=EDGE_CURVE('',#14198,#14197,#7915,.T.);
#17633=EDGE_CURVE('',#14178,#14197,#1589,.T.);
#17634=EDGE_CURVE('',#14180,#14198,#1590,.T.);
#23223=ORIENTED_EDGE('',*,*,#17383,.T.);
#23224=ORIENTED_EDGE('',*,*,#17384,.T.);
#23225=ORIENTED_EDGE('',*,*,#17385,.T.);
#23226=ORIENTED_EDGE('',*,*,#17386,.T.);
#23227=ORIENTED_EDGE('',*,*,#17387,.T.);
#23228=ORIENTED_EDGE('',*,*,#17388,.T.);
#23229=ORIENTED_EDGE('',*,*,#17389,.T.);
#23230=ORIENTED_EDGE('',*,*,#17390,.T.);
#23231=ORIENTED_EDGE('',*,*,#17391,.T.);
#23232=ORIENTED_EDGE('',*,*,#17392,.T.);
#23233=ORIENTED_EDGE('',*,*,#17393,.T.);
#23234=ORIENTED_EDGE('',*,*,#17394,.F.);
#23235=ORIENTED_EDGE('',*,*,#17395,.F.);
#23236=ORIENTED_EDGE('',*,*,#17396,.F.);
#23237=ORIENTED_EDGE('',*,*,#17397,.F.);
#23238=ORIENTED_EDGE('',*,*,#17398,.F.);
#23239=ORIENTED_EDGE('',*,*,#17399,.F.);
#23240=ORIENTED_EDGE('',*,*,#17400,.F.);
#23241=ORIENTED_EDGE('',*,*,#17401,.F.);
#23242=ORIENTED_EDGE('',*,*,#17402,.F.);
#23243=ORIENTED_EDGE('',*,*,#17403,.F.);
#23244=ORIENTED_EDGE('',*,*,#17404,.F.);
#23245=ORIENTED_EDGE('',*,*,#17405,.F.);
#23246=ORIENTED_EDGE('',*,*,#17406,.F.);
#23247=ORIENTED_EDGE('',*,*,#17407,.F.);
#23248=ORIENTED_EDGE('',*,*,#17408,.F.);
#23249=ORIENTED_EDGE('',*,*,#17409,.F.);
#23250=ORIENTED_EDGE('',*,*,#17410,.F.);
#23251=ORIENTED_EDGE('',*,*,#17411,.F.);
#23252=ORIENTED_EDGE('',*,*,#17412,.F.);
#23253=ORIENTED_EDGE('',*,*,#17413,.F.);
#23254=ORIENTED_EDGE('',*,*,#17414,.F.);
#23255=ORIENTED_EDGE('',*,*,#17415,.F.);
#23256=ORIENTED_EDGE('',*,*,#17416,.F.);
#23257=ORIENTED_EDGE('',*,*,#17417,.F.);
#23258=ORIENTED_EDGE('',*,*,#17418,.F.);
#23259=ORIENTED_EDGE('',*,*,#17419,.F.);
#23260=ORIENTED_EDGE('',*,*,#17420,.F.);
#23261=ORIENTED_EDGE('',*,*,#17421,.F.);
#23262=ORIENTED_EDGE('',*,*,#17422,.F.);
#23263=ORIENTED_EDGE('',*,*,#17423,.F.);
#23264=ORIENTED_EDGE('',*,*,#17424,.F.);
#23265=ORIENTED_EDGE('',*,*,#17425,.F.);
#23266=ORIENTED_EDGE('',*,*,#17426,.F.);
#23267=ORIENTED_EDGE('',*,*,#17427,.F.);
#23268=ORIENTED_EDGE('',*,*,#17428,.F.);
#23269=ORIENTED_EDGE('',*,*,#17429,.F.);
#23270=ORIENTED_EDGE('',*,*,#17430,.T.);
#23271=ORIENTED_EDGE('',*,*,#17431,.T.);
#23272=ORIENTED_EDGE('',*,*,#17432,.T.);
#23273=ORIENTED_EDGE('',*,*,#17433,.T.);
#23274=ORIENTED_EDGE('',*,*,#17434,.T.);
#23275=ORIENTED_EDGE('',*,*,#17435,.T.);
#23276=ORIENTED_EDGE('',*,*,#17436,.T.);
#23277=ORIENTED_EDGE('',*,*,#17437,.T.);
#23278=ORIENTED_EDGE('',*,*,#17438,.T.);
#23279=ORIENTED_EDGE('',*,*,#17439,.T.);
#23280=ORIENTED_EDGE('',*,*,#17440,.T.);
#23281=ORIENTED_EDGE('',*,*,#17441,.T.);
#23282=ORIENTED_EDGE('',*,*,#17442,.T.);
#23283=ORIENTED_EDGE('',*,*,#17443,.T.);
#23284=ORIENTED_EDGE('',*,*,#17444,.T.);
#23285=ORIENTED_EDGE('',*,*,#17445,.T.);
#23286=ORIENTED_EDGE('',*,*,#17446,.T.);
#23287=ORIENTED_EDGE('',*,*,#17447,.T.);
#23288=ORIENTED_EDGE('',*,*,#17448,.T.);
#23289=ORIENTED_EDGE('',*,*,#17449,.T.);
#23290=ORIENTED_EDGE('',*,*,#17450,.T.);
#23291=ORIENTED_EDGE('',*,*,#17451,.T.);
#23292=ORIENTED_EDGE('',*,*,#17452,.T.);
#23293=ORIENTED_EDGE('',*,*,#17453,.T.);
#23294=ORIENTED_EDGE('',*,*,#17454,.T.);
#23295=ORIENTED_EDGE('',*,*,#17455,.T.);
#23296=ORIENTED_EDGE('',*,*,#17403,.T.);
#23297=ORIENTED_EDGE('',*,*,#17456,.F.);
#23298=ORIENTED_EDGE('',*,*,#17457,.F.);
#23299=ORIENTED_EDGE('',*,*,#17458,.T.);
#23300=ORIENTED_EDGE('',*,*,#17459,.T.);
#23301=ORIENTED_EDGE('',*,*,#17460,.F.);
#23302=ORIENTED_EDGE('',*,*,#17447,.F.);
#23303=ORIENTED_EDGE('',*,*,#17459,.F.);
#23304=ORIENTED_EDGE('',*,*,#17461,.T.);
#23305=ORIENTED_EDGE('',*,*,#17457,.T.);
#23306=ORIENTED_EDGE('',*,*,#17462,.F.);
#23307=ORIENTED_EDGE('',*,*,#17456,.T.);
#23308=ORIENTED_EDGE('',*,*,#17411,.T.);
#23309=ORIENTED_EDGE('',*,*,#17463,.F.);
#23310=ORIENTED_EDGE('',*,*,#17464,.F.);
#23311=ORIENTED_EDGE('',*,*,#17460,.T.);
#23312=ORIENTED_EDGE('',*,*,#17465,.T.);
#23313=ORIENTED_EDGE('',*,*,#17466,.F.);
#23314=ORIENTED_EDGE('',*,*,#17439,.F.);
#23315=ORIENTED_EDGE('',*,*,#17465,.F.);
#23316=ORIENTED_EDGE('',*,*,#17462,.T.);
#23317=ORIENTED_EDGE('',*,*,#17464,.T.);
#23318=ORIENTED_EDGE('',*,*,#17467,.F.);
#23319=ORIENTED_EDGE('',*,*,#17463,.T.);
#23320=ORIENTED_EDGE('',*,*,#17410,.T.);
#23321=ORIENTED_EDGE('',*,*,#17468,.F.);
#23322=ORIENTED_EDGE('',*,*,#17469,.F.);
#23323=ORIENTED_EDGE('',*,*,#17466,.T.);
#23324=ORIENTED_EDGE('',*,*,#17470,.T.);
#23325=ORIENTED_EDGE('',*,*,#17471,.F.);
#23326=ORIENTED_EDGE('',*,*,#17440,.F.);
#23327=ORIENTED_EDGE('',*,*,#17470,.F.);
#23328=ORIENTED_EDGE('',*,*,#17467,.T.);
#23329=ORIENTED_EDGE('',*,*,#17469,.T.);
#23330=ORIENTED_EDGE('',*,*,#17472,.F.);
#23331=ORIENTED_EDGE('',*,*,#17468,.T.);
#23332=ORIENTED_EDGE('',*,*,#17409,.T.);
#23333=ORIENTED_EDGE('',*,*,#17473,.F.);
#23334=ORIENTED_EDGE('',*,*,#17474,.F.);
#23335=ORIENTED_EDGE('',*,*,#17471,.T.);
#23336=ORIENTED_EDGE('',*,*,#17475,.T.);
#23337=ORIENTED_EDGE('',*,*,#17476,.F.);
#23338=ORIENTED_EDGE('',*,*,#17441,.F.);
#23339=ORIENTED_EDGE('',*,*,#17475,.F.);
#23340=ORIENTED_EDGE('',*,*,#17472,.T.);
#23341=ORIENTED_EDGE('',*,*,#17474,.T.);
#23342=ORIENTED_EDGE('',*,*,#17477,.F.);
#23343=ORIENTED_EDGE('',*,*,#17473,.T.);
#23344=ORIENTED_EDGE('',*,*,#17408,.T.);
#23345=ORIENTED_EDGE('',*,*,#17478,.F.);
#23346=ORIENTED_EDGE('',*,*,#17479,.F.);
#23347=ORIENTED_EDGE('',*,*,#17476,.T.);
#23348=ORIENTED_EDGE('',*,*,#17480,.T.);
#23349=ORIENTED_EDGE('',*,*,#17481,.F.);
#23350=ORIENTED_EDGE('',*,*,#17442,.F.);
#23351=ORIENTED_EDGE('',*,*,#17480,.F.);
#23352=ORIENTED_EDGE('',*,*,#17477,.T.);
#23353=ORIENTED_EDGE('',*,*,#17479,.T.);
#23354=ORIENTED_EDGE('',*,*,#17482,.F.);
#23355=ORIENTED_EDGE('',*,*,#17478,.T.);
#23356=ORIENTED_EDGE('',*,*,#17407,.T.);
#23357=ORIENTED_EDGE('',*,*,#17483,.F.);
#23358=ORIENTED_EDGE('',*,*,#17484,.F.);
#23359=ORIENTED_EDGE('',*,*,#17481,.T.);
#23360=ORIENTED_EDGE('',*,*,#17485,.T.);
#23361=ORIENTED_EDGE('',*,*,#17486,.F.);
#23362=ORIENTED_EDGE('',*,*,#17443,.F.);
#23363=ORIENTED_EDGE('',*,*,#17485,.F.);
#23364=ORIENTED_EDGE('',*,*,#17482,.T.);
#23365=ORIENTED_EDGE('',*,*,#17484,.T.);
#23366=ORIENTED_EDGE('',*,*,#17487,.F.);
#23367=ORIENTED_EDGE('',*,*,#17483,.T.);
#23368=ORIENTED_EDGE('',*,*,#17406,.T.);
#23369=ORIENTED_EDGE('',*,*,#17488,.F.);
#23370=ORIENTED_EDGE('',*,*,#17489,.F.);
#23371=ORIENTED_EDGE('',*,*,#17486,.T.);
#23372=ORIENTED_EDGE('',*,*,#17490,.T.);
#23373=ORIENTED_EDGE('',*,*,#17491,.F.);
#23374=ORIENTED_EDGE('',*,*,#17444,.F.);
#23375=ORIENTED_EDGE('',*,*,#17490,.F.);
#23376=ORIENTED_EDGE('',*,*,#17487,.T.);
#23377=ORIENTED_EDGE('',*,*,#17489,.T.);
#23378=ORIENTED_EDGE('',*,*,#17492,.F.);
#23379=ORIENTED_EDGE('',*,*,#17488,.T.);
#23380=ORIENTED_EDGE('',*,*,#17405,.T.);
#23381=ORIENTED_EDGE('',*,*,#17493,.F.);
#23382=ORIENTED_EDGE('',*,*,#17494,.F.);
#23383=ORIENTED_EDGE('',*,*,#17491,.T.);
#23384=ORIENTED_EDGE('',*,*,#17495,.T.);
#23385=ORIENTED_EDGE('',*,*,#17496,.F.);
#23386=ORIENTED_EDGE('',*,*,#17445,.F.);
#23387=ORIENTED_EDGE('',*,*,#17495,.F.);
#23388=ORIENTED_EDGE('',*,*,#17492,.T.);
#23389=ORIENTED_EDGE('',*,*,#17494,.T.);
#23390=ORIENTED_EDGE('',*,*,#17497,.F.);
#23391=ORIENTED_EDGE('',*,*,#17493,.T.);
#23392=ORIENTED_EDGE('',*,*,#17404,.T.);
#23393=ORIENTED_EDGE('',*,*,#17455,.F.);
#23394=ORIENTED_EDGE('',*,*,#17498,.F.);
#23395=ORIENTED_EDGE('',*,*,#17496,.T.);
#23396=ORIENTED_EDGE('',*,*,#17499,.T.);
#23397=ORIENTED_EDGE('',*,*,#17458,.F.);
#23398=ORIENTED_EDGE('',*,*,#17446,.F.);
#23399=ORIENTED_EDGE('',*,*,#17499,.F.);
#23400=ORIENTED_EDGE('',*,*,#17497,.T.);
#23401=ORIENTED_EDGE('',*,*,#17498,.T.);
#23402=ORIENTED_EDGE('',*,*,#17461,.F.);
#23403=ORIENTED_EDGE('',*,*,#17500,.T.);
#23404=ORIENTED_EDGE('',*,*,#17413,.T.);
#23405=ORIENTED_EDGE('',*,*,#17501,.F.);
#23406=ORIENTED_EDGE('',*,*,#17502,.F.);
#23407=ORIENTED_EDGE('',*,*,#17503,.T.);
#23408=ORIENTED_EDGE('',*,*,#17504,.T.);
#23409=ORIENTED_EDGE('',*,*,#17505,.F.);
#23410=ORIENTED_EDGE('',*,*,#17453,.F.);
#23411=ORIENTED_EDGE('',*,*,#17504,.F.);
#23412=ORIENTED_EDGE('',*,*,#17506,.T.);
#23413=ORIENTED_EDGE('',*,*,#17502,.T.);
#23414=ORIENTED_EDGE('',*,*,#17507,.F.);
#23415=ORIENTED_EDGE('',*,*,#17501,.T.);
#23416=ORIENTED_EDGE('',*,*,#17412,.T.);
#23417=ORIENTED_EDGE('',*,*,#17508,.F.);
#23418=ORIENTED_EDGE('',*,*,#17509,.F.);
#23419=ORIENTED_EDGE('',*,*,#17505,.T.);
#23420=ORIENTED_EDGE('',*,*,#17510,.T.);
#23421=ORIENTED_EDGE('',*,*,#17511,.F.);
#23422=ORIENTED_EDGE('',*,*,#17454,.F.);
#23423=ORIENTED_EDGE('',*,*,#17510,.F.);
#23424=ORIENTED_EDGE('',*,*,#17507,.T.);
#23425=ORIENTED_EDGE('',*,*,#17509,.T.);
#23426=ORIENTED_EDGE('',*,*,#17512,.F.);
#23427=ORIENTED_EDGE('',*,*,#17508,.T.);
#23428=ORIENTED_EDGE('',*,*,#17418,.T.);
#23429=ORIENTED_EDGE('',*,*,#17513,.F.);
#23430=ORIENTED_EDGE('',*,*,#17514,.F.);
#23431=ORIENTED_EDGE('',*,*,#17511,.T.);
#23432=ORIENTED_EDGE('',*,*,#17515,.T.);
#23433=ORIENTED_EDGE('',*,*,#17516,.F.);
#23434=ORIENTED_EDGE('',*,*,#17448,.F.);
#23435=ORIENTED_EDGE('',*,*,#17515,.F.);
#23436=ORIENTED_EDGE('',*,*,#17512,.T.);
#23437=ORIENTED_EDGE('',*,*,#17514,.T.);
#23438=ORIENTED_EDGE('',*,*,#17517,.F.);
#23439=ORIENTED_EDGE('',*,*,#17513,.T.);
#23440=ORIENTED_EDGE('',*,*,#17417,.T.);
#23441=ORIENTED_EDGE('',*,*,#17518,.F.);
#23442=ORIENTED_EDGE('',*,*,#17519,.F.);
#23443=ORIENTED_EDGE('',*,*,#17516,.T.);
#23444=ORIENTED_EDGE('',*,*,#17520,.T.);
#23445=ORIENTED_EDGE('',*,*,#17521,.F.);
#23446=ORIENTED_EDGE('',*,*,#17449,.F.);
#23447=ORIENTED_EDGE('',*,*,#17520,.F.);
#23448=ORIENTED_EDGE('',*,*,#17517,.T.);
#23449=ORIENTED_EDGE('',*,*,#17519,.T.);
#23450=ORIENTED_EDGE('',*,*,#17522,.F.);
#23451=ORIENTED_EDGE('',*,*,#17518,.T.);
#23452=ORIENTED_EDGE('',*,*,#17416,.T.);
#23453=ORIENTED_EDGE('',*,*,#17523,.F.);
#23454=ORIENTED_EDGE('',*,*,#17524,.F.);
#23455=ORIENTED_EDGE('',*,*,#17521,.T.);
#23456=ORIENTED_EDGE('',*,*,#17525,.T.);
#23457=ORIENTED_EDGE('',*,*,#17526,.F.);
#23458=ORIENTED_EDGE('',*,*,#17450,.F.);
#23459=ORIENTED_EDGE('',*,*,#17525,.F.);
#23460=ORIENTED_EDGE('',*,*,#17522,.T.);
#23461=ORIENTED_EDGE('',*,*,#17524,.T.);
#23462=ORIENTED_EDGE('',*,*,#17527,.F.);
#23463=ORIENTED_EDGE('',*,*,#17523,.T.);
#23464=ORIENTED_EDGE('',*,*,#17415,.T.);
#23465=ORIENTED_EDGE('',*,*,#17528,.F.);
#23466=ORIENTED_EDGE('',*,*,#17529,.F.);
#23467=ORIENTED_EDGE('',*,*,#17526,.T.);
#23468=ORIENTED_EDGE('',*,*,#17530,.T.);
#23469=ORIENTED_EDGE('',*,*,#17531,.F.);
#23470=ORIENTED_EDGE('',*,*,#17451,.F.);
#23471=ORIENTED_EDGE('',*,*,#17530,.F.);
#23472=ORIENTED_EDGE('',*,*,#17527,.T.);
#23473=ORIENTED_EDGE('',*,*,#17529,.T.);
#23474=ORIENTED_EDGE('',*,*,#17532,.F.);
#23475=ORIENTED_EDGE('',*,*,#17528,.T.);
#23476=ORIENTED_EDGE('',*,*,#17414,.T.);
#23477=ORIENTED_EDGE('',*,*,#17500,.F.);
#23478=ORIENTED_EDGE('',*,*,#17533,.F.);
#23479=ORIENTED_EDGE('',*,*,#17531,.T.);
#23480=ORIENTED_EDGE('',*,*,#17534,.T.);
#23481=ORIENTED_EDGE('',*,*,#17503,.F.);
#23482=ORIENTED_EDGE('',*,*,#17452,.F.);
#23483=ORIENTED_EDGE('',*,*,#17534,.F.);
#23484=ORIENTED_EDGE('',*,*,#17532,.T.);
#23485=ORIENTED_EDGE('',*,*,#17533,.T.);
#23486=ORIENTED_EDGE('',*,*,#17506,.F.);
#23487=ORIENTED_EDGE('',*,*,#17535,.T.);
#23488=ORIENTED_EDGE('',*,*,#17395,.T.);
#23489=ORIENTED_EDGE('',*,*,#17536,.F.);
#23490=ORIENTED_EDGE('',*,*,#17537,.F.);
#23491=ORIENTED_EDGE('',*,*,#17538,.T.);
#23492=ORIENTED_EDGE('',*,*,#17539,.T.);
#23493=ORIENTED_EDGE('',*,*,#17540,.F.);
#23494=ORIENTED_EDGE('',*,*,#17437,.F.);
#23495=ORIENTED_EDGE('',*,*,#17539,.F.);
#23496=ORIENTED_EDGE('',*,*,#17541,.T.);
#23497=ORIENTED_EDGE('',*,*,#17537,.T.);
#23498=ORIENTED_EDGE('',*,*,#17542,.F.);
#23499=ORIENTED_EDGE('',*,*,#17536,.T.);
#23500=ORIENTED_EDGE('',*,*,#17394,.T.);
#23501=ORIENTED_EDGE('',*,*,#17543,.F.);
#23502=ORIENTED_EDGE('',*,*,#17544,.F.);
#23503=ORIENTED_EDGE('',*,*,#17540,.T.);
#23504=ORIENTED_EDGE('',*,*,#17545,.T.);
#23505=ORIENTED_EDGE('',*,*,#17546,.F.);
#23506=ORIENTED_EDGE('',*,*,#17438,.F.);
#23507=ORIENTED_EDGE('',*,*,#17545,.F.);
#23508=ORIENTED_EDGE('',*,*,#17542,.T.);
#23509=ORIENTED_EDGE('',*,*,#17544,.T.);
#23510=ORIENTED_EDGE('',*,*,#17547,.F.);
#23511=ORIENTED_EDGE('',*,*,#17543,.T.);
#23512=ORIENTED_EDGE('',*,*,#17402,.T.);
#23513=ORIENTED_EDGE('',*,*,#17548,.F.);
#23514=ORIENTED_EDGE('',*,*,#17549,.F.);
#23515=ORIENTED_EDGE('',*,*,#17546,.T.);
#23516=ORIENTED_EDGE('',*,*,#17550,.T.);
#23517=ORIENTED_EDGE('',*,*,#17551,.F.);
#23518=ORIENTED_EDGE('',*,*,#17430,.F.);
#23519=ORIENTED_EDGE('',*,*,#17550,.F.);
#23520=ORIENTED_EDGE('',*,*,#17547,.T.);
#23521=ORIENTED_EDGE('',*,*,#17549,.T.);
#23522=ORIENTED_EDGE('',*,*,#17552,.F.);
#23523=ORIENTED_EDGE('',*,*,#17548,.T.);
#23524=ORIENTED_EDGE('',*,*,#17401,.T.);
#23525=ORIENTED_EDGE('',*,*,#17553,.F.);
#23526=ORIENTED_EDGE('',*,*,#17554,.F.);
#23527=ORIENTED_EDGE('',*,*,#17551,.T.);
#23528=ORIENTED_EDGE('',*,*,#17555,.T.);
#23529=ORIENTED_EDGE('',*,*,#17556,.F.);
#23530=ORIENTED_EDGE('',*,*,#17431,.F.);
#23531=ORIENTED_EDGE('',*,*,#17555,.F.);
#23532=ORIENTED_EDGE('',*,*,#17552,.T.);
#23533=ORIENTED_EDGE('',*,*,#17554,.T.);
#23534=ORIENTED_EDGE('',*,*,#17557,.F.);
#23535=ORIENTED_EDGE('',*,*,#17553,.T.);
#23536=ORIENTED_EDGE('',*,*,#17400,.T.);
#23537=ORIENTED_EDGE('',*,*,#17558,.F.);
#23538=ORIENTED_EDGE('',*,*,#17559,.F.);
#23539=ORIENTED_EDGE('',*,*,#17556,.T.);
#23540=ORIENTED_EDGE('',*,*,#17560,.T.);
#23541=ORIENTED_EDGE('',*,*,#17561,.F.);
#23542=ORIENTED_EDGE('',*,*,#17432,.F.);
#23543=ORIENTED_EDGE('',*,*,#17560,.F.);
#23544=ORIENTED_EDGE('',*,*,#17557,.T.);
#23545=ORIENTED_EDGE('',*,*,#17559,.T.);
#23546=ORIENTED_EDGE('',*,*,#17562,.F.);
#23547=ORIENTED_EDGE('',*,*,#17558,.T.);
#23548=ORIENTED_EDGE('',*,*,#17399,.T.);
#23549=ORIENTED_EDGE('',*,*,#17563,.F.);
#23550=ORIENTED_EDGE('',*,*,#17564,.F.);
#23551=ORIENTED_EDGE('',*,*,#17561,.T.);
#23552=ORIENTED_EDGE('',*,*,#17565,.T.);
#23553=ORIENTED_EDGE('',*,*,#17566,.F.);
#23554=ORIENTED_EDGE('',*,*,#17433,.F.);
#23555=ORIENTED_EDGE('',*,*,#17565,.F.);
#23556=ORIENTED_EDGE('',*,*,#17562,.T.);
#23557=ORIENTED_EDGE('',*,*,#17564,.T.);
#23558=ORIENTED_EDGE('',*,*,#17567,.F.);
#23559=ORIENTED_EDGE('',*,*,#17563,.T.);
#23560=ORIENTED_EDGE('',*,*,#17398,.T.);
#23561=ORIENTED_EDGE('',*,*,#17568,.F.);
#23562=ORIENTED_EDGE('',*,*,#17569,.F.);
#23563=ORIENTED_EDGE('',*,*,#17566,.T.);
#23564=ORIENTED_EDGE('',*,*,#17570,.T.);
#23565=ORIENTED_EDGE('',*,*,#17571,.F.);
#23566=ORIENTED_EDGE('',*,*,#17434,.F.);
#23567=ORIENTED_EDGE('',*,*,#17570,.F.);
#23568=ORIENTED_EDGE('',*,*,#17567,.T.);
#23569=ORIENTED_EDGE('',*,*,#17569,.T.);
#23570=ORIENTED_EDGE('',*,*,#17572,.F.);
#23571=ORIENTED_EDGE('',*,*,#17568,.T.);
#23572=ORIENTED_EDGE('',*,*,#17397,.T.);
#23573=ORIENTED_EDGE('',*,*,#17573,.F.);
#23574=ORIENTED_EDGE('',*,*,#17574,.F.);
#23575=ORIENTED_EDGE('',*,*,#17571,.T.);
#23576=ORIENTED_EDGE('',*,*,#17575,.T.);
#23577=ORIENTED_EDGE('',*,*,#17576,.F.);
#23578=ORIENTED_EDGE('',*,*,#17435,.F.);
#23579=ORIENTED_EDGE('',*,*,#17575,.F.);
#23580=ORIENTED_EDGE('',*,*,#17572,.T.);
#23581=ORIENTED_EDGE('',*,*,#17574,.T.);
#23582=ORIENTED_EDGE('',*,*,#17577,.F.);
#23583=ORIENTED_EDGE('',*,*,#17573,.T.);
#23584=ORIENTED_EDGE('',*,*,#17396,.T.);
#23585=ORIENTED_EDGE('',*,*,#17535,.F.);
#23586=ORIENTED_EDGE('',*,*,#17578,.F.);
#23587=ORIENTED_EDGE('',*,*,#17576,.T.);
#23588=ORIENTED_EDGE('',*,*,#17579,.T.);
#23589=ORIENTED_EDGE('',*,*,#17538,.F.);
#23590=ORIENTED_EDGE('',*,*,#17436,.F.);
#23591=ORIENTED_EDGE('',*,*,#17579,.F.);
#23592=ORIENTED_EDGE('',*,*,#17577,.T.);
#23593=ORIENTED_EDGE('',*,*,#17578,.T.);
#23594=ORIENTED_EDGE('',*,*,#17541,.F.);
#23595=ORIENTED_EDGE('',*,*,#17580,.T.);
#23596=ORIENTED_EDGE('',*,*,#17581,.T.);
#23597=ORIENTED_EDGE('',*,*,#17582,.F.);
#23598=ORIENTED_EDGE('',*,*,#17392,.F.);
#23599=ORIENTED_EDGE('',*,*,#17583,.T.);
#23600=ORIENTED_EDGE('',*,*,#17420,.T.);
#23601=ORIENTED_EDGE('',*,*,#17584,.F.);
#23602=ORIENTED_EDGE('',*,*,#17585,.F.);
#23603=ORIENTED_EDGE('',*,*,#17585,.T.);
#23604=ORIENTED_EDGE('',*,*,#17586,.T.);
#23605=ORIENTED_EDGE('',*,*,#17581,.F.);
#23606=ORIENTED_EDGE('',*,*,#17587,.F.);
#23607=ORIENTED_EDGE('',*,*,#17588,.T.);
#23608=ORIENTED_EDGE('',*,*,#17589,.T.);
#23609=ORIENTED_EDGE('',*,*,#17580,.F.);
#23610=ORIENTED_EDGE('',*,*,#17391,.F.);
#23611=ORIENTED_EDGE('',*,*,#17590,.T.);
#23612=ORIENTED_EDGE('',*,*,#17421,.T.);
#23613=ORIENTED_EDGE('',*,*,#17583,.F.);
#23614=ORIENTED_EDGE('',*,*,#17591,.F.);
#23615=ORIENTED_EDGE('',*,*,#17591,.T.);
#23616=ORIENTED_EDGE('',*,*,#17587,.T.);
#23617=ORIENTED_EDGE('',*,*,#17589,.F.);
#23618=ORIENTED_EDGE('',*,*,#17592,.F.);
#23619=ORIENTED_EDGE('',*,*,#17593,.T.);
#23620=ORIENTED_EDGE('',*,*,#17594,.T.);
#23621=ORIENTED_EDGE('',*,*,#17588,.F.);
#23622=ORIENTED_EDGE('',*,*,#17390,.F.);
#23623=ORIENTED_EDGE('',*,*,#17595,.T.);
#23624=ORIENTED_EDGE('',*,*,#17422,.T.);
#23625=ORIENTED_EDGE('',*,*,#17590,.F.);
#23626=ORIENTED_EDGE('',*,*,#17596,.F.);
#23627=ORIENTED_EDGE('',*,*,#17596,.T.);
#23628=ORIENTED_EDGE('',*,*,#17592,.T.);
#23629=ORIENTED_EDGE('',*,*,#17594,.F.);
#23630=ORIENTED_EDGE('',*,*,#17597,.F.);
#23631=ORIENTED_EDGE('',*,*,#17598,.T.);
#23632=ORIENTED_EDGE('',*,*,#17599,.T.);
#23633=ORIENTED_EDGE('',*,*,#17593,.F.);
#23634=ORIENTED_EDGE('',*,*,#17389,.F.);
#23635=ORIENTED_EDGE('',*,*,#17600,.T.);
#23636=ORIENTED_EDGE('',*,*,#17423,.T.);
#23637=ORIENTED_EDGE('',*,*,#17595,.F.);
#23638=ORIENTED_EDGE('',*,*,#17601,.F.);
#23639=ORIENTED_EDGE('',*,*,#17601,.T.);
#23640=ORIENTED_EDGE('',*,*,#17597,.T.);
#23641=ORIENTED_EDGE('',*,*,#17599,.F.);
#23642=ORIENTED_EDGE('',*,*,#17602,.F.);
#23643=ORIENTED_EDGE('',*,*,#17603,.T.);
#23644=ORIENTED_EDGE('',*,*,#17604,.T.);
#23645=ORIENTED_EDGE('',*,*,#17598,.F.);
#23646=ORIENTED_EDGE('',*,*,#17388,.F.);
#23647=ORIENTED_EDGE('',*,*,#17605,.T.);
#23648=ORIENTED_EDGE('',*,*,#17424,.T.);
#23649=ORIENTED_EDGE('',*,*,#17600,.F.);
#23650=ORIENTED_EDGE('',*,*,#17606,.F.);
#23651=ORIENTED_EDGE('',*,*,#17606,.T.);
#23652=ORIENTED_EDGE('',*,*,#17602,.T.);
#23653=ORIENTED_EDGE('',*,*,#17604,.F.);
#23654=ORIENTED_EDGE('',*,*,#17607,.F.);
#23655=ORIENTED_EDGE('',*,*,#17608,.T.);
#23656=ORIENTED_EDGE('',*,*,#17609,.T.);
#23657=ORIENTED_EDGE('',*,*,#17603,.F.);
#23658=ORIENTED_EDGE('',*,*,#17387,.F.);
#23659=ORIENTED_EDGE('',*,*,#17610,.T.);
#23660=ORIENTED_EDGE('',*,*,#17425,.T.);
#23661=ORIENTED_EDGE('',*,*,#17605,.F.);
#23662=ORIENTED_EDGE('',*,*,#17611,.F.);
#23663=ORIENTED_EDGE('',*,*,#17611,.T.);
#23664=ORIENTED_EDGE('',*,*,#17607,.T.);
#23665=ORIENTED_EDGE('',*,*,#17609,.F.);
#23666=ORIENTED_EDGE('',*,*,#17612,.F.);
#23667=ORIENTED_EDGE('',*,*,#17613,.T.);
#23668=ORIENTED_EDGE('',*,*,#17614,.T.);
#23669=ORIENTED_EDGE('',*,*,#17608,.F.);
#23670=ORIENTED_EDGE('',*,*,#17386,.F.);
#23671=ORIENTED_EDGE('',*,*,#17615,.T.);
#23672=ORIENTED_EDGE('',*,*,#17426,.T.);
#23673=ORIENTED_EDGE('',*,*,#17610,.F.);
#23674=ORIENTED_EDGE('',*,*,#17616,.F.);
#23675=ORIENTED_EDGE('',*,*,#17616,.T.);
#23676=ORIENTED_EDGE('',*,*,#17612,.T.);
#23677=ORIENTED_EDGE('',*,*,#17614,.F.);
#23678=ORIENTED_EDGE('',*,*,#17617,.F.);
#23679=ORIENTED_EDGE('',*,*,#17618,.T.);
#23680=ORIENTED_EDGE('',*,*,#17619,.T.);
#23681=ORIENTED_EDGE('',*,*,#17613,.F.);
#23682=ORIENTED_EDGE('',*,*,#17385,.F.);
#23683=ORIENTED_EDGE('',*,*,#17620,.T.);
#23684=ORIENTED_EDGE('',*,*,#17427,.T.);
#23685=ORIENTED_EDGE('',*,*,#17615,.F.);
#23686=ORIENTED_EDGE('',*,*,#17621,.F.);
#23687=ORIENTED_EDGE('',*,*,#17621,.T.);
#23688=ORIENTED_EDGE('',*,*,#17617,.T.);
#23689=ORIENTED_EDGE('',*,*,#17619,.F.);
#23690=ORIENTED_EDGE('',*,*,#17622,.F.);
#23691=ORIENTED_EDGE('',*,*,#17623,.T.);
#23692=ORIENTED_EDGE('',*,*,#17624,.T.);
#23693=ORIENTED_EDGE('',*,*,#17618,.F.);
#23694=ORIENTED_EDGE('',*,*,#17384,.F.);
#23695=ORIENTED_EDGE('',*,*,#17625,.T.);
#23696=ORIENTED_EDGE('',*,*,#17428,.T.);
#23697=ORIENTED_EDGE('',*,*,#17620,.F.);
#23698=ORIENTED_EDGE('',*,*,#17626,.F.);
#23699=ORIENTED_EDGE('',*,*,#17626,.T.);
#23700=ORIENTED_EDGE('',*,*,#17622,.T.);
#23701=ORIENTED_EDGE('',*,*,#17624,.F.);
#23702=ORIENTED_EDGE('',*,*,#17627,.F.);
#23703=ORIENTED_EDGE('',*,*,#17628,.T.);
#23704=ORIENTED_EDGE('',*,*,#17629,.T.);
#23705=ORIENTED_EDGE('',*,*,#17623,.F.);
#23706=ORIENTED_EDGE('',*,*,#17383,.F.);
#23707=ORIENTED_EDGE('',*,*,#17630,.T.);
#23708=ORIENTED_EDGE('',*,*,#17429,.T.);
#23709=ORIENTED_EDGE('',*,*,#17625,.F.);
#23710=ORIENTED_EDGE('',*,*,#17631,.F.);
#23711=ORIENTED_EDGE('',*,*,#17631,.T.);
#23712=ORIENTED_EDGE('',*,*,#17627,.T.);
#23713=ORIENTED_EDGE('',*,*,#17629,.F.);
#23714=ORIENTED_EDGE('',*,*,#17632,.F.);
#23715=ORIENTED_EDGE('',*,*,#17582,.T.);
#23716=ORIENTED_EDGE('',*,*,#17633,.T.);
#23717=ORIENTED_EDGE('',*,*,#17628,.F.);
#23718=ORIENTED_EDGE('',*,*,#17393,.F.);
#23719=ORIENTED_EDGE('',*,*,#17584,.T.);
#23720=ORIENTED_EDGE('',*,*,#17419,.T.);
#23721=ORIENTED_EDGE('',*,*,#17630,.F.);
#23722=ORIENTED_EDGE('',*,*,#17634,.F.);
#23723=ORIENTED_EDGE('',*,*,#17634,.T.);
#23724=ORIENTED_EDGE('',*,*,#17632,.T.);
#23725=ORIENTED_EDGE('',*,*,#17633,.F.);
#23726=ORIENTED_EDGE('',*,*,#17586,.F.);
#32323=ADVANCED_FACE('',(#3575,#1262,#1263,#1264),#2121,.T.);
#32324=ADVANCED_FACE('',(#3576,#1265,#1266,#1267),#2122,.F.);
#32325=ADVANCED_FACE('',(#3577),#976,.T.);
#32326=ADVANCED_FACE('',(#3578),#977,.F.);
#32327=ADVANCED_FACE('',(#3579),#2608,.T.);
#32328=ADVANCED_FACE('',(#3580),#978,.T.);
#32329=ADVANCED_FACE('',(#3581),#979,.F.);
#32330=ADVANCED_FACE('',(#3582),#980,.F.);
#32331=ADVANCED_FACE('',(#3583),#981,.T.);
#32332=ADVANCED_FACE('',(#3584),#982,.F.);
#32333=ADVANCED_FACE('',(#3585),#983,.F.);
#32334=ADVANCED_FACE('',(#3586),#984,.T.);
#32335=ADVANCED_FACE('',(#3587),#985,.F.);
#32336=ADVANCED_FACE('',(#3588),#986,.F.);
#32337=ADVANCED_FACE('',(#3589),#987,.T.);
#32338=ADVANCED_FACE('',(#3590),#988,.F.);
#32339=ADVANCED_FACE('',(#3591),#989,.F.);
#32340=ADVANCED_FACE('',(#3592),#990,.T.);
#32341=ADVANCED_FACE('',(#3593),#991,.F.);
#32342=ADVANCED_FACE('',(#3594),#992,.F.);
#32343=ADVANCED_FACE('',(#3595),#993,.T.);
#32344=ADVANCED_FACE('',(#3596),#994,.F.);
#32345=ADVANCED_FACE('',(#3597),#995,.F.);
#32346=ADVANCED_FACE('',(#3598),#2609,.T.);
#32347=ADVANCED_FACE('',(#3599),#2610,.T.);
#32348=ADVANCED_FACE('',(#3600),#2123,.F.);
#32349=ADVANCED_FACE('',(#3601),#996,.T.);
#32350=ADVANCED_FACE('',(#3602),#997,.F.);
#32351=ADVANCED_FACE('',(#3603),#998,.F.);
#32352=ADVANCED_FACE('',(#3604),#999,.T.);
#32353=ADVANCED_FACE('',(#3605),#1000,.F.);
#32354=ADVANCED_FACE('',(#3606),#1001,.F.);
#32355=ADVANCED_FACE('',(#3607),#1002,.T.);
#32356=ADVANCED_FACE('',(#3608),#1003,.F.);
#32357=ADVANCED_FACE('',(#3609),#1004,.F.);
#32358=ADVANCED_FACE('',(#3610),#1005,.T.);
#32359=ADVANCED_FACE('',(#3611),#1006,.F.);
#32360=ADVANCED_FACE('',(#3612),#1007,.F.);
#32361=ADVANCED_FACE('',(#3613),#1008,.T.);
#32362=ADVANCED_FACE('',(#3614),#1009,.F.);
#32363=ADVANCED_FACE('',(#3615),#1010,.F.);
#32364=ADVANCED_FACE('',(#3616),#1011,.T.);
#32365=ADVANCED_FACE('',(#3617),#1012,.F.);
#32366=ADVANCED_FACE('',(#3618),#1013,.F.);
#32367=ADVANCED_FACE('',(#3619),#1014,.T.);
#32368=ADVANCED_FACE('',(#3620),#1015,.F.);
#32369=ADVANCED_FACE('',(#3621),#1016,.F.);
#32370=ADVANCED_FACE('',(#3622),#1017,.T.);
#32371=ADVANCED_FACE('',(#3623),#1018,.F.);
#32372=ADVANCED_FACE('',(#3624),#1019,.F.);
#32373=ADVANCED_FACE('',(#3625),#1020,.T.);
#32374=ADVANCED_FACE('',(#3626),#1021,.F.);
#32375=ADVANCED_FACE('',(#3627),#1022,.F.);
#32376=ADVANCED_FACE('',(#3628),#1023,.T.);
#32377=ADVANCED_FACE('',(#3629),#1024,.F.);
#32378=ADVANCED_FACE('',(#3630),#1025,.F.);
#32379=ADVANCED_FACE('',(#3631),#1026,.T.);
#32380=ADVANCED_FACE('',(#3632),#1027,.F.);
#32381=ADVANCED_FACE('',(#3633),#1028,.F.);
#32382=ADVANCED_FACE('',(#3634),#1029,.T.);
#32383=ADVANCED_FACE('',(#3635),#1030,.F.);
#32384=ADVANCED_FACE('',(#3636),#2611,.T.);
#32385=ADVANCED_FACE('',(#3637),#1031,.T.);
#32386=ADVANCED_FACE('',(#3638),#1032,.F.);
#32387=ADVANCED_FACE('',(#3639),#1033,.F.);
#32388=ADVANCED_FACE('',(#3640),#2612,.T.);
#32389=ADVANCED_FACE('',(#3641),#2613,.T.);
#32390=ADVANCED_FACE('',(#3642),#2124,.F.);
#32391=ADVANCED_FACE('',(#3643),#1034,.T.);
#32392=ADVANCED_FACE('',(#3644),#1035,.F.);
#32393=ADVANCED_FACE('',(#3645),#1036,.F.);
#32394=ADVANCED_FACE('',(#3646),#1037,.T.);
#32395=ADVANCED_FACE('',(#3647),#1038,.F.);
#32396=ADVANCED_FACE('',(#3648),#1039,.F.);
#32397=ADVANCED_FACE('',(#3649),#1040,.T.);
#32398=ADVANCED_FACE('',(#3650),#1041,.F.);
#32399=ADVANCED_FACE('',(#3651),#1042,.F.);
#32400=ADVANCED_FACE('',(#3652),#1043,.T.);
#32401=ADVANCED_FACE('',(#3653),#1044,.F.);
#32402=ADVANCED_FACE('',(#3654),#1045,.F.);
#32403=ADVANCED_FACE('',(#3655),#1046,.T.);
#32404=ADVANCED_FACE('',(#3656),#1047,.F.);
#32405=ADVANCED_FACE('',(#3657),#1048,.F.);
#32406=ADVANCED_FACE('',(#3658),#1049,.T.);
#32407=ADVANCED_FACE('',(#3659),#1050,.F.);
#32408=ADVANCED_FACE('',(#3660),#1051,.F.);
#32409=ADVANCED_FACE('',(#3661),#1052,.T.);
#32410=ADVANCED_FACE('',(#3662),#1053,.F.);
#32411=ADVANCED_FACE('',(#3663),#1054,.F.);
#32412=ADVANCED_FACE('',(#3664),#1055,.T.);
#32413=ADVANCED_FACE('',(#3665),#1056,.F.);
#32414=ADVANCED_FACE('',(#3666),#1057,.F.);
#32415=ADVANCED_FACE('',(#3667),#1058,.T.);
#32416=ADVANCED_FACE('',(#3668),#1059,.F.);
#32417=ADVANCED_FACE('',(#3669),#1060,.F.);
#32418=ADVANCED_FACE('',(#3670),#1061,.T.);
#32419=ADVANCED_FACE('',(#3671),#1062,.F.);
#32420=ADVANCED_FACE('',(#3672),#1063,.F.);
#32421=ADVANCED_FACE('',(#3673),#1064,.T.);
#32422=ADVANCED_FACE('',(#3674),#1065,.F.);
#32423=ADVANCED_FACE('',(#3675),#1066,.F.);
#32424=ADVANCED_FACE('',(#3676),#1067,.T.);
#32425=ADVANCED_FACE('',(#3677),#1068,.F.);
#32426=ADVANCED_FACE('',(#3678),#1069,.F.);
#32427=ADVANCED_FACE('',(#3679),#1070,.T.);
#32428=ADVANCED_FACE('',(#3680),#1071,.F.);
#32429=ADVANCED_FACE('',(#3681),#1072,.F.);
#32430=ADVANCED_FACE('',(#3682),#1073,.T.);
#32431=ADVANCED_FACE('',(#3683),#1074,.F.);
#32432=ADVANCED_FACE('',(#3684),#1075,.F.);
#34169=CLOSED_SHELL('',(#32323,#32324,#32325,#32326,#32327,#32328,#32329,
#32330,#32331,#32332,#32333,#32334,#32335,#32336,#32337,#32338,#32339,#32340,
#32341,#32342,#32343,#32344,#32345,#32346,#32347,#32348,#32349,#32350,#32351,
#32352,#32353,#32354,#32355,#32356,#32357,#32358,#32359,#32360,#32361,#32362,
#32363,#32364,#32365,#32366,#32367,#32368,#32369,#32370,#32371,#32372,#32373,
#32374,#32375,#32376,#32377,#32378,#32379,#32380,#32381,#32382,#32383,#32384,
#32385,#32386,#32387,#32388,#32389,#32390,#32391,#32392,#32393,#32394,#32395,
#32396,#32397,#32398,#32399,#32400,#32401,#32402,#32403,#32404,#32405,#32406,
#32407,#32408,#32409,#32410,#32411,#32412,#32413,#32414,#32415,#32416,#32417,
#32418,#32419,#32420,#32421,#32422,#32423,#32424,#32425,#32426,#32427,#32428,
#32429,#32430,#32431,#32432));
#34823=AXIS2_PLACEMENT_3D('',#57906,#39917,#39918);
#34824=AXIS2_PLACEMENT_3D('',#57907,#39919,#39920);
#34825=AXIS2_PLACEMENT_3D('',#58116,#39921,#39922);
#34826=AXIS2_PLACEMENT_3D('',#59282,#39923,#39924);
#34827=AXIS2_PLACEMENT_3D('',#59383,#39926,#39927);
#34828=AXIS2_PLACEMENT_3D('',#59537,#39928,#39929);
#34829=AXIS2_PLACEMENT_3D('',#59635,#39931,#39932);
#34830=AXIS2_PLACEMENT_3D('',#60368,#39933,#39934);
#34831=AXIS2_PLACEMENT_3D('',#60608,#39935,#39936);
#34832=AXIS2_PLACEMENT_3D('',#61448,#39937,#39938);
#34833=AXIS2_PLACEMENT_3D('',#61948,#39940,#39941);
#34834=AXIS2_PLACEMENT_3D('',#62762,#39942,#39943);
#34835=AXIS2_PLACEMENT_3D('',#63138,#39945,#39946);
#34836=AXIS2_PLACEMENT_3D('',#63451,#39947,#39948);
#34837=AXIS2_PLACEMENT_3D('',#63453,#39949,#39950);
#34838=AXIS2_PLACEMENT_3D('',#63454,#39951,#39952);
#34839=AXIS2_PLACEMENT_3D('',#63492,#39953,#39954);
#34840=AXIS2_PLACEMENT_3D('',#63494,#39955,#39956);
#34841=AXIS2_PLACEMENT_3D('',#63495,#39957,#39958);
#34842=AXIS2_PLACEMENT_3D('',#63496,#39959,#39960);
#34843=AXIS2_PLACEMENT_3D('',#63608,#39963,#39964);
#34844=AXIS2_PLACEMENT_3D('',#63863,#39965,#39966);
#34845=AXIS2_PLACEMENT_3D('',#63968,#39968,#39969);
#34846=AXIS2_PLACEMENT_3D('',#64088,#39970,#39971);
#34847=AXIS2_PLACEMENT_3D('',#64205,#39973,#39974);
#34848=AXIS2_PLACEMENT_3D('',#64421,#39975,#39976);
#34849=AXIS2_PLACEMENT_3D('',#64616,#39978,#39979);
#34850=AXIS2_PLACEMENT_3D('',#64880,#39980,#39981);
#34851=AXIS2_PLACEMENT_3D('',#64973,#39983,#39984);
#34852=AXIS2_PLACEMENT_3D('',#64974,#39985,#39986);
#34853=AXIS2_PLACEMENT_3D('',#65030,#39987,#39988);
#34854=AXIS2_PLACEMENT_3D('',#65031,#39989,#39990);
#34855=AXIS2_PLACEMENT_3D('',#65100,#39992,#39993);
#34856=AXIS2_PLACEMENT_3D('',#65171,#39994,#39995);
#34857=AXIS2_PLACEMENT_3D('',#65185,#39997,#39998);
#34858=AXIS2_PLACEMENT_3D('',#65219,#40000,#40001);
#34859=AXIS2_PLACEMENT_3D('',#65253,#40003,#40004);
#34860=AXIS2_PLACEMENT_3D('',#65495,#40006,#40007);
#34861=AXIS2_PLACEMENT_3D('',#65582,#40008,#40009);
#34862=AXIS2_PLACEMENT_3D('',#65674,#40012,#40013);
#34863=AXIS2_PLACEMENT_3D('',#65816,#40015,#40016);
#34864=AXIS2_PLACEMENT_3D('',#65982,#40017,#40018);
#34865=AXIS2_PLACEMENT_3D('',#66081,#40020,#40021);
#34866=AXIS2_PLACEMENT_3D('',#66341,#40023,#40024);
#34867=AXIS2_PLACEMENT_3D('',#66536,#40025,#40026);
#34868=AXIS2_PLACEMENT_3D('',#66629,#40028,#40029);
#34869=AXIS2_PLACEMENT_3D('',#66630,#40030,#40031);
#34870=AXIS2_PLACEMENT_3D('',#66686,#40032,#40033);
#34871=AXIS2_PLACEMENT_3D('',#66687,#40034,#40035);
#34872=AXIS2_PLACEMENT_3D('',#67044,#40037,#40038);
#34873=AXIS2_PLACEMENT_3D('',#67046,#40039,#40040);
#34874=AXIS2_PLACEMENT_3D('',#67144,#40041,#40042);
#34875=AXIS2_PLACEMENT_3D('',#67158,#40043,#40044);
#34876=AXIS2_PLACEMENT_3D('',#67264,#40047,#40048);
#34877=AXIS2_PLACEMENT_3D('',#67381,#40049,#40050);
#34878=AXIS2_PLACEMENT_3D('',#67516,#40052,#40053);
#34879=AXIS2_PLACEMENT_3D('',#67774,#40054,#40055);
#34880=AXIS2_PLACEMENT_3D('',#67879,#40057,#40058);
#34881=AXIS2_PLACEMENT_3D('',#67880,#40059,#40060);
#34882=AXIS2_PLACEMENT_3D('',#67918,#40061,#40062);
#34883=AXIS2_PLACEMENT_3D('',#67919,#40063,#40064);
#34884=AXIS2_PLACEMENT_3D('',#67920,#40065,#40066);
#34885=AXIS2_PLACEMENT_3D('',#68119,#40069,#40070);
#34886=AXIS2_PLACEMENT_3D('',#68121,#40071,#40072);
#34887=AXIS2_PLACEMENT_3D('',#68123,#40074,#40075);
#34888=AXIS2_PLACEMENT_3D('',#68126,#40077,#40078);
#34889=AXIS2_PLACEMENT_3D('',#68127,#40079,#40080);
#34890=AXIS2_PLACEMENT_3D('',#68184,#40082,#40083);
#34891=AXIS2_PLACEMENT_3D('',#68255,#40084,#40085);
#34892=AXIS2_PLACEMENT_3D('',#68324,#40087,#40088);
#34893=AXIS2_PLACEMENT_3D('',#68325,#40089,#40090);
#34894=AXIS2_PLACEMENT_3D('',#68381,#40091,#40092);
#34895=AXIS2_PLACEMENT_3D('',#68382,#40093,#40094);
#34896=AXIS2_PLACEMENT_3D('',#68796,#40096,#40097);
#34897=AXIS2_PLACEMENT_3D('',#68810,#40098,#40099);
#34898=AXIS2_PLACEMENT_3D('',#68884,#40100,#40101);
#34899=AXIS2_PLACEMENT_3D('',#68886,#40102,#40103);
#34900=AXIS2_PLACEMENT_3D('',#69007,#40106,#40107);
#34901=AXIS2_PLACEMENT_3D('',#69069,#40108,#40109);
#34902=AXIS2_PLACEMENT_3D('',#69181,#40111,#40112);
#34903=AXIS2_PLACEMENT_3D('',#69246,#40113,#40114);
#34904=AXIS2_PLACEMENT_3D('',#69321,#40116,#40117);
#34905=AXIS2_PLACEMENT_3D('',#69386,#40118,#40119);
#34906=AXIS2_PLACEMENT_3D('',#69461,#40121,#40122);
#34907=AXIS2_PLACEMENT_3D('',#69523,#40123,#40124);
#34908=AXIS2_PLACEMENT_3D('',#69653,#40126,#40127);
#34909=AXIS2_PLACEMENT_3D('',#69748,#40128,#40129);
#34910=AXIS2_PLACEMENT_3D('',#69904,#40131,#40132);
#34911=AXIS2_PLACEMENT_3D('',#70011,#40133,#40134);
#34912=AXIS2_PLACEMENT_3D('',#70315,#40136,#40137);
#34913=AXIS2_PLACEMENT_3D('',#70536,#40138,#40139);
#34914=AXIS2_PLACEMENT_3D('',#70710,#40141,#40142);
#34915=AXIS2_PLACEMENT_3D('',#70711,#40143,#40144);
#34916=AXIS2_PLACEMENT_3D('',#70767,#40145,#40146);
#34917=AXIS2_PLACEMENT_3D('',#70768,#40147,#40148);
#34918=AXIS2_PLACEMENT_3D('',#70963,#40150,#40151);
#34919=AXIS2_PLACEMENT_3D('',#71166,#40152,#40153);
#39917=DIRECTION('axis',(0.,0.,1.));
#39918=DIRECTION('refdir',(1.,0.,0.));
#39919=DIRECTION('center_axis',(0.,1.,0.));
#39920=DIRECTION('ref_axis',(1.,0.,0.));
#39921=DIRECTION('center_axis',(-4.53826900753912E-20,1.,-1.89783535791704E-12));
#39922=DIRECTION('ref_axis',(0.999999996595594,-1.56555493309401E-16,-8.25155224061155E-5));
#39923=DIRECTION('center_axis',(-3.6775085234444E-13,-1.,1.12427017219775E-12));
#39924=DIRECTION('ref_axis',(0.949453459673758,3.75489493260349E-15,0.313907833469525));
#39925=DIRECTION('',(6.70258519737E-14,0.,1.));
#39926=DIRECTION('center_axis',(1.50438405503027E-11,-1.,-7.96818632756709E-11));
#39927=DIRECTION('ref_axis',(0.982070554550592,-2.47012319048512E-13,0.188513728637183));
#39928=DIRECTION('center_axis',(0.,-1.,0.));
#39929=DIRECTION('ref_axis',(0.983200783709105,0.,-0.182527310049212));
#39930=DIRECTION('',(5.34758952088E-14,0.,-1.));
#39931=DIRECTION('center_axis',(4.23985864404906E-13,-1.,1.28365524709865E-12));
#39932=DIRECTION('ref_axis',(0.949639883258862,4.08975341799599E-16,-0.313343409255875));
#39933=DIRECTION('center_axis',(0.,1.,0.));
#39934=DIRECTION('ref_axis',(0.99999996092868,0.,0.000279540048092856));
#39935=DIRECTION('center_axis',(0.,1.,0.));
#39936=DIRECTION('ref_axis',(1.,0.,0.));
#39937=DIRECTION('center_axis',(0.,1.,0.));
#39938=DIRECTION('ref_axis',(0.999999972082516,0.,-0.000236294239609272));
#39939=DIRECTION('',(6.51345827468E-14,0.,1.));
#39940=DIRECTION('center_axis',(0.,-1.,0.));
#39941=DIRECTION('ref_axis',(0.94940501112193,0.,0.31405433424261));
#39942=DIRECTION('center_axis',(0.,-1.,0.));
#39943=DIRECTION('ref_axis',(0.949684781053655,0.,-0.313207306164895));
#39944=DIRECTION('',(5.92102704963E-14,0.,-1.));
#39945=DIRECTION('center_axis',(0.,1.,0.));
#39946=DIRECTION('ref_axis',(0.999999881236024,0.,0.000487368379934368));
#39947=DIRECTION('center_axis',(-0.981439111391386,-6.91947304276285E-7,
0.19177400926822));
#39948=DIRECTION('ref_axis',(0.135605174340565,-0.707106824297193,0.693982114844759));
#39949=DIRECTION('center_axis',(-0.983800902348753,2.55819041831388E-6,
0.179264565743584));
#39950=DIRECTION('ref_axis',(0.126757816828919,-0.707104514303595,0.695654843815698));
#39951=DIRECTION('center_axis',(0.,-1.,0.));
#39952=DIRECTION('ref_axis',(0.982643704634813,0.,-0.185502964239308));
#39953=DIRECTION('center_axis',(-0.981438226141561,-7.89143835502642E-7,
0.191778539642689));
#39954=DIRECTION('ref_axis',(-0.13560735839919,-0.70710678023174,-0.693981732971621));
#39955=DIRECTION('center_axis',(0.,-1.,0.));
#39956=DIRECTION('ref_axis',(0.982643702177,0.,-0.185502977258799));
#39957=DIRECTION('center_axis',(-0.983803848856482,2.10287653257285E-5,
0.179248393390189));
#39958=DIRECTION('ref_axis',(0.126755899045361,0.707142957839062,0.695616114847712));
#39959=DIRECTION('center_axis',(0.,1.,0.));
#39960=DIRECTION('ref_axis',(0.185521087284598,0.,0.98264028320273));
#39961=DIRECTION('',(0.,1.,0.));
#39962=DIRECTION('',(0.,1.,0.));
#39963=DIRECTION('center_axis',(0.154836917217659,-3.12361430976921E-6,
0.987940043249981));
#39964=DIRECTION('ref_axis',(0.698580542308629,-0.707104979136634,-0.109488695251894));
#39965=DIRECTION('center_axis',(0.154845223447756,-1.35064972128871E-7,
0.98793874140829));
#39966=DIRECTION('ref_axis',(-0.698578109459083,-0.707106871046533,0.109491999266408));
#39967=DIRECTION('',(0.,1.,0.));
#39968=DIRECTION('center_axis',(0.520972865596847,1.69414956570985E-6,0.853573238397819));
#39969=DIRECTION('ref_axis',(0.603568577001839,-0.707106162849763,-0.368382745681526));
#39970=DIRECTION('center_axis',(0.520969134614679,-1.13333766643287E-11,
0.85357551556897));
#39971=DIRECTION('ref_axis',(0.603569036189203,0.707106780165659,-0.368380808399938));
#39972=DIRECTION('',(0.,1.,0.));
#39973=DIRECTION('center_axis',(0.473837063552872,-1.24145995566389E-6,
-0.880612535228775));
#39974=DIRECTION('ref_axis',(0.622687803281783,0.707106449521282,0.335052784930248));
#39975=DIRECTION('center_axis',(0.473828846366866,-2.37517960535292E-6,
-0.88061695665312));
#39976=DIRECTION('ref_axis',(-0.622690007725239,0.707106120461181,-0.335049382457988));
#39977=DIRECTION('',(0.,1.,0.));
#39978=DIRECTION('center_axis',(0.904703679923686,3.52343105396791E-6,-0.426041373014554));
#39979=DIRECTION('ref_axis',(0.301254485151548,0.70710679235048,0.639723158395795));
#39980=DIRECTION('center_axis',(0.904707515904337,-3.36627255552488E-8,
-0.42603322718563));
#39981=DIRECTION('ref_axis',(0.301250989895463,-0.707106716692524,0.639724887975543));
#39982=DIRECTION('',(0.,1.,0.));
#39983=DIRECTION('center_axis',(0.980476419194366,4.59982314936753E-7,-0.196636699025342));
#39984=DIRECTION('ref_axis',(0.139042808353642,0.70710686281341,0.693301508730011));
#39985=DIRECTION('center_axis',(0.,-1.,0.));
#39986=DIRECTION('ref_axis',(0.949544989671707,0.,-0.313630854013693));
#39987=DIRECTION('center_axis',(0.,-1.,0.));
#39988=DIRECTION('ref_axis',(0.949544989671193,0.,-0.313630854015248));
#39989=DIRECTION('center_axis',(0.980477123615918,9.28542161123966E-7,-0.196633186580987));
#39990=DIRECTION('ref_axis',(0.139041425768334,-0.707106158854598,0.693302503983798));
#39991=DIRECTION('',(0.,1.,0.));
#39992=DIRECTION('center_axis',(-1.01620465039977E-5,4.17131142926177E-6,
-0.999999999939666));
#39993=DIRECTION('ref_axis',(0.707097475073845,0.707116087164088,-4.23595600861289E-6));
#39994=DIRECTION('center_axis',(-9.12499515000718E-8,-3.77832852281249E-8,
-0.999999999999995));
#39995=DIRECTION('ref_axis',(0.70710678547465,-0.707106776898444,-3.78066428416396E-8));
#39996=DIRECTION('',(2.51386213433E-14,1.,0.));
#39997=DIRECTION('center_axis',(5.34758952088E-14,0.,-1.));
#39998=DIRECTION('ref_axis',(-1.,2.31296463463574E-14,-5.34758952088E-14));
#39999=DIRECTION('',(5.3463780235E-14,0.,-1.));
#40000=DIRECTION('center_axis',(5.92118946467E-14,-1.35858726807196E-28,
-1.));
#40001=DIRECTION('ref_axis',(5.42101086242749E-16,-1.,1.67957559213664E-28));
#40002=DIRECTION('',(5.3463780235E-14,0.,-1.));
#40003=DIRECTION('center_axis',(1.,-2.51304279671E-14,5.34739473113E-14));
#40004=DIRECTION('ref_axis',(-5.34739473113E-14,0.,1.));
#40005=DIRECTION('',(0.,1.,0.));
#40006=DIRECTION('center_axis',(0.0335673088203785,9.76784545296555E-7,
0.999436459099628));
#40007=DIRECTION('ref_axis',(0.706708319465629,-0.707106782500715,-0.0237349813472152));
#40008=DIRECTION('center_axis',(0.033571208573789,-2.79700859966269E-6,
0.999436328110537));
#40009=DIRECTION('ref_axis',(0.70670899253357,0.707106059613177,-0.0237364767923099));
#40010=DIRECTION('',(0.,1.,0.));
#40011=DIRECTION('',(0.,1.,0.));
#40012=DIRECTION('center_axis',(0.999999978084788,-0.000101096238990269,
0.000183330234716788));
#40013=DIRECTION('ref_axis',(5.81481962535521E-5,-0.707106853629676,-0.707106706352533));
#40014=DIRECTION('',(0.,1.,0.));
#40015=DIRECTION('center_axis',(0.0335656369607943,-6.36312949534584E-7,
-0.999436515249974));
#40016=DIRECTION('ref_axis',(0.706708024598012,0.707107109174478,0.0237340288128194));
#40017=DIRECTION('center_axis',(0.0335621289194674,1.19749411790846E-10,
-0.999436633060042));
#40018=DIRECTION('ref_axis',(-0.706708201393549,0.707107000522345,-0.023732001504006));
#40019=DIRECTION('',(0.,1.,0.));
#40020=DIRECTION('center_axis',(-0.296880383254147,-5.5879869627127E-5,
-0.954914674154875));
#40021=DIRECTION('ref_axis',(0.675214504950974,0.707107206299133,-0.209963737592105));
#40022=DIRECTION('',(0.,1.,0.));
#40023=DIRECTION('center_axis',(-0.97943439723664,1.88767156221692E-7,-0.201762884370897));
#40024=DIRECTION('ref_axis',(0.142668223249667,0.707105845503049,-0.692565593521799));
#40025=DIRECTION('center_axis',(-0.979434890534362,-1.13639773389063E-6,
-0.201760489696696));
#40026=DIRECTION('ref_axis',(0.142667101613083,-0.707106265008557,-0.692565396264476));
#40027=DIRECTION('',(0.,1.,0.));
#40028=DIRECTION('center_axis',(-0.979434533515105,-4.50567798853205E-7,
0.201762222821431));
#40029=DIRECTION('ref_axis',(0.142667769468626,-0.707106674739596,0.692564840353275));
#40030=DIRECTION('center_axis',(0.,1.,0.));
#40031=DIRECTION('ref_axis',(1.,0.,4.53995751566807E-15));
#40032=DIRECTION('center_axis',(0.,1.,0.));
#40033=DIRECTION('ref_axis',(1.,0.,-1.77342090453718E-17));
#40034=DIRECTION('center_axis',(-0.979433511432438,-1.51283178385928E-6,
0.201767184350767));
#40035=DIRECTION('ref_axis',(-0.142669686404077,-0.707107822666436,-0.692563273430879));
#40036=DIRECTION('',(0.,1.,0.));
#40037=DIRECTION('center_axis',(0.473835002614585,-4.38921425069636E-12,
0.880613644169358));
#40038=DIRECTION('ref_axis',(0.62268754361935,-0.70710716248492,-0.335051762842439));
#40039=DIRECTION('center_axis',(0.520966517709422,1.18825474124969E-6,-0.853577112758014));
#40040=DIRECTION('ref_axis',(0.603569632363666,0.707106892020158,0.368379616898087));
#40041=DIRECTION('center_axis',(0.473834278771671,2.54149984160096E-8,0.880614033649777));
#40042=DIRECTION('ref_axis',(-0.622688145028847,-0.707106782614661,0.335051446827015));
#40043=DIRECTION('center_axis',(0.520965370835567,-1.29982441725717E-6,
-0.853577812732074));
#40044=DIRECTION('ref_axis',(-0.603570181217405,0.707106780728377,-0.368378931255765));
#40045=DIRECTION('',(0.,1.,0.));
#40046=DIRECTION('',(0.,1.,0.));
#40047=DIRECTION('center_axis',(0.154843595557673,1.07297464218487E-6,-0.987938996554757));
#40048=DIRECTION('ref_axis',(0.698578639261851,0.707106383509641,0.109491767576273));
#40049=DIRECTION('center_axis',(0.1548978156336,3.28185673290842E-5,-0.987930496358363));
#40050=DIRECTION('ref_axis',(-0.698568936199091,0.707113878525059,-0.109505270078283));
#40051=DIRECTION('',(0.,1.,0.));
#40052=DIRECTION('center_axis',(-0.983798505452903,-7.41074738031404E-6,
-0.179277719233919));
#40053=DIRECTION('ref_axis',(0.12676491018783,0.707097999012039,-0.695660173747384));
#40054=DIRECTION('center_axis',(-0.983801593483001,7.34382161735624E-7,
-0.17926077278582));
#40055=DIRECTION('ref_axis',(-0.126755910682294,0.70710726361168,0.695652396570805));
#40056=DIRECTION('',(0.,1.,0.));
#40057=DIRECTION('center_axis',(-0.981439661906731,1.44249277216099E-6,
-0.191771191878033));
#40058=DIRECTION('ref_axis',(0.135603711019434,0.707106782535524,-0.693982443329813));
#40059=DIRECTION('center_axis',(0.,-1.,0.));
#40060=DIRECTION('ref_axis',(0.982642715024755,0.,0.185508206311143));
#40061=DIRECTION('center_axis',(0.,-1.,0.));
#40062=DIRECTION('ref_axis',(0.982642715024755,0.,0.185508206311143));
#40063=DIRECTION('center_axis',(-0.981441652211516,-4.67297560071752E-6,
-0.191761005635902));
#40064=DIRECTION('ref_axis',(0.135598750250042,-0.707106782087573,-0.69398341309889));
#40065=DIRECTION('center_axis',(0.,1.,0.));
#40066=DIRECTION('ref_axis',(-0.185521087269691,0.,0.982640283205544));
#40067=DIRECTION('',(0.,1.,0.));
#40068=DIRECTION('',(-5.31321018928E-14,1.,0.));
#40069=DIRECTION('center_axis',(6.70258519737E-14,-4.98239453982157E-43,
1.));
#40070=DIRECTION('ref_axis',(1.,4.62592926927149E-14,-6.70258519737E-14));
#40071=DIRECTION('center_axis',(-1.10324427504723E-11,-1.10324427504724E-11,
1.));
#40072=DIRECTION('ref_axis',(0.707106778746433,-0.707106783626662,-5.38408906596044E-20));
#40073=DIRECTION('',(6.70203270059E-14,0.,1.));
#40074=DIRECTION('center_axis',(6.51330841113E-14,-8.98109190113476E-29,
1.));
#40075=DIRECTION('ref_axis',(-7.22801448323666E-16,-1.,-4.27326314819128E-29));
#40076=DIRECTION('',(6.70203270059E-14,0.,1.));
#40077=DIRECTION('center_axis',(-7.94004949271736E-11,7.94004949271753E-11,
1.));
#40078=DIRECTION('ref_axis',(-0.707106780907752,-0.707106781465343,4.42741533183115E-20));
#40079=DIRECTION('center_axis',(-1.,-5.30625513235E-14,6.70263256881E-14));
#40080=DIRECTION('ref_axis',(-5.30625513235E-14,1.,-1.81689879574742E-43));
#40081=DIRECTION('',(0.,1.,0.));
#40082=DIRECTION('center_axis',(0.980478566353175,3.7723498926218E-6,0.196625992452148));
#40083=DIRECTION('ref_axis',(0.139037044282546,-0.707112597974319,-0.693296815298601));
#40084=DIRECTION('center_axis',(0.980476663067875,-1.6843586153538E-12,
0.196635483011803));
#40085=DIRECTION('ref_axis',(0.139042284163302,0.70710677761346,-0.693301700753547));
#40086=DIRECTION('',(0.,1.,0.));
#40087=DIRECTION('center_axis',(0.904708058486416,4.59948929901095E-7,0.426032074977376));
#40088=DIRECTION('ref_axis',(0.301250429246376,-0.707106861495181,-0.639724991934275));
#40089=DIRECTION('center_axis',(0.,-1.,0.));
#40090=DIRECTION('ref_axis',(0.949544989671187,0.,0.313630854015266));
#40091=DIRECTION('center_axis',(0.,-1.,0.));
#40092=DIRECTION('ref_axis',(0.949544989671187,0.,0.313630854015266));
#40093=DIRECTION('center_axis',(0.904706532331394,9.28476887061025E-7,0.426035315855436));
#40094=DIRECTION('ref_axis',(-0.301252132655329,-0.707106157393727,0.639724968049938));
#40095=DIRECTION('',(0.,1.,0.));
#40096=DIRECTION('center_axis',(0.831646496536582,-3.85743040235925E-7,
0.555305415783314));
#40097=DIRECTION('ref_axis',(-0.392659665147305,-0.707108198105435,0.588061547406809));
#40098=DIRECTION('center_axis',(0.520955689889625,-6.10489755846883E-6,
-0.853583721221507));
#40099=DIRECTION('ref_axis',(-0.603570886687802,0.70710877515402,-0.368373947019984));
#40100=DIRECTION('center_axis',(0.831646480866685,3.73065313146438E-7,0.555305439251157));
#40101=DIRECTION('ref_axis',(0.392659054445677,-0.707109314315335,-0.588060613007131));
#40102=DIRECTION('center_axis',(0.520969129687222,5.06965085525085E-8,-0.85357551857638));
#40103=DIRECTION('ref_axis',(0.603569010894602,0.707106790406539,0.368380830186201));
#40104=DIRECTION('',(0.,1.,0.));
#40105=DIRECTION('',(0.,1.,0.));
#40106=DIRECTION('center_axis',(-0.160486455919009,-1.14494809085679E-8,
-0.987038042562978));
#40107=DIRECTION('ref_axis',(-0.697941290843371,0.707106784875672,0.113481052685807));
#40108=DIRECTION('center_axis',(-0.160486595636023,6.52250457089104E-13,
-0.987038019845821));
#40109=DIRECTION('ref_axis',(0.697941276113114,0.707106782208678,-0.113481159899282));
#40110=DIRECTION('',(0.,1.,0.));
#40111=DIRECTION('center_axis',(0.999999997768984,-1.78060155735714E-9,
6.67984466585521E-5));
#40112=DIRECTION('ref_axis',(4.72348957176867E-5,0.707106750687066,-0.707106810108377));
#40113=DIRECTION('center_axis',(0.999999997862801,4.18017746208693E-16,
6.53788750221213E-5));
#40114=DIRECTION('ref_axis',(4.6229822268084E-5,-0.707107142261732,-0.707106418599952));
#40115=DIRECTION('',(0.,1.,0.));
#40116=DIRECTION('center_axis',(-0.160485631761041,-3.83256429423384E-7,
0.987038176565685));
#40117=DIRECTION('ref_axis',(-0.697939946398453,-0.707108197591881,-0.113480518679139));
#40118=DIRECTION('center_axis',(-0.160485659064817,3.71132526604556E-7,
0.987038172126283));
#40119=DIRECTION('ref_axis',(0.697938843129776,-0.707109313555971,0.11348035042717));
#40120=DIRECTION('',(0.,1.,0.));
#40121=DIRECTION('center_axis',(0.831647339569147,-2.01970215594345E-7,
-0.555304153223726));
#40122=DIRECTION('ref_axis',(-0.392659211278407,0.70710678535694,-0.58806354920229));
#40123=DIRECTION('center_axis',(0.831642793947518,2.20503061757152E-6,-0.555310960877151));
#40124=DIRECTION('ref_axis',(0.392662307348694,0.707107757326728,0.588060313161809));
#40125=DIRECTION('',(0.,1.,0.));
#40126=DIRECTION('center_axis',(0.52097569735597,-2.97995712518636E-6,0.853571510042117));
#40127=DIRECTION('ref_axis',(0.603567201195272,0.707106897821364,-0.368383589068178));
#40128=DIRECTION('center_axis',(0.520966807973242,-7.72496346239503E-7,
0.853576935600755));
#40129=DIRECTION('ref_axis',(0.603569754740143,-0.707106781322477,-0.368379628875825));
#40130=DIRECTION('',(0.,1.,0.));
#40131=DIRECTION('center_axis',(0.154844796216802,-8.97906301415941E-8,
0.987938808370523));
#40132=DIRECTION('ref_axis',(-0.698578220064376,-0.707106802000707,0.109491739487604));
#40133=DIRECTION('center_axis',(0.154844863297137,1.72305380745362E-8,0.987938797856674));
#40134=DIRECTION('ref_axis',(0.698578206815753,-0.707106799844172,-0.109491837943393));
#40135=DIRECTION('',(0.,1.,0.));
#40136=DIRECTION('center_axis',(-0.990334650762026,-1.38749992122331E-10,
0.138698520179765));
#40137=DIRECTION('ref_axis',(0.0980746699601121,0.707106738665372,0.700272389321638));
#40138=DIRECTION('center_axis',(-0.990334159630947,1.08015952695937E-6,
0.138702026902633));
#40139=DIRECTION('ref_axis',(0.098076591555837,-0.707105309160556,0.700273563649053));
#40140=DIRECTION('',(0.,1.,0.));
#40141=DIRECTION('center_axis',(-0.990334489416453,-4.27056810582187E-7,
-0.138699672213279));
#40142=DIRECTION('ref_axis',(0.0980757788219265,-0.707106774008865,-0.700272198333797));
#40143=DIRECTION('center_axis',(0.,1.,0.));
#40144=DIRECTION('ref_axis',(1.,0.,5.1304900982414E-15));
#40145=DIRECTION('center_axis',(-0.990345075157185,2.9441547790821E-5,-0.138624064451688));
#40146=DIRECTION('ref_axis',(0.0980424742908994,0.707107928682427,-0.700275696015052));
#40147=DIRECTION('center_axis',(0.,1.,0.));
#40148=DIRECTION('ref_axis',(1.,0.,1.00009553569338E-17));
#40149=DIRECTION('',(0.,1.,0.));
#40150=DIRECTION('center_axis',(0.154794000275648,-2.07516415067679E-5,
-0.987946768327136));
#40151=DIRECTION('ref_axis',(-0.698579366791292,0.707109029425635,-0.109470036074784));
#40152=DIRECTION('center_axis',(0.154851124507597,-3.12677899154245E-6,
-0.987937816478829));
#40153=DIRECTION('ref_axis',(0.698577610398848,0.707107045772696,0.109494054943846));
#40154=DIRECTION('',(0.,1.,0.));
#57906=CARTESIAN_POINT('',(0.,0.,0.));
#57907=CARTESIAN_POINT('Origin',(-3.35265884719E-30,-36.2742356128,3.15283103411E-22));
#57908=CARTESIAN_POINT('',(10.7486851001341,-36.2742356128,0.754201403925636));
#57909=CARTESIAN_POINT('',(1.34538289151,-36.2742356128,-9.83573536665));
#57910=CARTESIAN_POINT('Ctrl Pts',(10.7486858765334,-36.2742356128,0.754196450359814));
#57911=CARTESIAN_POINT('Ctrl Pts',(10.7489629244814,-36.2742356128,0.752428733958977));
#57912=CARTESIAN_POINT('Ctrl Pts',(10.7492374499617,-36.2742356128,0.750675177529054));
#57913=CARTESIAN_POINT('Ctrl Pts',(10.7495128278646,-36.2742356128,0.748914143783128));
#57914=CARTESIAN_POINT('Ctrl Pts',(10.7507758135579,-36.2742356128,0.74083738670444));
#57915=CARTESIAN_POINT('Ctrl Pts',(10.7520323311518,-36.2742356128,0.73275908912306));
#57916=CARTESIAN_POINT('Ctrl Pts',(10.7532823709248,-36.2742356128,0.724679179487232));
#57917=CARTESIAN_POINT('Ctrl Pts',(10.7678711925259,-36.2742356128005,0.630381091716242));
#57918=CARTESIAN_POINT('Ctrl Pts',(10.7815770251776,-36.2742356128038,0.535855381856853));
#57919=CARTESIAN_POINT('Ctrl Pts',(10.7943682424213,-36.2742356128065,0.441041993340083));
#57920=CARTESIAN_POINT('Ctrl Pts',(10.8075688570078,-36.2742356128093,0.343193995326961));
#57921=CARTESIAN_POINT('Ctrl Pts',(10.8197950578014,-36.2742356128115,0.245039728220827));
#57922=CARTESIAN_POINT('Ctrl Pts',(10.8309655494112,-36.2742356128255,0.146545962675994));
#57923=CARTESIAN_POINT('Ctrl Pts',(10.8427480065759,-36.2742356128402,0.0426563028413041));
#57924=CARTESIAN_POINT('Ctrl Pts',(10.8533556511679,-36.2742356128608,-0.0616110371222863));
#57925=CARTESIAN_POINT('Ctrl Pts',(10.8626464096652,-36.2742356129736,-0.166260199650818));
#57926=CARTESIAN_POINT('Ctrl Pts',(10.8657801493804,-36.2742356130117,-0.201557989048003));
#57927=CARTESIAN_POINT('Ctrl Pts',(10.8687637124405,-36.2742356130614,-0.236898940796127));
#57928=CARTESIAN_POINT('Ctrl Pts',(10.8715906326909,-36.274235613131,-0.272282403346824));
#57929=CARTESIAN_POINT('Ctrl Pts',(10.8812699153207,-36.2742356133694,-0.393434223744914));
#57930=CARTESIAN_POINT('Ctrl Pts',(10.8891344949282,-36.2742356141013,-0.515016935053823));
#57931=CARTESIAN_POINT('Ctrl Pts',(10.8948762742751,-36.2742356281832,-0.636806406497127));
#57932=CARTESIAN_POINT('Ctrl Pts',(10.8963186883058,-36.2742356317208,-0.66740159864657));
#57933=CARTESIAN_POINT('Ctrl Pts',(10.8976270296754,-36.2742356361001,-0.698009597208687));
#57934=CARTESIAN_POINT('Ctrl Pts',(10.8987962631872,-36.2742356414173,-0.728626390660339));
#57935=CARTESIAN_POINT('Ctrl Pts',(10.9038986843607,-36.2742356646208,-0.862235095504958));
#57936=CARTESIAN_POINT('Ctrl Pts',(10.9063461028681,-36.2742357053368,-0.99603469063249));
#57937=CARTESIAN_POINT('Ctrl Pts',(10.905701363612,-36.2742357223532,-1.12991502257281));
#57938=CARTESIAN_POINT('Ctrl Pts',(10.905610239575,-36.2742357247582,-1.14883696070543));
#57939=CARTESIAN_POINT('Ctrl Pts',(10.9054573112217,-36.274235726648,-1.167760435996));
#57940=CARTESIAN_POINT('Ctrl Pts',(10.9052413159717,-36.2742357279012,-1.18668506610303));
#57941=CARTESIAN_POINT('Ctrl Pts',(10.9036142484637,-36.2742357373409,-1.32924213971618));
#57942=CARTESIAN_POINT('Ctrl Pts',(10.8984251378642,-36.2742357268193,-1.47186368584055));
#57943=CARTESIAN_POINT('Ctrl Pts',(10.8892016012729,-36.2742357087315,-1.61424401603744));
#57944=CARTESIAN_POINT('Ctrl Pts',(10.8815756184603,-36.2742356937766,-1.73196349816884));
#57945=CARTESIAN_POINT('Ctrl Pts',(10.8711911520625,-36.2742356745366,-1.84951690288712));
#57946=CARTESIAN_POINT('Ctrl Pts',(10.8578169153327,-36.2742356586438,-1.96672376842866));
#57947=CARTESIAN_POINT('Ctrl Pts',(10.8453069774373,-36.2742356437781,-2.07635623856265));
#57948=CARTESIAN_POINT('Ctrl Pts',(10.8301806199933,-36.274235631925,-2.18568500938683));
#57949=CARTESIAN_POINT('Ctrl Pts',(10.8122909632233,-36.2742356246492,-2.29456528269846));
#57950=CARTESIAN_POINT('Ctrl Pts',(10.7957295635652,-36.2742356179135,-2.39536149943887));
#57951=CARTESIAN_POINT('Ctrl Pts',(10.7767997912498,-36.2742356149251,-2.49577308102596));
#57952=CARTESIAN_POINT('Ctrl Pts',(10.7554275183188,-36.2742356137244,-2.59569279244582));
#57953=CARTESIAN_POINT('Ctrl Pts',(10.7350120113479,-36.2742356125775,-2.69113942891732));
#57954=CARTESIAN_POINT('Ctrl Pts',(10.7123675696945,-36.2742356128,-2.78613705522593));
#57955=CARTESIAN_POINT('Ctrl Pts',(10.6874728382363,-36.2742356128,-2.88060265456909));
#57956=CARTESIAN_POINT('Ctrl Pts',(10.6628505227107,-36.2742356128,-2.97403454385301));
#57957=CARTESIAN_POINT('Ctrl Pts',(10.6360194039611,-36.2742356128,-3.06693894766016));
#57958=CARTESIAN_POINT('Ctrl Pts',(10.6069482491376,-36.2742356128,-3.15920931784575));
#57959=CARTESIAN_POINT('Ctrl Pts',(10.5762645045941,-36.2742356128,-3.2565979659714));
#57960=CARTESIAN_POINT('Ctrl Pts',(10.5430855146013,-36.2742356128,-3.35327963951917));
#57961=CARTESIAN_POINT('Ctrl Pts',(10.5074324792489,-36.2742356128003,-3.44913299552277));
#57962=CARTESIAN_POINT('Ctrl Pts',(10.4698050071003,-36.2742356128006,-3.55029463429309));
#57963=CARTESIAN_POINT('Ctrl Pts',(10.4294222890416,-36.2742356128012,-3.65053271747348));
#57964=CARTESIAN_POINT('Ctrl Pts',(10.3863673413088,-36.2742356128042,-3.74972158036864));
#57965=CARTESIAN_POINT('Ctrl Pts',(10.3433123935759,-36.2742356128072,-3.8489104432638));
#57966=CARTESIAN_POINT('Ctrl Pts',(10.2975862065294,-36.2742356128123,-3.94704921131114));
#57967=CARTESIAN_POINT('Ctrl Pts',(10.2493168210226,-36.2742356128257,-4.04404255191892));
#57968=CARTESIAN_POINT('Ctrl Pts',(10.200143434872,-36.2742356128393,-4.14285240710298));
#57969=CARTESIAN_POINT('Ctrl Pts',(10.1483512913797,-36.2742356129685,-4.24044318113654));
#57970=CARTESIAN_POINT('Ctrl Pts',(10.0940811009206,-36.2742356129563,-4.33679486057107));
#57971=CARTESIAN_POINT('Ctrl Pts',(10.0860953319727,-36.2742356129545,-4.35097285116214));
#57972=CARTESIAN_POINT('Ctrl Pts',(10.078055934547,-36.2742356129488,-4.36512410006593));
#57973=CARTESIAN_POINT('Ctrl Pts',(10.069963381529,-36.2742356129389,-4.37924863866557));
#57974=CARTESIAN_POINT('Ctrl Pts',(10.0206103075602,-36.274235612879,-4.46538825328766));
#57975=CARTESIAN_POINT('Ctrl Pts',(9.96927479557785,-36.2742356128063,-4.55054423432799));
#57976=CARTESIAN_POINT('Ctrl Pts',(9.91611980874301,-36.2742356128011,-4.63468661170844));
#57977=CARTESIAN_POINT('Ctrl Pts',(9.90132634625179,-36.2742356127997,-4.65810411546152));
#57978=CARTESIAN_POINT('Ctrl Pts',(9.88639201933375,-36.2742356128,-4.681443411214));
#57979=CARTESIAN_POINT('Ctrl Pts',(9.87132045450753,-36.2742356128,-4.70470457439913));
#57980=CARTESIAN_POINT('Ctrl Pts',(9.81905209423248,-36.2742356128,-4.7853745560365));
#57981=CARTESIAN_POINT('Ctrl Pts',(9.76511812234536,-36.2742356128,-4.86512219137804));
#57982=CARTESIAN_POINT('Ctrl Pts',(9.70971375293503,-36.2742356128,-4.94390068743296));
#57983=CARTESIAN_POINT('Ctrl Pts',(9.65177867900376,-36.2742356128,-5.02627754762849));
#57984=CARTESIAN_POINT('Ctrl Pts',(9.59223559676037,-36.2742356128,-5.1075953157557));
#57985=CARTESIAN_POINT('Ctrl Pts',(9.53126893611934,-36.2742356128,-5.18784861358279));
#57986=CARTESIAN_POINT('Ctrl Pts',(9.47173298842051,-36.2742356128,-5.26621859632177));
#57987=CARTESIAN_POINT('Ctrl Pts',(9.41083594231989,-36.2742356128,-5.34357802755611));
#57988=CARTESIAN_POINT('Ctrl Pts',(9.34873429723885,-36.2742356128,-5.41993655239066));
#57989=CARTESIAN_POINT('Ctrl Pts',(9.26848598527828,-36.2742356128,-5.51860773435008));
#57990=CARTESIAN_POINT('Ctrl Pts',(9.18622336300651,-36.2742356128,-5.61561399252855));
#57991=CARTESIAN_POINT('Ctrl Pts',(9.10218677827788,-36.2742356128,-5.71107162296444));
#57992=CARTESIAN_POINT('Ctrl Pts',(9.03699830774157,-36.2742356128,-5.78511957421366));
#57993=CARTESIAN_POINT('Ctrl Pts',(8.97073968508115,-36.2742356128,-5.85823828748615));
#57994=CARTESIAN_POINT('Ctrl Pts',(8.90351033446202,-36.2742356128,-5.93047839850826));
#57995=CARTESIAN_POINT('Ctrl Pts',(8.81845068839717,-36.2742356128,-6.02187773850837));
#57996=CARTESIAN_POINT('Ctrl Pts',(8.73184574609042,-36.2742356128,-6.11186368999363));
#57997=CARTESIAN_POINT('Ctrl Pts',(8.64390118549355,-36.2742356128,-6.20048968024117));
#57998=CARTESIAN_POINT('Ctrl Pts',(8.56984778372845,-36.2742356128,-6.2751168773991));
#57999=CARTESIAN_POINT('Ctrl Pts',(8.49484383511191,-36.2742356128,-6.34878012596499));
#58000=CARTESIAN_POINT('Ctrl Pts',(8.41901681523273,-36.2742356128,-6.42146890548941));
#58001=CARTESIAN_POINT('Ctrl Pts',(8.4047929558046,-36.2742356128,-6.43510408439536));
#58002=CARTESIAN_POINT('Ctrl Pts',(8.39054016429969,-36.2742356128,-6.4487048304708));
#58003=CARTESIAN_POINT('Ctrl Pts',(8.37625932979208,-36.2742356128,-6.46227086223795));
#58004=CARTESIAN_POINT('Ctrl Pts',(8.27691241049981,-36.2742356128,-6.55664514144192));
#58005=CARTESIAN_POINT('Ctrl Pts',(8.17619343587986,-36.2742356127799,-6.64936525637284));
#58006=CARTESIAN_POINT('Ctrl Pts',(8.07431943600004,-36.2742356130106,-6.74042458337472));
#58007=CARTESIAN_POINT('Ctrl Pts',(7.9740368388946,-36.2742356132376,-6.83006144668816));
#58008=CARTESIAN_POINT('Ctrl Pts',(7.8726372330311,-36.2742356137614,-6.91808713967223));
#58009=CARTESIAN_POINT('Ctrl Pts',(7.77030787671347,-36.2742356141754,-7.00445497976472));
#58010=CARTESIAN_POINT('Ctrl Pts',(7.69016343904083,-36.2742356144997,-7.07209834454587));
#58011=CARTESIAN_POINT('Ctrl Pts',(7.60944864485436,-36.2742356146977,-7.13872371640073));
#58012=CARTESIAN_POINT('Ctrl Pts',(7.52823172485476,-36.2742356144998,-7.20430188678942));
#58013=CARTESIAN_POINT('Ctrl Pts',(7.44113992314812,-36.2742356142876,-7.27462369918769));
#58014=CARTESIAN_POINT('Ctrl Pts',(7.35346425048188,-36.2742356138161,-7.34374843931962));
#58015=CARTESIAN_POINT('Ctrl Pts',(7.26526468412603,-36.2742356134793,-7.41163792641398));
#58016=CARTESIAN_POINT('Ctrl Pts',(7.20648357004512,-36.2742356132547,-7.45688327002131));
#58017=CARTESIAN_POINT('Ctrl Pts',(7.1474689412501,-36.274235613086,-7.50158006695547));
#58018=CARTESIAN_POINT('Ctrl Pts',(7.08822590343499,-36.2742356129864,-7.545720515055));
#58019=CARTESIAN_POINT('Ctrl Pts',(7.00824771615769,-36.2742356128519,-7.60531018423479));
#58020=CARTESIAN_POINT('Ctrl Pts',(6.92783272624198,-36.2742356128213,-7.66390180221629));
#58021=CARTESIAN_POINT('Ctrl Pts',(6.84694168646384,-36.2742356128083,-7.72149588608444));
#58022=CARTESIAN_POINT('Ctrl Pts',(6.77800623059529,-36.2742356127972,-7.77057764393639));
#58023=CARTESIAN_POINT('Ctrl Pts',(6.70872455283564,-36.2742356128,-7.8189350194394));
#58024=CARTESIAN_POINT('Ctrl Pts',(6.63904441016083,-36.2742356128,-7.86657935124075));
#58025=CARTESIAN_POINT('Ctrl Pts',(6.51500653126901,-36.2742356128,-7.95139120194889));
#58026=CARTESIAN_POINT('Ctrl Pts',(6.38973081761568,-36.2742356128,-8.03391823531077));
#58027=CARTESIAN_POINT('Ctrl Pts',(6.26311690885472,-36.2742356128,-8.11405915608162));
#58028=CARTESIAN_POINT('Ctrl Pts',(6.14082382425489,-36.2742356128,-8.19146518911263));
#58029=CARTESIAN_POINT('Ctrl Pts',(6.01728298717408,-36.2742356128,-8.26664531147886));
#58030=CARTESIAN_POINT('Ctrl Pts',(5.8924473777231,-36.2742356128,-8.33951374852886));
#58031=CARTESIAN_POINT('Ctrl Pts',(5.80107807308279,-36.2742356128,-8.39284739629784));
#58032=CARTESIAN_POINT('Ctrl Pts',(5.7090133522859,-36.2742356128,-8.4449442395566));
#58033=CARTESIAN_POINT('Ctrl Pts',(5.6162580577169,-36.2742356128,-8.4957663466978));
#58034=CARTESIAN_POINT('Ctrl Pts',(5.46867697199189,-36.2742356128,-8.57662838034864));
#58035=CARTESIAN_POINT('Ctrl Pts',(5.319347849749,-36.2742356128,-8.65426137281124));
#58036=CARTESIAN_POINT('Ctrl Pts',(5.16833129815377,-36.2742356128,-8.72852821430025));
#58037=CARTESIAN_POINT('Ctrl Pts',(5.0252243894345,-36.2742356128,-8.79890525571437));
#58038=CARTESIAN_POINT('Ctrl Pts',(4.88060325867337,-36.2742356128,-8.86625971607705));
#58039=CARTESIAN_POINT('Ctrl Pts',(4.73456180799277,-36.2742356128,-8.9304829996254));
#58040=CARTESIAN_POINT('Ctrl Pts',(4.56802863892683,-36.2742356128,-9.00371773460841));
#58041=CARTESIAN_POINT('Ctrl Pts',(4.39963331229614,-36.2742356128,-9.07288577272594));
#58042=CARTESIAN_POINT('Ctrl Pts',(4.22952064919205,-36.2742356128,-9.13789430463033));
#58043=CARTESIAN_POINT('Ctrl Pts',(4.07030290524576,-36.2742356128,-9.19873934460684));
#58044=CARTESIAN_POINT('Ctrl Pts',(3.90958104396924,-36.2742356128,-9.2559399870542));
#58045=CARTESIAN_POINT('Ctrl Pts',(3.74749475790497,-36.2742356128,-9.30946145440929));
#58046=CARTESIAN_POINT('Ctrl Pts',(3.73640355073492,-36.2742356128,-9.3131238104105));
#58047=CARTESIAN_POINT('Ctrl Pts',(3.72530596253903,-36.2742356128,-9.31676895825965));
#58048=CARTESIAN_POINT('Ctrl Pts',(3.71420204145765,-36.2742356128,-9.32039689553507));
#58049=CARTESIAN_POINT('Ctrl Pts',(3.64269698207382,-36.2742356128,-9.34375944183012));
#58050=CARTESIAN_POINT('Ctrl Pts',(3.57093421782095,-36.2742356128,-9.366407200153));
#58051=CARTESIAN_POINT('Ctrl Pts',(3.49894135622052,-36.2742356128,-9.38833730031651));
#58052=CARTESIAN_POINT('Ctrl Pts',(3.36037902120776,-36.2742356128,-9.43054545565535));
#58053=CARTESIAN_POINT('Ctrl Pts',(3.2209545156788,-36.2742356128,-9.47009577861699));
#58054=CARTESIAN_POINT('Ctrl Pts',(3.08060901729276,-36.2742356128,-9.50703410737918));
#58055=CARTESIAN_POINT('Ctrl Pts',(3.01043626809975,-36.2742356128,-9.52550327176028));
#58056=CARTESIAN_POINT('Ctrl Pts',(2.94003215345144,-36.2742356128,-9.54331999022258));
#58057=CARTESIAN_POINT('Ctrl Pts',(2.86942630620849,-36.2742356128,-9.56048475195216));
#58058=CARTESIAN_POINT('Ctrl Pts',(2.80680351316639,-36.2742356128,-9.57570877890434));
#58059=CARTESIAN_POINT('Ctrl Pts',(2.74402151902805,-36.2742356128,-9.59042005980405));
#58060=CARTESIAN_POINT('Ctrl Pts',(2.68114420127632,-36.2742356128,-9.60461135390141));
#58061=CARTESIAN_POINT('Ctrl Pts',(2.67312870066971,-36.2742356128,-9.60642043753464));
#58062=CARTESIAN_POINT('Ctrl Pts',(2.66511172001634,-36.2742356128,-9.60822105857561));
#58063=CARTESIAN_POINT('Ctrl Pts',(2.65709345518398,-36.2742356128,-9.61001319054557));
#58064=CARTESIAN_POINT('Ctrl Pts',(2.61808941652459,-36.2742356128,-9.61873083533534));
#58065=CARTESIAN_POINT('Ctrl Pts',(2.5790435824319,-36.2742356128,-9.62725011661459));
#58066=CARTESIAN_POINT('Ctrl Pts',(2.53993928470411,-36.2742356128,-9.63557594572615));
#58067=CARTESIAN_POINT('Ctrl Pts',(2.49942937662269,-36.2742356128,-9.64420104812176));
#58068=CARTESIAN_POINT('Ctrl Pts',(2.45885925103264,-36.2742356128,-9.65261800011732));
#58069=CARTESIAN_POINT('Ctrl Pts',(2.41824922175855,-36.2742356128,-9.66082393256145));
#58070=CARTESIAN_POINT('Ctrl Pts',(2.37659230003858,-36.2742356128,-9.66924140705173));
#58071=CARTESIAN_POINT('Ctrl Pts',(2.33480257980723,-36.2742356128,-9.67745500886163));
#58072=CARTESIAN_POINT('Ctrl Pts',(2.29293606002991,-36.2742356128,-9.68545254735298));
#58073=CARTESIAN_POINT('Ctrl Pts',(2.25459003428932,-36.2742356128,-9.69277758460188));
#58074=CARTESIAN_POINT('Ctrl Pts',(2.21618141740729,-36.2742356128,-9.69992099315214));
#58075=CARTESIAN_POINT('Ctrl Pts',(2.17771533929591,-36.2742356128,-9.7068828050064));
#58076=CARTESIAN_POINT('Ctrl Pts',(2.14430668976644,-36.2742356128,-9.71292929437441));
#58077=CARTESIAN_POINT('Ctrl Pts',(2.11089595707496,-36.2742356128,-9.71883173440012));
#58078=CARTESIAN_POINT('Ctrl Pts',(2.07730895436942,-36.2742356128,-9.72462310550832));
#58079=CARTESIAN_POINT('Ctrl Pts',(2.07044188243394,-36.2742356128,-9.7258071874091));
#58080=CARTESIAN_POINT('Ctrl Pts',(2.06356727156797,-36.2742356128,-9.72698664924094));
#58081=CARTESIAN_POINT('Ctrl Pts',(2.05668335047021,-36.2742356128,-9.72816181233373));
#58082=CARTESIAN_POINT('Ctrl Pts',(2.03915739474699,-36.2742356128,-9.73115369095048));
#58083=CARTESIAN_POINT('Ctrl Pts',(2.02157756711238,-36.2742356127996,-9.73411696258259));
#58084=CARTESIAN_POINT('Ctrl Pts',(2.00384190141366,-36.2742356128022,-9.7370687432509));
#58085=CARTESIAN_POINT('Ctrl Pts',(1.98521996349978,-36.2742356128049,-9.74016802789431));
#58086=CARTESIAN_POINT('Ctrl Pts',(1.9664264382516,-36.2742356128118,-9.74325461496629));
#58087=CARTESIAN_POINT('Ctrl Pts',(1.94740019190711,-36.2742356128226,-9.74634003414102));
#58088=CARTESIAN_POINT('Ctrl Pts',(1.94261758327247,-36.2742356128253,-9.74711561289257));
#58089=CARTESIAN_POINT('Ctrl Pts',(1.93782052766086,-36.2742356128282,-9.74789108023816));
#58090=CARTESIAN_POINT('Ctrl Pts',(1.93300854997167,-36.2742356128312,-9.74866654690155));
#58091=CARTESIAN_POINT('Ctrl Pts',(1.91128349112384,-36.2742356128447,-9.75216761444278));
#58092=CARTESIAN_POINT('Ctrl Pts',(1.88923535030687,-36.2742356128578,-9.75567154153552));
#58093=CARTESIAN_POINT('Ctrl Pts',(1.86684962573881,-36.2742356128663,-9.75918465724687));
#58094=CARTESIAN_POINT('Ctrl Pts',(1.84177859870743,-36.2742356128757,-9.76311919234293));
#58095=CARTESIAN_POINT('Ctrl Pts',(1.81628495192361,-36.2742356128796,-9.76706514100968));
#58096=CARTESIAN_POINT('Ctrl Pts',(1.79042259448784,-36.2742356128782,-9.77102027035687));
#58097=CARTESIAN_POINT('Ctrl Pts',(1.75485788918616,-36.2742356128763,-9.77645917939724));
#58098=CARTESIAN_POINT('Ctrl Pts',(1.71859866610285,-36.2742356128649,-9.78191510402332));
#58099=CARTESIAN_POINT('Ctrl Pts',(1.68190111891461,-36.2742356128521,-9.78736428204235));
#58100=CARTESIAN_POINT('Ctrl Pts',(1.65417492786119,-36.2742356128425,-9.79148131335413));
#58101=CARTESIAN_POINT('Ctrl Pts',(1.62620285863509,-36.2742356128323,-9.79559383857571));
#58102=CARTESIAN_POINT('Ctrl Pts',(1.59808657345918,-36.2742356128241,-9.79969240046506));
#58103=CARTESIAN_POINT('Ctrl Pts',(1.57334962904916,-36.2742356128169,-9.80329834972128));
#58104=CARTESIAN_POINT('Ctrl Pts',(1.5485022020045,-36.2742356128113,-9.80689331747091));
#58105=CARTESIAN_POINT('Ctrl Pts',(1.5235774246962,-36.2742356128076,-9.81047583278086));
#58106=CARTESIAN_POINT('Ctrl Pts',(1.50128004231585,-36.2742356128042,-9.8136807044939));
#58107=CARTESIAN_POINT('Ctrl Pts',(1.4789210815784,-36.2742356128023,-9.81687556029816));
#58108=CARTESIAN_POINT('Ctrl Pts',(1.45648473849049,-36.2742356128013,-9.82006491224659));
#58109=CARTESIAN_POINT('Ctrl Pts',(1.43437802239104,-36.2742356128003,-9.82320740733988));
#58110=CARTESIAN_POINT('Ctrl Pts',(1.41219693864792,-36.2742356128001,-9.82634444875315));
#58111=CARTESIAN_POINT('Ctrl Pts',(1.38987732415055,-36.2742356128,-9.82948731744555));
#58112=CARTESIAN_POINT('Ctrl Pts',(1.37512031792225,-36.2742356128,-9.8315652804352));
#58113=CARTESIAN_POINT('Ctrl Pts',(1.36029433326,-36.2742356128,-9.83364697235));
#58114=CARTESIAN_POINT('Ctrl Pts',(1.34538289151,-36.2742356128,-9.83573536665));
#58115=CARTESIAN_POINT('',(-1.34538336432,-36.2742356128,-9.83573530247));
#58116=CARTESIAN_POINT('Origin',(-0.000204993183026136,-36.2742356127865,
-2.71388259243404));
#58117=CARTESIAN_POINT('',(-10.7486857267508,-36.2742356128,0.754197292576714));
#58118=CARTESIAN_POINT('Ctrl Pts',(-1.34538336432,-36.2742356128,-9.83573530247));
#58119=CARTESIAN_POINT('Ctrl Pts',(-1.36873192615361,-36.2742356128,-9.83246526657691));
#58120=CARTESIAN_POINT('Ctrl Pts',(-1.39186001383178,-36.2742356128,-9.82921313015801));
#58121=CARTESIAN_POINT('Ctrl Pts',(-1.41485686696532,-36.2742356128,-9.82596411801518));
#58122=CARTESIAN_POINT('Ctrl Pts',(-1.43950188342316,-36.2742356128,-9.82248225215873));
#58123=CARTESIAN_POINT('Ctrl Pts',(-1.46399603833782,-36.2742356128,-9.81900399480443));
#58124=CARTESIAN_POINT('Ctrl Pts',(-1.48838901468098,-36.2742356128,-9.81551943919389));
#58125=CARTESIAN_POINT('Ctrl Pts',(-1.51553080490511,-36.2742356128,-9.81164221338614));
#58126=CARTESIAN_POINT('Ctrl Pts',(-1.54254718023759,-36.2742356128,-9.80775721188026));
#58127=CARTESIAN_POINT('Ctrl Pts',(-1.56943612727103,-36.2742356128,-9.803860463866));
#58128=CARTESIAN_POINT('Ctrl Pts',(-1.59559432632052,-36.2742356128,-9.80006961589876));
#58129=CARTESIAN_POINT('Ctrl Pts',(-1.62163027431294,-36.2742356128,-9.79626788013378));
#58130=CARTESIAN_POINT('Ctrl Pts',(-1.64749532464658,-36.2742356128,-9.79245800174802));
#58131=CARTESIAN_POINT('Ctrl Pts',(-1.68855743602486,-36.2742356128,-9.78640962184556));
#58132=CARTESIAN_POINT('Ctrl Pts',(-1.72915458194226,-36.2742356128,-9.78034584082381));
#58133=CARTESIAN_POINT('Ctrl Pts',(-1.76902422177875,-36.2742356128,-9.77428634403978));
#58134=CARTESIAN_POINT('Ctrl Pts',(-1.79804062664776,-36.2742356128,-9.76987635155655));
#58135=CARTESIAN_POINT('Ctrl Pts',(-1.82666762765698,-36.2742356128,-9.76546917205919));
#58136=CARTESIAN_POINT('Ctrl Pts',(-1.85481242636501,-36.2742356128,-9.76107078246235));
#58137=CARTESIAN_POINT('Ctrl Pts',(-1.88089833376722,-36.2742356128,-9.75699415057977));
#58138=CARTESIAN_POINT('Ctrl Pts',(-1.90656839898667,-36.2742356128,-9.75292529183231));
#58139=CARTESIAN_POINT('Ctrl Pts',(-1.93178873575894,-36.2742356128,-9.74886307273241));
#58140=CARTESIAN_POINT('Ctrl Pts',(-1.95424178948369,-36.2742356128,-9.74524657765879));
#58141=CARTESIAN_POINT('Ctrl Pts',(-1.97632472956562,-36.2742356128,-9.74163749451863));
#58142=CARTESIAN_POINT('Ctrl Pts',(-1.99819673805766,-36.2742356128,-9.73800714264926));
#58143=CARTESIAN_POINT('Ctrl Pts',(-2.02006874654969,-36.2742356128,-9.7343767907799));
#58144=CARTESIAN_POINT('Ctrl Pts',(-2.04172901427369,-36.2742356128,-9.73072531915584));
#58145=CARTESIAN_POINT('Ctrl Pts',(-2.06328081535604,-36.2742356128,-9.72703421190412));
#58146=CARTESIAN_POINT('Ctrl Pts',(-2.08754806620901,-36.2742356128,-9.72287803835462));
#58147=CARTESIAN_POINT('Ctrl Pts',(-2.11170713674881,-36.2742356128,-9.71866665247062));
#58148=CARTESIAN_POINT('Ctrl Pts',(-2.13583519969934,-36.2742356128,-9.71438572233037));
#58149=CARTESIAN_POINT('Ctrl Pts',(-2.1545635127234,-36.2742356128,-9.71106284473903));
#58150=CARTESIAN_POINT('Ctrl Pts',(-2.17327157628719,-36.2742356128,-9.70769835376932));
#58151=CARTESIAN_POINT('Ctrl Pts',(-2.19197454480384,-36.2742356128,-9.70428935658671));
#58152=CARTESIAN_POINT('Ctrl Pts',(-2.22291726659735,-36.2742356128,-9.69864941492063));
#58153=CARTESIAN_POINT('Ctrl Pts',(-2.25381741316753,-36.2742356128,-9.69289305897368));
#58154=CARTESIAN_POINT('Ctrl Pts',(-2.2846783512042,-36.2742356128,-9.6870198736353));
#58155=CARTESIAN_POINT('Ctrl Pts',(-2.3163344605537,-36.2742356128,-9.68099535820805));
#58156=CARTESIAN_POINT('Ctrl Pts',(-2.34794406706507,-36.2742356128,-9.67484888353989));
#58157=CARTESIAN_POINT('Ctrl Pts',(-2.37949158813658,-36.2742356128,-9.66858317796076));
#58158=CARTESIAN_POINT('Ctrl Pts',(-2.40226571075079,-36.2742356128,-9.66405997162704));
#58159=CARTESIAN_POINT('Ctrl Pts',(-2.42500680916096,-36.2742356128,-9.65947474510775));
#58160=CARTESIAN_POINT('Ctrl Pts',(-2.44772709714164,-36.2742356128,-9.65482507592072));
#58161=CARTESIAN_POINT('Ctrl Pts',(-2.56023068653774,-36.2742356128,-9.63180140326789));
#58162=CARTESIAN_POINT('Ctrl Pts',(-2.67239663947122,-36.2742356128,-9.60716179468203));
#58163=CARTESIAN_POINT('Ctrl Pts',(-2.78410583615521,-36.2742356128,-9.58089117609618));
#58164=CARTESIAN_POINT('Ctrl Pts',(-2.91213087583812,-36.2742356128,-9.5507835655611));
#58165=CARTESIAN_POINT('Ctrl Pts',(-3.03955637547996,-36.2742356128,-9.51853361892697));
#58166=CARTESIAN_POINT('Ctrl Pts',(-3.16627236350259,-36.2742356128,-9.48412781383033));
#58167=CARTESIAN_POINT('Ctrl Pts',(-3.33084393041467,-36.2742356128,-9.43944349779427));
#58168=CARTESIAN_POINT('Ctrl Pts',(-3.49422083013493,-36.2742356128,-9.39112237778561));
#58169=CARTESIAN_POINT('Ctrl Pts',(-3.65625877301338,-36.2742356128,-9.3391546000114));
#58170=CARTESIAN_POINT('Ctrl Pts',(-3.72138584122313,-36.2742356128,-9.31826746118647));
#58171=CARTESIAN_POINT('Ctrl Pts',(-3.78629724319742,-36.2742356128,-9.29679144790176));
#58172=CARTESIAN_POINT('Ctrl Pts',(-3.85098428965109,-36.2742356128,-9.27472670369536));
#58173=CARTESIAN_POINT('Ctrl Pts',(-3.9588347526871,-36.2742356128,-9.23793892298973));
#58174=CARTESIAN_POINT('Ctrl Pts',(-4.06606530659819,-36.2742356128,-9.19951199868619));
#58175=CARTESIAN_POINT('Ctrl Pts',(-4.17264953538524,-36.2742356128,-9.15944992060988));
#58176=CARTESIAN_POINT('Ctrl Pts',(-4.31330125818643,-36.2742356128,-9.10658280917554));
#58177=CARTESIAN_POINT('Ctrl Pts',(-4.45282276293723,-36.2742356128,-9.05086944491036));
#58178=CARTESIAN_POINT('Ctrl Pts',(-4.59109734883041,-36.2742356128,-8.99237091677724));
#58179=CARTESIAN_POINT('Ctrl Pts',(-4.68122888517629,-36.2742356128,-8.95423981567466));
#58180=CARTESIAN_POINT('Ctrl Pts',(-4.77082945282832,-36.2742356128,-8.91492649134275));
#58181=CARTESIAN_POINT('Ctrl Pts',(-4.85988107462091,-36.2742356128,-8.87444749687177));
#58182=CARTESIAN_POINT('Ctrl Pts',(-5.02447950840956,-36.2742356128,-8.79962820714811));
#58183=CARTESIAN_POINT('Ctrl Pts',(-5.1872188048343,-36.2742356128,-8.72081653937812));
#58184=CARTESIAN_POINT('Ctrl Pts',(-5.34797972852781,-36.2742356128,-8.63818055603731));
#58185=CARTESIAN_POINT('Ctrl Pts',(-5.48874063022716,-36.2742356128,-8.56582518969192));
#58186=CARTESIAN_POINT('Ctrl Pts',(-5.62798392544602,-36.2742356128,-8.49053890087286));
#58187=CARTESIAN_POINT('Ctrl Pts',(-5.76567045786445,-36.2742356128,-8.41244582504101));
#58188=CARTESIAN_POINT('Ctrl Pts',(-5.78523365789672,-36.2742356128,-8.40134996521508));
#58189=CARTESIAN_POINT('Ctrl Pts',(-5.80476551601904,-36.2742356128,-8.39019744922167));
#58190=CARTESIAN_POINT('Ctrl Pts',(-5.82426601120212,-36.2742356128,-8.37898863848497));
#58191=CARTESIAN_POINT('Ctrl Pts',(-5.94879618143595,-36.2742356128,-8.30740916852515));
#58192=CARTESIAN_POINT('Ctrl Pts',(-6.0720464167817,-36.2742356128013,-8.23353358940084));
#58193=CARTESIAN_POINT('Ctrl Pts',(-6.19404162526371,-36.2742356128036,
-8.15745074881589));
#58194=CARTESIAN_POINT('Ctrl Pts',(-6.22651395401904,-36.2742356128042,
-8.13719924022915));
#58195=CARTESIAN_POINT('Ctrl Pts',(-6.25889764340576,-36.2742356128047,
-8.11679132494019));
#58196=CARTESIAN_POINT('Ctrl Pts',(-6.29119380735,-36.2742356128048,-8.0962286165475));
#58197=CARTESIAN_POINT('Ctrl Pts',(-6.40358306597281,-36.2742356128052,
-8.02467127755451));
#58198=CARTESIAN_POINT('Ctrl Pts',(-6.51492060843053,-36.2742356128007,
-7.95123207123157));
#58199=CARTESIAN_POINT('Ctrl Pts',(-6.62528347199178,-36.2742356128002,
-7.87597629186123));
#58200=CARTESIAN_POINT('Ctrl Pts',(-6.66578018426995,-36.2742356128,-7.84836182494647));
#58201=CARTESIAN_POINT('Ctrl Pts',(-6.70614614403169,-36.2742356128,-7.82050268772187));
#58202=CARTESIAN_POINT('Ctrl Pts',(-6.74638693431083,-36.2742356128,-7.7924018035638));
#58203=CARTESIAN_POINT('Ctrl Pts',(-6.83209224893783,-36.2742356128,-7.73255220564692));
#58204=CARTESIAN_POINT('Ctrl Pts',(-6.91722166165999,-36.2742356127998,
-7.67161278498377));
#58205=CARTESIAN_POINT('Ctrl Pts',(-7.00186018562873,-36.2742356128002,
-7.60955849043406));
#58206=CARTESIAN_POINT('Ctrl Pts',(-7.06526117816682,-36.2742356128005,
-7.56307488366468));
#58207=CARTESIAN_POINT('Ctrl Pts',(-7.12838556141735,-36.2742356128008,
-7.51596612269866));
#58208=CARTESIAN_POINT('Ctrl Pts',(-7.19125084904421,-36.2742356128052,
-7.46822717531959));
#58209=CARTESIAN_POINT('Ctrl Pts',(-7.28093214970969,-36.2742356128117,
-7.40012455374617));
#58210=CARTESIAN_POINT('Ctrl Pts',(-7.37008459041437,-36.2742356128522,
-7.33074518643801));
#58211=CARTESIAN_POINT('Ctrl Pts',(-7.45866128730512,-36.2742356130763,
-7.26012267330857));
#58212=CARTESIAN_POINT('Ctrl Pts',(-7.51506525656589,-36.2742356132191,
-7.21515158949649));
#58213=CARTESIAN_POINT('Ctrl Pts',(-7.57123465324818,-36.2742356134335,
-7.16967680621853));
#58214=CARTESIAN_POINT('Ctrl Pts',(-7.62714692446239,-36.2742356136452,
-7.1237099999356));
#58215=CARTESIAN_POINT('Ctrl Pts',(-7.72186099987924,-36.2742356140038,
-7.04584330873512));
#58216=CARTESIAN_POINT('Ctrl Pts',(-7.81583817186816,-36.2742356139541,
-6.9665618692806));
#58217=CARTESIAN_POINT('Ctrl Pts',(-7.90897295499202,-36.2742356137047,
-6.88589608108511));
#58218=CARTESIAN_POINT('Ctrl Pts',(-8.00830703058412,-36.2742356134387,
-6.79986096902981));
#58219=CARTESIAN_POINT('Ctrl Pts',(-8.1066825535539,-36.2742356130684,-6.71225191373121));
#58220=CARTESIAN_POINT('Ctrl Pts',(-8.20390980861941,-36.2742356129219,
-6.6231017683274));
#58221=CARTESIAN_POINT('Ctrl Pts',(-8.29323343819682,-36.2742356127874,
-6.54119865834599));
#58222=CARTESIAN_POINT('Ctrl Pts',(-8.3815866134665,-36.2742356128,-6.45799529379827));
#58223=CARTESIAN_POINT('Ctrl Pts',(-8.46878561291554,-36.2742356128,-6.37350477083193));
#58224=CARTESIAN_POINT('Ctrl Pts',(-8.54861727170136,-36.2742356128,-6.29615275254384));
#58225=CARTESIAN_POINT('Ctrl Pts',(-8.62746167428925,-36.2742356128,-6.21773879006739));
#58226=CARTESIAN_POINT('Ctrl Pts',(-8.70522553838402,-36.2742356128,-6.13822690867235));
#58227=CARTESIAN_POINT('Ctrl Pts',(-8.78679099037235,-36.2742356128,-6.05482798527877));
#58228=CARTESIAN_POINT('Ctrl Pts',(-8.86716721026386,-36.2742356128,-5.97022079146199));
#58229=CARTESIAN_POINT('Ctrl Pts',(-8.94618759528663,-36.2742356128,-5.88435809015603));
#58230=CARTESIAN_POINT('Ctrl Pts',(-9.03255992341744,-36.2742356128,-5.79050684646417));
#58231=CARTESIAN_POINT('Ctrl Pts',(-9.11731190902216,-36.2742356128,-5.69515496172929));
#58232=CARTESIAN_POINT('Ctrl Pts',(-9.20016409670066,-36.2742356128,-5.59824222254515));
#58233=CARTESIAN_POINT('Ctrl Pts',(-9.21466058872522,-36.2742356128,-5.58128558217118));
#58234=CARTESIAN_POINT('Ctrl Pts',(-9.2290987929291,-36.2742356128,-5.56428117657646));
#58235=CARTESIAN_POINT('Ctrl Pts',(-9.24347706216678,-36.2742356128,-5.54722871240165));
#58236=CARTESIAN_POINT('Ctrl Pts',(-9.33736505491488,-36.2742356128,-5.4358786182898));
#58237=CARTESIAN_POINT('Ctrl Pts',(-9.42881343962009,-36.2742356128,-5.3223429594838));
#58238=CARTESIAN_POINT('Ctrl Pts',(-9.51727873836186,-36.2742356128,-5.20658874584902));
#58239=CARTESIAN_POINT('Ctrl Pts',(-9.60085311192403,-36.2742356128001,
-5.09723416242138));
#58240=CARTESIAN_POINT('Ctrl Pts',(-9.68176232664951,-36.2742356128,-4.98589877259242));
#58241=CARTESIAN_POINT('Ctrl Pts',(-9.75953527294624,-36.2742356128024,
-4.8725958051016));
#58242=CARTESIAN_POINT('Ctrl Pts',(-9.8278398193407,-36.2742356128045,-4.77308680913173));
#58243=CARTESIAN_POINT('Ctrl Pts',(-9.89372402734391,-36.2742356128084,
-4.67206030412638));
#58244=CARTESIAN_POINT('Ctrl Pts',(-9.95688389736168,-36.2742356128213,
-4.56956060979233));
#58245=CARTESIAN_POINT('Ctrl Pts',(-10.0093323537572,-36.2742356128319,
-4.48444405164669));
#58246=CARTESIAN_POINT('Ctrl Pts',(-10.0599020890899,-36.2742356128488,
-4.39831207412655));
#58247=CARTESIAN_POINT('Ctrl Pts',(-10.1084364459268,-36.2742356128813,
-4.3112115267652));
#58248=CARTESIAN_POINT('Ctrl Pts',(-10.16098590539,-36.2742356129165,-4.21690541082817));
#58249=CARTESIAN_POINT('Ctrl Pts',(-10.2111728748833,-36.2742356129955,
-4.12142324744));
#58250=CARTESIAN_POINT('Ctrl Pts',(-10.258847617925,-36.2742356129274,-4.0247804028775));
#58251=CARTESIAN_POINT('Ctrl Pts',(-10.3065223609667,-36.2742356128594,
-3.928137558315));
#58252=CARTESIAN_POINT('Ctrl Pts',(-10.3516784769153,-36.2742356128,-3.83034388890688));
#58253=CARTESIAN_POINT('Ctrl Pts',(-10.3941808250964,-36.2742356128,-3.73153260041563));
#58254=CARTESIAN_POINT('Ctrl Pts',(-10.4361612215928,-36.2742356128,-3.63393476766765));
#58255=CARTESIAN_POINT('Ctrl Pts',(-10.4755527962184,-36.2742356128,-3.53533183188484));
#58256=CARTESIAN_POINT('Ctrl Pts',(-10.5122849628678,-36.2742356128,-3.4358640110323));
#58257=CARTESIAN_POINT('Ctrl Pts',(-10.5499713898602,-36.2742356128,-3.33381212815696));
#58258=CARTESIAN_POINT('Ctrl Pts',(-10.5848585502045,-36.2742356128,-3.23084950337341));
#58259=CARTESIAN_POINT('Ctrl Pts',(-10.6169249038884,-36.2742356128,-3.12711324194226));
#58260=CARTESIAN_POINT('Ctrl Pts',(-10.6498801971988,-36.2742356128,-3.02050121626292));
#58261=CARTESIAN_POINT('Ctrl Pts',(-10.6798562655977,-36.2742356128,-2.91307165429687));
#58262=CARTESIAN_POINT('Ctrl Pts',(-10.7068847881371,-36.2742356128,-2.80496421163292));
#58263=CARTESIAN_POINT('Ctrl Pts',(-10.7351414874224,-36.2742356128,-2.69194436404779));
#58264=CARTESIAN_POINT('Ctrl Pts',(-10.7601767403046,-36.2742356128,-2.57818309705358));
#58265=CARTESIAN_POINT('Ctrl Pts',(-10.7820847464602,-36.2742356128,-2.46383743509071));
#58266=CARTESIAN_POINT('Ctrl Pts',(-10.804480029669,-36.2742356128,-2.34694850119332));
#58267=CARTESIAN_POINT('Ctrl Pts',(-10.8236077570002,-36.2742356128,-2.22944822633344));
#58268=CARTESIAN_POINT('Ctrl Pts',(-10.83962436159,-36.2742356128,-2.11151102066995));
#58269=CARTESIAN_POINT('Ctrl Pts',(-10.8560200341834,-36.2742356128,-1.99078257290199));
#58270=CARTESIAN_POINT('Ctrl Pts',(-10.8691559979564,-36.2742356128,-1.86959548423268));
#58271=CARTESIAN_POINT('Ctrl Pts',(-10.8792519960503,-36.2742356128,-1.74815488119674));
#58272=CARTESIAN_POINT('Ctrl Pts',(-10.8879558783918,-36.2742356128,-1.64345946520516));
#58273=CARTESIAN_POINT('Ctrl Pts',(-10.8944014197242,-36.2742356128,-1.53857564242055));
#58274=CARTESIAN_POINT('Ctrl Pts',(-10.8987553032475,-36.2742356128,-1.43365203176424));
#58275=CARTESIAN_POINT('Ctrl Pts',(-10.9028812002675,-36.2742356128,-1.33422263494579));
#58276=CARTESIAN_POINT('Ctrl Pts',(-10.9051326101663,-36.2742356128147,
-1.23473829160415));
#58277=CARTESIAN_POINT('Ctrl Pts',(-10.9056752402414,-36.2742356128297,
-1.13528552213591));
#58278=CARTESIAN_POINT('Ctrl Pts',(-10.905948870433,-36.2742356128373,-1.08513481796376));
#58279=CARTESIAN_POINT('Ctrl Pts',(-10.9057882730935,-36.2742356128356,
-1.03499309683131));
#58280=CARTESIAN_POINT('Ctrl Pts',(-10.9052159192415,-36.2742356128214,
-0.984876028825734));
#58281=CARTESIAN_POINT('Ctrl Pts',(-10.9036483921713,-36.2742356127825,
-0.847618525439958));
#58282=CARTESIAN_POINT('Ctrl Pts',(-10.8990065748664,-36.2742356128,-0.710462270989658));
#58283=CARTESIAN_POINT('Ctrl Pts',(-10.8917400860261,-36.2742356128,-0.573593958805236));
#58284=CARTESIAN_POINT('Ctrl Pts',(-10.89109179549,-36.2742356128,-0.561383050147837));
#58285=CARTESIAN_POINT('Ctrl Pts',(-10.8904225852203,-36.2742356128,-0.549174450233));
#58286=CARTESIAN_POINT('Ctrl Pts',(-10.8897327552813,-36.2742356128,-0.536968294734768));
#58287=CARTESIAN_POINT('Ctrl Pts',(-10.8837830369874,-36.2742356128,-0.431691352474246));
#58288=CARTESIAN_POINT('Ctrl Pts',(-10.8763040991208,-36.2742356127999,
-0.326639000646442));
#58289=CARTESIAN_POINT('Ctrl Pts',(-10.8674818264598,-36.2742356128008,
-0.22192376216726));
#58290=CARTESIAN_POINT('Ctrl Pts',(-10.8594054799106,-36.2742356128016,
-0.126062232215319));
#58291=CARTESIAN_POINT('Ctrl Pts',(-10.8502036955816,-36.2742356128034,
-0.0304844637507402));
#58292=CARTESIAN_POINT('Ctrl Pts',(-10.8399937081216,-36.2742356128072,
0.0647615827492694));
#58293=CARTESIAN_POINT('Ctrl Pts',(-10.8309039223079,-36.2742356128105,
0.149557589177328));
#58294=CARTESIAN_POINT('Ctrl Pts',(-10.821014992842,-36.2742356128154,0.234090431265654));
#58295=CARTESIAN_POINT('Ctrl Pts',(-10.8103871197297,-36.2742356128217,
0.318366652044579));
#58296=CARTESIAN_POINT('Ctrl Pts',(-10.8090773681909,-36.2742356128224,
0.328752635080224));
#58297=CARTESIAN_POINT('Ctrl Pts',(-10.8077563633402,-36.2742356128232,
0.339134778623737));
#58298=CARTESIAN_POINT('Ctrl Pts',(-10.8064241912105,-36.274235612824,0.349513145801407));
#58299=CARTESIAN_POINT('Ctrl Pts',(-10.7964147294364,-36.2742356128301,
0.427492460355431));
#58300=CARTESIAN_POINT('Ctrl Pts',(-10.7857704427514,-36.2742356128116,
0.505286572762631));
#58301=CARTESIAN_POINT('Ctrl Pts',(-10.7745234778453,-36.2742356128047,
0.582901949111922));
#58302=CARTESIAN_POINT('Ctrl Pts',(-10.7664801617643,-36.2742356127998,
0.638408924543487));
#58303=CARTESIAN_POINT('Ctrl Pts',(-10.7581282570519,-36.2742356128,0.693825319961049));
#58304=CARTESIAN_POINT('Ctrl Pts',(-10.7494730251887,-36.2742356128,0.749168689975769));
#58305=CARTESIAN_POINT('Ctrl Pts',(-10.7492108798837,-36.2742356128,0.750844902102528));
#58306=CARTESIAN_POINT('Ctrl Pts',(-10.7489485455957,-36.2742356128,0.752520471234549));
#58307=CARTESIAN_POINT('Ctrl Pts',(-10.7486857254,-36.2742356128,0.754197292365));
#58308=CARTESIAN_POINT('',(-10.0697229965085,-36.2742356128,2.85693688465354));
#58309=CARTESIAN_POINT('Ctrl Pts',(-10.7486857274262,-36.2742356128,0.754197292682571));
#58310=CARTESIAN_POINT('Ctrl Pts',(-10.7466347100106,-36.2742356128,0.76728316308377));
#58311=CARTESIAN_POINT('Ctrl Pts',(-10.7445707440896,-36.2742356128,0.780341200776172));
#58312=CARTESIAN_POINT('Ctrl Pts',(-10.7424805359006,-36.2742356128,0.793459979414592));
#58313=CARTESIAN_POINT('Ctrl Pts',(-10.7403033711681,-36.2742356128,0.807124523613989));
#58314=CARTESIAN_POINT('Ctrl Pts',(-10.7380978053388,-36.2742356128,0.820854571233398));
#58315=CARTESIAN_POINT('Ctrl Pts',(-10.735858085814,-36.2742356128,0.83469174146334));
#58316=CARTESIAN_POINT('Ctrl Pts',(-10.7334143699778,-36.2742356128,0.84978921757311));
#58317=CARTESIAN_POINT('Ctrl Pts',(-10.7309300554775,-36.2742356128,0.86501392019776));
#58318=CARTESIAN_POINT('Ctrl Pts',(-10.7284075639199,-36.2742356128,0.880356505459193));
#58319=CARTESIAN_POINT('Ctrl Pts',(-10.7271711788056,-36.2742356128,0.88787658772669));
#58320=CARTESIAN_POINT('Ctrl Pts',(-10.7259257592404,-36.2742356128,0.895424102088776));
#58321=CARTESIAN_POINT('Ctrl Pts',(-10.7246722509293,-36.2742356128,0.902993610477458));
#58322=CARTESIAN_POINT('Ctrl Pts',(-10.7214793362214,-36.2742356128,0.92227453143526));
#58323=CARTESIAN_POINT('Ctrl Pts',(-10.7182369499646,-36.2742356128,0.941680848865234));
#58324=CARTESIAN_POINT('Ctrl Pts',(-10.7149640328869,-36.2742356128,0.961095935537187));
#58325=CARTESIAN_POINT('Ctrl Pts',(-10.710943115382,-36.2742356128,0.984948193325674));
#58326=CARTESIAN_POINT('Ctrl Pts',(-10.7068773780433,-36.2742356128,1.00880694510491));
#58327=CARTESIAN_POINT('Ctrl Pts',(-10.7028050282133,-36.2742356128,1.0324118968847));
#58328=CARTESIAN_POINT('Ctrl Pts',(-10.7014661577841,-36.2742356128,1.04017251992562));
#58329=CARTESIAN_POINT('Ctrl Pts',(-10.700126495208,-36.2742356128,1.04790594476556));
#58330=CARTESIAN_POINT('Ctrl Pts',(-10.6987869997851,-36.2742356128,1.05560462756857));
#58331=CARTESIAN_POINT('Ctrl Pts',(-10.6948568818239,-36.2742356128,1.07819278355985));
#58332=CARTESIAN_POINT('Ctrl Pts',(-10.6909302150522,-36.2742356128003,
1.10047278567806));
#58333=CARTESIAN_POINT('Ctrl Pts',(-10.6869822640891,-36.2742356128002,
1.12254281928174));
#58334=CARTESIAN_POINT('Ctrl Pts',(-10.6865220270064,-36.2742356128002,
1.12511565971891));
#58335=CARTESIAN_POINT('Ctrl Pts',(-10.6860615104574,-36.2742356128001,
1.12768558829675));
#58336=CARTESIAN_POINT('Ctrl Pts',(-10.6856006835494,-36.2742356128001,
1.13025271194762));
#58337=CARTESIAN_POINT('Ctrl Pts',(-10.6817956442668,-36.2742356127999,
1.15144940460008));
#58338=CARTESIAN_POINT('Ctrl Pts',(-10.6779522323996,-36.2742356128,1.17255666838632));
#58339=CARTESIAN_POINT('Ctrl Pts',(-10.6740322378691,-36.2742356128,1.19373676928056));
#58340=CARTESIAN_POINT('Ctrl Pts',(-10.673405047118,-36.2742356128,1.1971255401797));
#58341=CARTESIAN_POINT('Ctrl Pts',(-10.6727759081903,-36.2742356128,1.20051606814297));
#58342=CARTESIAN_POINT('Ctrl Pts',(-10.6721446787479,-36.2742356128,1.20390889359303));
#58343=CARTESIAN_POINT('Ctrl Pts',(-10.66836441158,-36.2742356128,1.22422763317181));
#58344=CARTESIAN_POINT('Ctrl Pts',(-10.6645208672205,-36.2742356128,1.24456658224732));
#58345=CARTESIAN_POINT('Ctrl Pts',(-10.6605990453886,-36.2742356128,1.26495926229726));
#58346=CARTESIAN_POINT('Ctrl Pts',(-10.6567628806364,-36.2742356128,1.28490654286344));
#58347=CARTESIAN_POINT('Ctrl Pts',(-10.6528517834809,-36.2742356128,1.30490532216204));
#58348=CARTESIAN_POINT('Ctrl Pts',(-10.6488595061404,-36.2742356128,1.32493766270311));
#58349=CARTESIAN_POINT('Ctrl Pts',(-10.647051148248,-36.2742356128,1.3340115916994));
#58350=CARTESIAN_POINT('Ctrl Pts',(-10.6452262447456,-36.2742356128,1.34309171940456));
#58351=CARTESIAN_POINT('Ctrl Pts',(-10.6433847866665,-36.2742356128,1.35217287965678));
#58352=CARTESIAN_POINT('Ctrl Pts',(-10.6323806657411,-36.2742356128,1.4064397601746));
#58353=CARTESIAN_POINT('Ctrl Pts',(-10.6207566097892,-36.2742356127913,
1.46090931661876));
#58354=CARTESIAN_POINT('Ctrl Pts',(-10.6083335044896,-36.2742356130669,
1.51550391096666));
#58355=CARTESIAN_POINT('Ctrl Pts',(-10.5980828513871,-36.2742356132943,
1.56055144412652));
#58356=CARTESIAN_POINT('Ctrl Pts',(-10.5872879549167,-36.274235613725,1.60568467857377));
#58357=CARTESIAN_POINT('Ctrl Pts',(-10.5758640413931,-36.2742356139669,
1.65083743440026));
#58358=CARTESIAN_POINT('Ctrl Pts',(-10.5642537549898,-36.2742356142128,
1.69672682475306));
#58359=CARTESIAN_POINT('Ctrl Pts',(-10.5519752282585,-36.274235613683,1.74268958094638));
#58360=CARTESIAN_POINT('Ctrl Pts',(-10.5389566649902,-36.2742356133024,
1.78865941825916));
#58361=CARTESIAN_POINT('Ctrl Pts',(-10.526916197855,-36.2742356129504,1.8311755011765));
#58362=CARTESIAN_POINT('Ctrl Pts',(-10.5142426023854,-36.2742356128146,
1.87369793007753));
#58363=CARTESIAN_POINT('Ctrl Pts',(-10.5008991730841,-36.2742356128026,
1.91613325004487));
#58364=CARTESIAN_POINT('Ctrl Pts',(-10.4971520525212,-36.2742356127993,
1.9280499962163));
#58365=CARTESIAN_POINT('Ctrl Pts',(-10.4933522433736,-36.2742356128,1.9399595947355));
#58366=CARTESIAN_POINT('Ctrl Pts',(-10.4894992656358,-36.2742356128,1.95185928753506));
#58367=CARTESIAN_POINT('Ctrl Pts',(-10.4764630530136,-36.2742356128,1.99212085560819));
#58368=CARTESIAN_POINT('Ctrl Pts',(-10.4628146547796,-36.2742356128,2.03226539351294));
#58369=CARTESIAN_POINT('Ctrl Pts',(-10.4485531184273,-36.2742356128,2.0722161323579));
#58370=CARTESIAN_POINT('Ctrl Pts',(-10.4311510100196,-36.2742356128,2.12096453303303));
#58371=CARTESIAN_POINT('Ctrl Pts',(-10.4128342967672,-36.2742356128,2.16942495256767));
#58372=CARTESIAN_POINT('Ctrl Pts',(-10.3935735418708,-36.2742356128,2.21753443994428));
#58373=CARTESIAN_POINT('Ctrl Pts',(-10.3892397005709,-36.2742356128,2.22835950284712));
#58374=CARTESIAN_POINT('Ctrl Pts',(-10.3848580462214,-36.2742356128,2.23916701592833));
#58375=CARTESIAN_POINT('Ctrl Pts',(-10.3804282816357,-36.2742356128,2.24995656315333));
#58376=CARTESIAN_POINT('Ctrl Pts',(-10.3602858532663,-36.2742356128,2.29901733780848));
#58377=CARTESIAN_POINT('Ctrl Pts',(-10.3391381285185,-36.2742356127991,
2.34772286924062));
#58378=CARTESIAN_POINT('Ctrl Pts',(-10.3169784470883,-36.2742356128009,
2.39604450406616));
#58379=CARTESIAN_POINT('Ctrl Pts',(-10.2996209021515,-36.2742356128023,
2.43389454945364));
#58380=CARTESIAN_POINT('Ctrl Pts',(-10.2816424669362,-36.2742356128035,
2.47151008695783));
#58381=CARTESIAN_POINT('Ctrl Pts',(-10.2630751322098,-36.2742356128281,
2.50885913887986));
#58382=CARTESIAN_POINT('Ctrl Pts',(-10.2579382954049,-36.274235612835,2.51919212352028));
#58383=CARTESIAN_POINT('Ctrl Pts',(-10.2527566283131,-36.2742356128438,
2.52950454518725));
#58384=CARTESIAN_POINT('Ctrl Pts',(-10.2475314196008,-36.2742356128559,
2.53979528804326));
#58385=CARTESIAN_POINT('Ctrl Pts',(-10.2308331190384,-36.2742356128946,
2.57268161406069));
#58386=CARTESIAN_POINT('Ctrl Pts',(-10.2136865708931,-36.2742356129131,
2.60534561599341));
#58387=CARTESIAN_POINT('Ctrl Pts',(-10.1961534776876,-36.2742356129027,
2.63773913604163));
#58388=CARTESIAN_POINT('Ctrl Pts',(-10.1794029073218,-36.2742356128926,
2.66868689469456));
#58389=CARTESIAN_POINT('Ctrl Pts',(-10.1622992734439,-36.2742356128632,
2.69938813456047));
#58390=CARTESIAN_POINT('Ctrl Pts',(-10.1449311774068,-36.2742356128411,
2.72977010446408));
#58391=CARTESIAN_POINT('Ctrl Pts',(-10.1284729936058,-36.2742356128201,
2.75856036701445));
#58392=CARTESIAN_POINT('Ctrl Pts',(-10.1117772303903,-36.2742356128067,
2.78706411662779));
#58393=CARTESIAN_POINT('Ctrl Pts',(-10.0949536082382,-36.2742356128024,
2.81518754030304));
#58394=CARTESIAN_POINT('Ctrl Pts',(-10.0874038333031,-36.2742356128005,
2.82780821837302));
#58395=CARTESIAN_POINT('Ctrl Pts',(-10.0798287935207,-36.2742356128,2.84035184669534));
#58396=CARTESIAN_POINT('Ctrl Pts',(-10.0722409181048,-36.2742356128,2.852807544641));
#58397=CARTESIAN_POINT('Ctrl Pts',(-10.0714016752641,-36.2742356128,2.85418518393445));
#58398=CARTESIAN_POINT('Ctrl Pts',(-10.0705624326333,-36.2742356128,2.8555615233));
#58399=CARTESIAN_POINT('Ctrl Pts',(-10.0697233643,-36.2742356128,2.85693628205));
#58400=CARTESIAN_POINT('',(-6.79137755865781,-36.2742356128,3.87179939717186));
#58401=CARTESIAN_POINT('Ctrl Pts',(-10.0697226283806,-36.2742356128,2.85693748780849));
#58402=CARTESIAN_POINT('Ctrl Pts',(-10.0427054783743,-36.2742356128,2.90120340679101));
#58403=CARTESIAN_POINT('Ctrl Pts',(-10.0149092741399,-36.2742356127643,
2.94543590664087));
#58404=CARTESIAN_POINT('Ctrl Pts',(-9.98630861921963,-36.2742356129976,
2.98947462773241));
#58405=CARTESIAN_POINT('Ctrl Pts',(-9.95238280831748,-36.2742356132744,
3.04171291836917));
#58406=CARTESIAN_POINT('Ctrl Pts',(-9.91732467064534,-36.2742356140585,
3.09367893362379));
#58407=CARTESIAN_POINT('Ctrl Pts',(-9.8810149855395,-36.2742356151925,3.14509238921441));
#58408=CARTESIAN_POINT('Ctrl Pts',(-9.83360425537131,-36.2742356166732,
3.21222460098977));
#58409=CARTESIAN_POINT('Ctrl Pts',(-9.78405490480505,-36.2742356185765,
3.27841636101275));
#58410=CARTESIAN_POINT('Ctrl Pts',(-9.73201375282073,-36.2742356181146,
3.34300597725677));
#58411=CARTESIAN_POINT('Ctrl Pts',(-9.70350081936561,-36.2742356178616,
3.37839411452191));
#58412=CARTESIAN_POINT('Ctrl Pts',(-9.67423897805512,-36.2742356168433,
3.41330054426729));
#58413=CARTESIAN_POINT('Ctrl Pts',(-9.64417559703147,-36.274235615507,3.44761070496689));
#58414=CARTESIAN_POINT('Ctrl Pts',(-9.62933185379337,-36.2742356148472,
3.46455128844558));
#58415=CARTESIAN_POINT('Ctrl Pts',(-9.61430073230973,-36.2742356142845,
3.48133977663211));
#58416=CARTESIAN_POINT('Ctrl Pts',(-9.599046805007,-36.2742356137917,3.49799331944716));
#58417=CARTESIAN_POINT('Ctrl Pts',(-9.56787880217537,-36.2742356127846,
3.5320211248323));
#58418=CARTESIAN_POINT('Ctrl Pts',(-9.53575078071007,-36.2742356128432,
3.56552793219254));
#58419=CARTESIAN_POINT('Ctrl Pts',(-9.50271875164664,-36.2742356128141,
3.59827348432265));
#58420=CARTESIAN_POINT('Ctrl Pts',(-9.47108900403978,-36.2742356127862,
3.62962891656492));
#58421=CARTESIAN_POINT('Ctrl Pts',(-9.43863006930466,-36.2742356128,3.66028600049937));
#58422=CARTESIAN_POINT('Ctrl Pts',(-9.40543468805781,-36.2742356128,3.69004501056594));
#58423=CARTESIAN_POINT('Ctrl Pts',(-9.38837927873625,-36.2742356128,3.70533485146023));
#58424=CARTESIAN_POINT('Ctrl Pts',(-9.37111188743919,-36.2742356128,3.72040465547206));
#58425=CARTESIAN_POINT('Ctrl Pts',(-9.35361298710807,-36.2742356128,3.7352537065342));
#58426=CARTESIAN_POINT('Ctrl Pts',(-9.33611408677695,-36.2742356128,3.75010275759635));
#58427=CARTESIAN_POINT('Ctrl Pts',(-9.31839145737053,-36.2742356128,3.76472409613011));
#58428=CARTESIAN_POINT('Ctrl Pts',(-9.3004523225125,-36.2742356128,3.77909703529853));
#58429=CARTESIAN_POINT('Ctrl Pts',(-9.26457467434064,-36.2742356128,3.80784241565055));
#58430=CARTESIAN_POINT('Ctrl Pts',(-9.22782771264016,-36.2742356127664,
3.83559691701146));
#58431=CARTESIAN_POINT('Ctrl Pts',(-9.19027921250024,-36.2742356128789,
3.8622242824312));
#58432=CARTESIAN_POINT('Ctrl Pts',(-9.14099507705105,-36.2742356130266,
3.89717392566892));
#58433=CARTESIAN_POINT('Ctrl Pts',(-9.09031340536593,-36.2742356131635,
3.93018099942358));
#58434=CARTESIAN_POINT('Ctrl Pts',(-9.03839051489239,-36.2742356131207,
3.96101252749138));
#58435=CARTESIAN_POINT('Ctrl Pts',(-8.99022085714499,-36.2742356130811,
3.98961540651663));
#58436=CARTESIAN_POINT('Ctrl Pts',(-8.9409863450218,-36.2742356129554,4.01634539515136));
#58437=CARTESIAN_POINT('Ctrl Pts',(-8.89081544190779,-36.2742356128852,
4.04105717654398));
#58438=CARTESIAN_POINT('Ctrl Pts',(-8.84743531451334,-36.2742356128246,
4.06242414740595));
#58439=CARTESIAN_POINT('Ctrl Pts',(-8.80335630463337,-36.2742356128044,
4.0822825411275));
#58440=CARTESIAN_POINT('Ctrl Pts',(-8.75863697366334,-36.2742356128011,
4.10057022063283));
#58441=CARTESIAN_POINT('Ctrl Pts',(-8.74071780299924,-36.2742356127997,
4.10789814891347));
#58442=CARTESIAN_POINT('Ctrl Pts',(-8.72269543374841,-36.2742356128,4.11497425111613));
#58443=CARTESIAN_POINT('Ctrl Pts',(-8.70457175859042,-36.2742356128,4.12179612575218));
#58444=CARTESIAN_POINT('Ctrl Pts',(-8.6615121138754,-36.2742356128,4.13800406898433));
#58445=CARTESIAN_POINT('Ctrl Pts',(-8.61789280767915,-36.2742356128,4.15276924567355));
#58446=CARTESIAN_POINT('Ctrl Pts',(-8.5738109236211,-36.2742356128,4.16603168248515));
#58447=CARTESIAN_POINT('Ctrl Pts',(-8.5297290395644,-36.2742356128,4.17929411929633));
#58448=CARTESIAN_POINT('Ctrl Pts',(-8.48517579881231,-36.2742356128,4.19105632591689));
#58449=CARTESIAN_POINT('Ctrl Pts',(-8.44026209959521,-36.2742356128,4.20127113718018));
#58450=CARTESIAN_POINT('Ctrl Pts',(-8.38205916949961,-36.2742356128,4.21450834445235));
#58451=CARTESIAN_POINT('Ctrl Pts',(-8.32322710377887,-36.2742356127636,
4.22515208387702));
#58452=CARTESIAN_POINT('Ctrl Pts',(-8.26402667084017,-36.2742356128676,
4.23313872217696));
#58453=CARTESIAN_POINT('Ctrl Pts',(-8.23179791984128,-36.2742356129243,
4.23748665283067));
#58454=CARTESIAN_POINT('Ctrl Pts',(-8.19946018010296,-36.2742356130279,
4.24104800942531));
#58455=CARTESIAN_POINT('Ctrl Pts',(-8.16705632722208,-36.2742356133205,
4.24381893187712));
#58456=CARTESIAN_POINT('Ctrl Pts',(-8.12108841962377,-36.2742356137355,
4.24774974552742));
#58457=CARTESIAN_POINT('Ctrl Pts',(-8.07497261313446,-36.2742356144736,
4.25008843425972));
#58458=CARTESIAN_POINT('Ctrl Pts',(-8.0288281545193,-36.2742356152679,4.25083293408457));
#58459=CARTESIAN_POINT('Ctrl Pts',(-7.9826836958928,-36.2742356160621,4.25157743390961));
#58460=CARTESIAN_POINT('Ctrl Pts',(-7.93649883740971,-36.2742356168617,
4.250727941337));
#58461=CARTESIAN_POINT('Ctrl Pts',(-7.89039210993449,-36.2742356173469,
4.24829715711204));
#58462=CARTESIAN_POINT('Ctrl Pts',(-7.834906727744,-36.2742356179308,4.24537192257188));
#58463=CARTESIAN_POINT('Ctrl Pts',(-7.7794543674561,-36.2742356178824,4.24014910795062));
#58464=CARTESIAN_POINT('Ctrl Pts',(-7.72430050783329,-36.2742356176083,
4.23267735116746));
#58465=CARTESIAN_POINT('Ctrl Pts',(-7.68776143955221,-36.2742356174267,
4.22772736157206));
#58466=CARTESIAN_POINT('Ctrl Pts',(-7.65135327208932,-36.2742356171596,
4.22179141327856));
#58467=CARTESIAN_POINT('Ctrl Pts',(-7.6151500678385,-36.2742356169389,4.21489584135738));
#58468=CARTESIAN_POINT('Ctrl Pts',(-7.5697206010662,-36.2742356166621,4.20624295656578));
#58469=CARTESIAN_POINT('Ctrl Pts',(-7.52462017878676,-36.2742356157747,
4.19607685488961));
#58470=CARTESIAN_POINT('Ctrl Pts',(-7.47993901973256,-36.2742356147942,
4.18445357293978));
#58471=CARTESIAN_POINT('Ctrl Pts',(-7.43525786067835,-36.2742356138136,
4.17283029098994));
#58472=CARTESIAN_POINT('Ctrl Pts',(-7.3909849319815,-36.2742356131111,4.15974726321221));
#58473=CARTESIAN_POINT('Ctrl Pts',(-7.34717653623377,-36.2742356130129,
4.14527055133627));
#58474=CARTESIAN_POINT('Ctrl Pts',(-7.28763333788614,-36.2742356128795,
4.1255941922289));
#58475=CARTESIAN_POINT('Ctrl Pts',(-7.22891046922083,-36.2742356128427,
4.10330989587243));
#58476=CARTESIAN_POINT('Ctrl Pts',(-7.17122241053169,-36.2742356128223,
4.07858993246661));
#58477=CARTESIAN_POINT('Ctrl Pts',(-7.11432694101598,-36.2742356128022,
4.05420960218085));
#58478=CARTESIAN_POINT('Ctrl Pts',(-7.05843851288911,-36.2742356128016,
4.02746041159676));
#58479=CARTESIAN_POINT('Ctrl Pts',(-7.00372558585949,-36.2742356128006,
3.99854144870779));
#58480=CARTESIAN_POINT('Ctrl Pts',(-6.95016215270973,-36.2742356127996,
3.97023006016474));
#58481=CARTESIAN_POINT('Ctrl Pts',(-6.89772568521568,-36.2742356128,3.93983946721879));
#58482=CARTESIAN_POINT('Ctrl Pts',(-6.84653239340986,-36.2742356128,3.90758397389369));
#58483=CARTESIAN_POINT('Ctrl Pts',(-6.83371007465548,-36.2742356128,3.89950498146314));
#58484=CARTESIAN_POINT('Ctrl Pts',(-6.82096552334532,-36.2742356128,3.891309118064));
#58485=CARTESIAN_POINT('Ctrl Pts',(-6.8083001050419,-36.2742356128,3.88299998927819));
#58486=CARTESIAN_POINT('Ctrl Pts',(-6.80264328257797,-36.2742356128,3.87928883933863));
#58487=CARTESIAN_POINT('Ctrl Pts',(-6.79699868907667,-36.2742356128,3.87555272110333));
#58488=CARTESIAN_POINT('Ctrl Pts',(-6.79137755926,-36.2742356128,3.87179939627));
#58489=CARTESIAN_POINT('',(-5.86597168177314,-36.2742356128,4.46707928587636));
#58490=CARTESIAN_POINT('Ctrl Pts',(-6.79137755835672,-36.2742356128,3.87179939762279));
#58491=CARTESIAN_POINT('Ctrl Pts',(-6.76761184639918,-36.2742356128,3.85593061410674));
#58492=CARTESIAN_POINT('Ctrl Pts',(-6.74270438593246,-36.2742356128002,
3.84174534933221));
#58493=CARTESIAN_POINT('Ctrl Pts',(-6.71690530938368,-36.2742356128077,
3.82940307968605));
#58494=CARTESIAN_POINT('Ctrl Pts',(-6.69055450068662,-36.2742356128154,
3.81679686156354));
#58495=CARTESIAN_POINT('Ctrl Pts',(-6.66327401414774,-36.2742356128296,
3.80611343344803));
#58496=CARTESIAN_POINT('Ctrl Pts',(-6.63535439365547,-36.2742356128256,
3.797474184043));
#58497=CARTESIAN_POINT('Ctrl Pts',(-6.62783704541903,-36.2742356128245,
3.7951480691054));
#58498=CARTESIAN_POINT('Ctrl Pts',(-6.62027347180955,-36.2742356128222,
3.79296987495101));
#58499=CARTESIAN_POINT('Ctrl Pts',(-6.61266956107909,-36.2742356128189,
3.79094136987596));
#58500=CARTESIAN_POINT('Ctrl Pts',(-6.58404678702163,-36.2742356128064,
3.7833056355156));
#58501=CARTESIAN_POINT('Ctrl Pts',(-6.5548544424529,-36.2742356128063,3.77779824758968));
#58502=CARTESIAN_POINT('Ctrl Pts',(-6.52541631983754,-36.274235612809,3.77448101612473));
#58503=CARTESIAN_POINT('Ctrl Pts',(-6.49579762225793,-36.2742356128117,
3.77114343659068));
#58504=CARTESIAN_POINT('Ctrl Pts',(-6.4659307586813,-36.2742356128191,3.77002298684856));
#58505=CARTESIAN_POINT('Ctrl Pts',(-6.43615056222019,-36.2742356128416,
3.77113037025664));
#58506=CARTESIAN_POINT('Ctrl Pts',(-6.42803345799806,-36.2742356128477,
3.77143220663132));
#58507=CARTESIAN_POINT('Ctrl Pts',(-6.41992279052018,-36.274235612855,3.77189925623979));
#58508=CARTESIAN_POINT('Ctrl Pts',(-6.41182530777443,-36.2742356128637,
3.77253106516291));
#58509=CARTESIAN_POINT('Ctrl Pts',(-6.38224976818375,-36.2742356128954,
3.77483870698273));
#58510=CARTESIAN_POINT('Ctrl Pts',(-6.35285068902878,-36.2742356128708,
3.77934535731408));
#58511=CARTESIAN_POINT('Ctrl Pts',(-6.32395091201471,-36.2742356128434,
3.78599870729406));
#58512=CARTESIAN_POINT('Ctrl Pts',(-6.29548019782323,-36.2742356128164,
3.79255327778794));
#58513=CARTESIAN_POINT('Ctrl Pts',(-6.26749464288281,-36.2742356128016,
3.8011911613719));
#58514=CARTESIAN_POINT('Ctrl Pts',(-6.24028833581526,-36.2742356128003,
3.81181401814056));
#58515=CARTESIAN_POINT('Ctrl Pts',(-6.23221871909247,-36.2742356127999,
3.8149648457193));
#58516=CARTESIAN_POINT('Ctrl Pts',(-6.22421752784224,-36.2742356128,3.81828998335235));
#58517=CARTESIAN_POINT('Ctrl Pts',(-6.21629207071364,-36.2742356128,3.82178605280247));
#58518=CARTESIAN_POINT('Ctrl Pts',(-6.18903048380091,-36.2742356128,3.83381165582083));
#58519=CARTESIAN_POINT('Ctrl Pts',(-6.16266648013035,-36.2742356128015,
3.84786387672877));
#58520=CARTESIAN_POINT('Ctrl Pts',(-6.13748779945074,-36.2742356128333,
3.86379149731598));
#58521=CARTESIAN_POINT('Ctrl Pts',(-6.11197343727939,-36.2742356128655,
3.87993146451129));
#58522=CARTESIAN_POINT('Ctrl Pts',(-6.08767667101957,-36.2742356129214,
3.89799683301395));
#58523=CARTESIAN_POINT('Ctrl Pts',(-6.0648706288655,-36.2742356128984,3.91778392372097));
#58524=CARTESIAN_POINT('Ctrl Pts',(-6.05935038385834,-36.2742356128928,
3.92257342590393));
#58525=CARTESIAN_POINT('Ctrl Pts',(-6.05391734170426,-36.274235612883,3.92746360531471));
#58526=CARTESIAN_POINT('Ctrl Pts',(-6.04857510195205,-36.2742356128702,
3.93245120810224));
#58527=CARTESIAN_POINT('Ctrl Pts',(-6.02628005996784,-36.274235612817,3.95326622553057));
#58528=CARTESIAN_POINT('Ctrl Pts',(-6.00557086076768,-36.2742356128086,
3.97578568705138));
#58529=CARTESIAN_POINT('Ctrl Pts',(-5.98668919867165,-36.2742356128037,
3.99975188059635));
#58530=CARTESIAN_POINT('Ctrl Pts',(-5.96788968088333,-36.2742356127989,
4.02361380967733));
#58531=CARTESIAN_POINT('Ctrl Pts',(-5.95090221910612,-36.2742356128,4.04890948259598));
#58532=CARTESIAN_POINT('Ctrl Pts',(-5.93592640503596,-36.2742356128,4.0753508284618));
#58533=CARTESIAN_POINT('Ctrl Pts',(-5.9327569959689,-36.2742356128,4.08094674738412));
#58534=CARTESIAN_POINT('Ctrl Pts',(-5.92967753613311,-36.2742356128,4.08659387281414));
#58535=CARTESIAN_POINT('Ctrl Pts',(-5.92668966701898,-36.2742356128,4.09228930726427));
#58536=CARTESIAN_POINT('Ctrl Pts',(-5.91288634093118,-36.2742356128,4.11860101501454));
#58537=CARTESIAN_POINT('Ctrl Pts',(-5.90104238722179,-36.2742356127986,
4.14594540821402));
#58538=CARTESIAN_POINT('Ctrl Pts',(-5.89129324247737,-36.2742356128083,
4.17401939030619));
#58539=CARTESIAN_POINT('Ctrl Pts',(-5.88170403456135,-36.2742356128179,
4.20163281264937));
#58540=CARTESIAN_POINT('Ctrl Pts',(-5.87414169718084,-36.2742356128408,
4.22995165567001));
#58541=CARTESIAN_POINT('Ctrl Pts',(-5.86868793689861,-36.2742356128729,
4.25866970663748));
#58542=CARTESIAN_POINT('Ctrl Pts',(-5.86707823012509,-36.2742356128823,
4.26714599433122));
#58543=CARTESIAN_POINT('Ctrl Pts',(-5.86565188625897,-36.2742356128923,
4.27565696309787));
#58544=CARTESIAN_POINT('Ctrl Pts',(-5.86441015811822,-36.2742356129023,
4.28419451843095));
#58545=CARTESIAN_POINT('Ctrl Pts',(-5.86024059061394,-36.2742356129359,
4.31286255945746));
#58546=CARTESIAN_POINT('Ctrl Pts',(-5.85815474191147,-36.2742356128985,
4.34182710763987));
#58547=CARTESIAN_POINT('Ctrl Pts',(-5.85816763299558,-36.2742356128601,
4.37078377328871));
#58548=CARTESIAN_POINT('Ctrl Pts',(-5.85817731164302,-36.2742356128313,
4.39252448611661));
#58549=CARTESIAN_POINT('Ctrl Pts',(-5.85936912895101,-36.2742356128086,
4.41426052100927));
#58550=CARTESIAN_POINT('Ctrl Pts',(-5.86173021509392,-36.2742356128025,
4.43586047460259));
#58551=CARTESIAN_POINT('Ctrl Pts',(-5.8626477852411,-36.2742356128001,4.44425469294026));
#58552=CARTESIAN_POINT('Ctrl Pts',(-5.8637420657599,-36.2742356128,4.45263000166015));
#58553=CARTESIAN_POINT('Ctrl Pts',(-5.86501138994113,-36.2742356128,4.46097597332566));
#58554=CARTESIAN_POINT('Ctrl Pts',(-5.86532105398436,-36.2742356128,4.4630120547057));
#58555=CARTESIAN_POINT('Ctrl Pts',(-5.86564124357689,-36.2742356128,4.46504699468167));
#58556=CARTESIAN_POINT('Ctrl Pts',(-5.86597166755,-36.2742356128,4.4670791984));
#58557=CARTESIAN_POINT('',(2.00400681001E-5,-36.2742356128,11.3643459915));
#58558=CARTESIAN_POINT('Ctrl Pts',(-5.86597169611384,-36.2742356128,4.46707937407566));
#58559=CARTESIAN_POINT('Ctrl Pts',(-5.8917537841064,-36.2742356128,4.62564653271355));
#58560=CARTESIAN_POINT('Ctrl Pts',(-5.91113350168116,-36.2742356127996,
4.78526058020349));
#58561=CARTESIAN_POINT('Ctrl Pts',(-5.92402582739545,-36.2742356128017,
4.9453930553239));
#58562=CARTESIAN_POINT('Ctrl Pts',(-5.93703567776282,-36.2742356128039,
5.10698527587751));
#58563=CARTESIAN_POINT('Ctrl Pts',(-5.94343938459977,-36.2742356128092,
5.26910521717685));
#58564=CARTESIAN_POINT('Ctrl Pts',(-5.94320281925437,-36.2742356128227,
5.43120865955647));
#58565=CARTESIAN_POINT('Ctrl Pts',(-5.94296301946909,-36.2742356128364,
5.59552846138439));
#58566=CARTESIAN_POINT('Ctrl Pts',(-5.9359001599745,-36.2742356128589,5.75983108901504));
#58567=CARTESIAN_POINT('Ctrl Pts',(-5.92203248068316,-36.2742356128929,
5.92355170789826));
#58568=CARTESIAN_POINT('Ctrl Pts',(-5.90806831172284,-36.2742356129272,
6.08841147544444));
#58569=CARTESIAN_POINT('Ctrl Pts',(-5.88720439804731,-36.2742356129733,
6.25268087420031));
#58570=CARTESIAN_POINT('Ctrl Pts',(-5.85951245233149,-36.2742356130288,
6.41578866465459));
#58571=CARTESIAN_POINT('Ctrl Pts',(-5.83153691837167,-36.2742356130848,
6.58056681270492));
#58572=CARTESIAN_POINT('Ctrl Pts',(-5.79659286542048,-36.2742356131502,
6.74415918610583));
#58573=CARTESIAN_POINT('Ctrl Pts',(-5.75480692584564,-36.2742356132163,
6.90598606231219));
#58574=CARTESIAN_POINT('Ctrl Pts',(-5.71753047360896,-36.2742356132753,
7.05034878055894));
#58575=CARTESIAN_POINT('Ctrl Pts',(-5.67480998545357,-36.2742356133345,
7.19330651107798));
#58576=CARTESIAN_POINT('Ctrl Pts',(-5.6267692791197,-36.274235613385,7.334456277306));
#58577=CARTESIAN_POINT('Ctrl Pts',(-5.57231694921545,-36.2742356134422,
7.49444421718227));
#58578=CARTESIAN_POINT('Ctrl Pts',(-5.51102853554952,-36.2742356134451,
7.65210758867517));
#58579=CARTESIAN_POINT('Ctrl Pts',(-5.44313216551832,-36.2742356134085,
7.80687595572862));
#58580=CARTESIAN_POINT('Ctrl Pts',(-5.37497521134488,-36.2742356133719,
7.96223831892878));
#58581=CARTESIAN_POINT('Ctrl Pts',(-5.30015963440195,-36.2742356132978,
8.11468314343555));
#58582=CARTESIAN_POINT('Ctrl Pts',(-5.21896431965411,-36.274235613218,8.26365448761046));
#58583=CARTESIAN_POINT('Ctrl Pts',(-5.13753259016911,-36.274235613138,8.4130595886011));
#58584=CARTESIAN_POINT('Ctrl Pts',(-5.0496840815577,-36.2742356130535,8.55897068001005));
#58585=CARTESIAN_POINT('Ctrl Pts',(-4.95574602924874,-36.2742356129869,
8.70085219792462));
#58586=CARTESIAN_POINT('Ctrl Pts',(-4.86181143441669,-36.2742356129203,
8.84272849375868));
#58587=CARTESIAN_POINT('Ctrl Pts',(-4.76178793134922,-36.2742356128717,
8.98057525162899));
#58588=CARTESIAN_POINT('Ctrl Pts',(-4.65604588330678,-36.2742356128431,
9.11388616448563));
#58589=CARTESIAN_POINT('Ctrl Pts',(-4.55056648084933,-36.2742356128146,
9.24686595530198));
#58590=CARTESIAN_POINT('Ctrl Pts',(-4.4393971075515,-36.2742356128051,9.37533216035669));
#58591=CARTESIAN_POINT('Ctrl Pts',(-4.32294538768296,-36.2742356128018,
9.49881506179245));
#58592=CARTESIAN_POINT('Ctrl Pts',(-4.23823731799389,-36.2742356127995,
9.58863767868498));
#58593=CARTESIAN_POINT('Ctrl Pts',(-4.15073506984275,-36.2742356128,9.67582417482043));
#58594=CARTESIAN_POINT('Ctrl Pts',(-4.06060797518421,-36.2742356128,9.76020584146258));
#58595=CARTESIAN_POINT('Ctrl Pts',(-3.93701288663076,-36.2742356128,9.87592198210191));
#58596=CARTESIAN_POINT('Ctrl Pts',(-3.80848026352504,-36.2742356128,9.98636089573716));
#58597=CARTESIAN_POINT('Ctrl Pts',(-3.67547833414633,-36.2742356128,10.0911139764056));
#58598=CARTESIAN_POINT('Ctrl Pts',(-3.54294605058195,-36.2742356128,10.1954971613431));
#58599=CARTESIAN_POINT('Ctrl Pts',(-3.40597617606029,-36.2742356128,10.2942344499813));
#58600=CARTESIAN_POINT('Ctrl Pts',(-3.26506202837529,-36.2742356128,10.3869635798179));
#58601=CARTESIAN_POINT('Ctrl Pts',(-3.12463152047159,-36.2742356128,10.479374448523));
#58602=CARTESIAN_POINT('Ctrl Pts',(-2.98028396985441,-36.2742356128001,
10.5658181858481));
#58603=CARTESIAN_POINT('Ctrl Pts',(-2.83253445146773,-36.2742356128001,
10.6459802356601));
#58604=CARTESIAN_POINT('Ctrl Pts',(-2.68541849570139,-36.2742356128001,
10.72579854372));
#58605=CARTESIAN_POINT('Ctrl Pts',(-2.5349298855088,-36.2742356128002,10.7993887888944));
#58606=CARTESIAN_POINT('Ctrl Pts',(-2.38160072644212,-36.2742356128002,
10.8664861850762));
#58607=CARTESIAN_POINT('Ctrl Pts',(-2.22904444720905,-36.2742356128002,
10.9332453662393));
#58608=CARTESIAN_POINT('Ctrl Pts',(-2.0736763794413,-36.2742356128003,10.9935768682926));
#58609=CARTESIAN_POINT('Ctrl Pts',(-1.91604110659622,-36.2742356128003,
11.0472671542599));
#58610=CARTESIAN_POINT('Ctrl Pts',(-1.75983755284287,-36.2742356128003,
11.1004697993199));
#58611=CARTESIAN_POINT('Ctrl Pts',(-1.60140798882314,-36.2742356128004,
11.1471512359842));
#58612=CARTESIAN_POINT('Ctrl Pts',(-1.44129950961667,-36.2742356128003,
11.1871516829491));
#58613=CARTESIAN_POINT('Ctrl Pts',(-1.28207456984831,-36.2742356128003,
11.2269313922454));
#58614=CARTESIAN_POINT('Ctrl Pts',(-1.12118937306491,-36.2742356128003,
11.2601035402185));
#58615=CARTESIAN_POINT('Ctrl Pts',(-0.959196318817928,-36.2742356128003,
11.286560085187));
#58616=CARTESIAN_POINT('Ctrl Pts',(-0.798772591246272,-36.2742356128002,
11.3127603292791));
#58617=CARTESIAN_POINT('Ctrl Pts',(-0.637262545229791,-36.2742356128002,
11.3323743934019));
#58618=CARTESIAN_POINT('Ctrl Pts',(-0.475214087498627,-36.2742356128001,
11.34534683313));
#58619=CARTESIAN_POINT('Ctrl Pts',(-0.318810407195243,-36.2742356128,11.3578673923775));
#58620=CARTESIAN_POINT('Ctrl Pts',(-0.161905358524558,-36.2742356128,11.3642011232218));
#58621=CARTESIAN_POINT('Ctrl Pts',(-0.00499952426527361,-36.2742356128,
11.3643435450127));
#58622=CARTESIAN_POINT('Ctrl Pts',(-0.00332634407496558,-36.2742356128,
11.364345063741));
#58623=CARTESIAN_POINT('Ctrl Pts',(-0.00165316357213757,-36.2742356128,
11.3643458788333));
#58624=CARTESIAN_POINT('Ctrl Pts',(2.00400681000801E-5,-36.2742356128,11.3643459915));
#58625=CARTESIAN_POINT('',(5.86597167565,-36.2742356128,4.4670793309));
#58626=CARTESIAN_POINT('Ctrl Pts',(2.0040068100144E-5,-36.2742356128,11.3643459915));
#58627=CARTESIAN_POINT('Ctrl Pts',(0.160669261245717,-36.2742356128,11.3643342068985));
#58628=CARTESIAN_POINT('Ctrl Pts',(0.321323836354438,-36.2742356127995,
11.3578350469369));
#58629=CARTESIAN_POINT('Ctrl Pts',(0.48144851078575,-36.2742356128017,11.3448494418734));
#58630=CARTESIAN_POINT('Ctrl Pts',(0.643032821894107,-36.2742356128039,
11.3317454648881));
#58631=CARTESIAN_POINT('Ctrl Pts',(0.804077338593767,-36.2742356128091,
11.3120363431189));
#58632=CARTESIAN_POINT('Ctrl Pts',(0.96403942366694,-36.2742356128227,11.2857757694845));
#58633=CARTESIAN_POINT('Ctrl Pts',(1.12618852773305,-36.2742356128364,11.2591561584365));
#58634=CARTESIAN_POINT('Ctrl Pts',(1.28722518656786,-36.2742356128588,11.2258047936747));
#58635=CARTESIAN_POINT('Ctrl Pts',(1.44659482423436,-36.2742356128929,11.1858303670584));
#58636=CARTESIAN_POINT('Ctrl Pts',(1.60707331376536,-36.2742356129272,11.1455778089351));
#58637=CARTESIAN_POINT('Ctrl Pts',(1.76586129014309,-36.2742356129733,11.0986098401703));
#58638=CARTESIAN_POINT('Ctrl Pts',(1.92240644122734,-36.2742356130288,11.0450889599348));
#58639=CARTESIAN_POINT('Ctrl Pts',(2.08055469303748,-36.2742356130848,10.9910199990889));
#58640=CARTESIAN_POINT('Ctrl Pts',(2.23641371203394,-36.2742356131502,10.9302633474154));
#58641=CARTESIAN_POINT('Ctrl Pts',(2.38943163147733,-36.2742356132163,10.8630370730498));
#58642=CARTESIAN_POINT('Ctrl Pts',(2.52592578651562,-36.2742356132753,10.8030702825635));
#58643=CARTESIAN_POINT('Ctrl Pts',(2.66015944790375,-36.2742356133345,10.7379564690856));
#58644=CARTESIAN_POINT('Ctrl Pts',(2.79175483379253,-36.274235613385,10.6678825015028));
#58645=CARTESIAN_POINT('Ctrl Pts',(2.94092485046201,-36.2742356134422,10.5884501198747));
#58646=CARTESIAN_POINT('Ctrl Pts',(3.08670290511894,-36.2742356134451,10.5026435517876));
#58647=CARTESIAN_POINT('Ctrl Pts',(3.22856258818739,-36.2742356134085,10.4107795500798));
#58648=CARTESIAN_POINT('Ctrl Pts',(3.3709667242985,-36.2742356133719,10.3185629771964));
#58649=CARTESIAN_POINT('Ctrl Pts',(3.50942211228398,-36.2742356132978,10.2202425794934));
#58650=CARTESIAN_POINT('Ctrl Pts',(3.6434247982021,-36.274235613218,10.1161828818025));
#58651=CARTESIAN_POINT('Ctrl Pts',(3.77781765702698,-36.274235613138,10.0118201955973));
#58652=CARTESIAN_POINT('Ctrl Pts',(3.90773160377994,-36.2742356130535,9.90168494462553));
#58653=CARTESIAN_POINT('Ctrl Pts',(4.03269056067304,-36.2742356129869,9.78618610525616));
#58654=CARTESIAN_POINT('Ctrl Pts',(4.15764491834771,-36.2742356129203,9.67069151691772));
#58655=CARTESIAN_POINT('Ctrl Pts',(4.27764442325623,-36.2742356128717,9.54983396169469));
#58656=CARTESIAN_POINT('Ctrl Pts',(4.39224879920933,-36.2742356128431,9.42406028704545));
#58657=CARTESIAN_POINT('Ctrl Pts',(4.50656851704689,-36.2742356128146,9.29859901318294));
#58658=CARTESIAN_POINT('Ctrl Pts',(4.61551966406313,-36.2742356128051,9.16824624956892));
#58659=CARTESIAN_POINT('Ctrl Pts',(4.71870406094502,-36.2742356128018,9.0334797468142));
#58660=CARTESIAN_POINT('Ctrl Pts',(4.79376135581583,-36.2742356127995,8.93544933289853));
#58661=CARTESIAN_POINT('Ctrl Pts',(4.86576811547973,-36.2742356128,8.8350842239588));
#58662=CARTESIAN_POINT('Ctrl Pts',(4.93458500645283,-36.2742356128,8.73257864184937));
#58663=CARTESIAN_POINT('Ctrl Pts',(5.02895651343094,-36.2742356128,8.59200841089956));
#58664=CARTESIAN_POINT('Ctrl Pts',(5.11732652024821,-36.2742356128,8.44741196978782));
#58665=CARTESIAN_POINT('Ctrl Pts',(5.19936689681885,-36.2742356128,8.29931707527905));
#58666=CARTESIAN_POINT('Ctrl Pts',(5.2811175789149,-36.2742356128,8.15174512172261));
#58667=CARTESIAN_POINT('Ctrl Pts',(5.35658314132099,-36.2742356128,8.00069960672827));
#58668=CARTESIAN_POINT('Ctrl Pts',(5.42548522439472,-36.2742356128,7.84672561054384));
#58669=CARTESIAN_POINT('Ctrl Pts',(5.49415082453722,-36.2742356128,7.69328007765586));
#58670=CARTESIAN_POINT('Ctrl Pts',(5.55629781244997,-36.2742356128001,7.53692635372705));
#58671=CARTESIAN_POINT('Ctrl Pts',(5.61169840914281,-36.2742356128001,7.37822333453516));
#58672=CARTESIAN_POINT('Ctrl Pts',(5.66686144330851,-36.2742356128001,7.22020084754966));
#58673=CARTESIAN_POINT('Ctrl Pts',(5.71533572155684,-36.2742356128002,7.05984938881124));
#58674=CARTESIAN_POINT('Ctrl Pts',(5.75694532357763,-36.2742356128002,6.89773667307677));
#58675=CARTESIAN_POINT('Ctrl Pts',(5.79834518582213,-36.2742356128002,6.73644111211145));
#58676=CARTESIAN_POINT('Ctrl Pts',(5.83294931383753,-36.2742356128003,6.57340221821182));
#58677=CARTESIAN_POINT('Ctrl Pts',(5.86063437496362,-36.2742356128003,6.40919179399785));
#58678=CARTESIAN_POINT('Ctrl Pts',(5.88806798709023,-36.2742356128003,6.24647280759158));
#58679=CARTESIAN_POINT('Ctrl Pts',(5.90870759712497,-36.2742356128004,6.08260368375527));
#58680=CARTESIAN_POINT('Ctrl Pts',(5.92248333397203,-36.2742356128003,5.91815007354724));
#58681=CARTESIAN_POINT('Ctrl Pts',(5.93618305106614,-36.2742356128003,5.75460398087947));
#58682=CARTESIAN_POINT('Ctrl Pts',(5.94309436640146,-36.2742356128003,5.59048002886484));
#58683=CARTESIAN_POINT('Ctrl Pts',(5.9431993289485,-36.2742356128003,5.42634079730078));
#58684=CARTESIAN_POINT('Ctrl Pts',(5.94330327465857,-36.2742356128002,5.26379168378016));
#58685=CARTESIAN_POINT('Ctrl Pts',(5.93673206979469,-36.2742356128002,5.10122777113394));
#58686=CARTESIAN_POINT('Ctrl Pts',(5.92351895692325,-36.2742356128001,4.93919876000739));
#58687=CARTESIAN_POINT('Ctrl Pts',(5.91076610807552,-36.2742356128,4.78281384844637));
#58688=CARTESIAN_POINT('Ctrl Pts',(5.89182619464975,-36.2742356128,4.62692738262583));
#58689=CARTESIAN_POINT('Ctrl Pts',(5.86677516387858,-36.2742356128,4.47203417080732));
#58690=CARTESIAN_POINT('Ctrl Pts',(5.866508029849,-36.2742356128,4.47038245243268));
#58691=CARTESIAN_POINT('Ctrl Pts',(5.86624020126667,-36.2742356128,4.4687308467));
#58692=CARTESIAN_POINT('Ctrl Pts',(5.86597167565,-36.2742356128,4.4670793309));
#58693=CARTESIAN_POINT('',(6.79137814945778,-36.2742356128,3.87179980964612));
#58694=CARTESIAN_POINT('Ctrl Pts',(5.86597167565,-36.2742356128,4.4670793309));
#58695=CARTESIAN_POINT('Ctrl Pts',(5.86138310686398,-36.2742356128,4.43885832277569));
#58696=CARTESIAN_POINT('Ctrl Pts',(5.85880207480769,-36.2742356128002,4.41029637378214));
#58697=CARTESIAN_POINT('Ctrl Pts',(5.85826991574712,-36.2742356128077,4.38168750048739));
#58698=CARTESIAN_POINT('Ctrl Pts',(5.85772633902877,-36.2742356128154,4.35246481386365));
#58699=CARTESIAN_POINT('Ctrl Pts',(5.85932040979103,-36.2742356128296,4.32319365636273));
#58700=CARTESIAN_POINT('Ctrl Pts',(5.86304204786118,-36.2742356128256,4.29418908540444));
#58701=CARTESIAN_POINT('Ctrl Pts',(5.86403957209765,-36.2742356128245,4.28641488437951));
#58702=CARTESIAN_POINT('Ctrl Pts',(5.86518965424346,-36.2742356128222,4.27865982151693));
#58703=CARTESIAN_POINT('Ctrl Pts',(5.86649147241364,-36.2742356128189,4.27092991253681));
#58704=CARTESIAN_POINT('Ctrl Pts',(5.87141122237932,-36.2742356128064,4.24171752304138));
#58705=CARTESIAN_POINT('Ctrl Pts',(5.87850390340837,-36.2742356128063,4.2128693309871));
#58706=CARTESIAN_POINT('Ctrl Pts',(5.887691504304,-36.274235612809,4.18470561171533));
#58707=CARTESIAN_POINT('Ctrl Pts',(5.89693546242266,-36.2742356128117,4.15636913472078));
#58708=CARTESIAN_POINT('Ctrl Pts',(5.90829987588764,-36.2742356128191,4.12872614174051));
#58709=CARTESIAN_POINT('Ctrl Pts',(5.92165564928313,-36.2742356128416,4.10208576405828));
#58710=CARTESIAN_POINT('Ctrl Pts',(5.92529599468891,-36.2742356128477,4.09482447160953));
#58711=CARTESIAN_POINT('Ctrl Pts',(5.92908401278061,-36.274235612855,4.08763754057056));
#58712=CARTESIAN_POINT('Ctrl Pts',(5.93301649251076,-36.2742356128637,4.080530923298));
#58713=CARTESIAN_POINT('Ctrl Pts',(5.9473796244506,-36.2742356128954,4.05457445599592));
#58714=CARTESIAN_POINT('Ctrl Pts',(5.96367065437727,-36.2742356128708,4.02969036273551));
#58715=CARTESIAN_POINT('Ctrl Pts',(5.98170811879717,-36.2742356128434,4.00615073538495));
#58716=CARTESIAN_POINT('Ctrl Pts',(5.99947778858028,-36.2742356128164,3.98296059096665));
#58717=CARTESIAN_POINT('Ctrl Pts',(6.0189420762282,-36.2742356128016,3.96107576001189));
#58718=CARTESIAN_POINT('Ctrl Pts',(6.0398895528597,-36.2742356128003,3.94072308317647));
#58719=CARTESIAN_POINT('Ctrl Pts',(6.04610274843812,-36.2742356127999,3.93468631015854));
#58720=CARTESIAN_POINT('Ctrl Pts',(6.05244619165565,-36.2742356128,3.92878407929817));
#58721=CARTESIAN_POINT('Ctrl Pts',(6.0589137779052,-36.2742356128,3.92302164060569));
#58722=CARTESIAN_POINT('Ctrl Pts',(6.08116065440074,-36.2742356128,3.90320029505909));
#58723=CARTESIAN_POINT('Ctrl Pts',(6.10487954933902,-36.2742356128015,3.88503605466741));
#58724=CARTESIAN_POINT('Ctrl Pts',(6.12981354785304,-36.2742356128333,3.86872805722725));
#58725=CARTESIAN_POINT('Ctrl Pts',(6.15507996575881,-36.2742356128655,3.85220264200764));
#58726=CARTESIAN_POINT('Ctrl Pts',(6.1815936063361,-36.2742356129214,3.83758357031686));
#58727=CARTESIAN_POINT('Ctrl Pts',(6.20905587461221,-36.2742356128984,3.82503493124853));
#58728=CARTESIAN_POINT('Ctrl Pts',(6.21570316769405,-36.2742356128928,3.8219975098372));
#58729=CARTESIAN_POINT('Ctrl Pts',(6.22240591775922,-36.274235612883,3.81908118658232));
#58730=CARTESIAN_POINT('Ctrl Pts',(6.22915967133299,-36.2742356128702,3.81628788784265));
#58731=CARTESIAN_POINT('Ctrl Pts',(6.25734545658257,-36.274235612817,3.80463047133284));
#58732=CARTESIAN_POINT('Ctrl Pts',(6.28642470665912,-36.2742356128086,3.79512287984581));
#58733=CARTESIAN_POINT('Ctrl Pts',(6.31606269113364,-36.2742356128037,3.78787819386153));
#58734=CARTESIAN_POINT('Ctrl Pts',(6.34557173612636,-36.2742356127989,3.78066502574437));
#58735=CARTESIAN_POINT('Ctrl Pts',(6.37563411554278,-36.2742356128,3.77569529013553));
#58736=CARTESIAN_POINT('Ctrl Pts',(6.40590493031561,-36.2742356128,3.7730311667504));
#58737=CARTESIAN_POINT('Ctrl Pts',(6.41231129949293,-36.2742356128,3.77246734453197));
#58738=CARTESIAN_POINT('Ctrl Pts',(6.41872696926415,-36.2742356128,3.77200660708024));
#58739=CARTESIAN_POINT('Ctrl Pts',(6.42514862232994,-36.2742356128,3.77164924671227));
#58740=CARTESIAN_POINT('Ctrl Pts',(6.45481530760457,-36.2742356128,3.76999831704387));
#58741=CARTESIAN_POINT('Ctrl Pts',(6.48460928672341,-36.2742356127986,3.77055858065525));
#58742=CARTESIAN_POINT('Ctrl Pts',(6.51419858877646,-36.2742356128083,3.77332760680242));
#58743=CARTESIAN_POINT('Ctrl Pts',(6.54330247191718,-36.2742356128179,3.77605120647559));
#58744=CARTESIAN_POINT('Ctrl Pts',(6.57220785528294,-36.2742356128408,3.78091172458778));
#58745=CARTESIAN_POINT('Ctrl Pts',(6.60060221092621,-36.2742356128729,3.78785654476743));
#58746=CARTESIAN_POINT('Ctrl Pts',(6.60898295791085,-36.2742356128823,3.78990634584448));
#58747=CARTESIAN_POINT('Ctrl Pts',(6.61731923451022,-36.2742356128923,3.79213738464737));
#58748=CARTESIAN_POINT('Ctrl Pts',(6.62560315537363,-36.2742356129023,3.79454744491348));
#58749=CARTESIAN_POINT('Ctrl Pts',(6.65341952465768,-36.2742356129359,3.80264012559749));
#58750=CARTESIAN_POINT('Ctrl Pts',(6.68064171724888,-36.2742356128985,3.81275190378225));
#58751=CARTESIAN_POINT('Ctrl Pts',(6.70698651466996,-36.2742356128601,3.8247702360994));
#58752=CARTESIAN_POINT('Ctrl Pts',(6.72676623217281,-36.2742356128313,3.83379361989275));
#58753=CARTESIAN_POINT('Ctrl Pts',(6.74605153046156,-36.2742356128086,3.84389079290531));
#58754=CARTESIAN_POINT('Ctrl Pts',(6.76472817074846,-36.2742356128025,3.85499555865129));
#58755=CARTESIAN_POINT('Ctrl Pts',(6.77198632512756,-36.2742356128001,3.85931111556571));
#58756=CARTESIAN_POINT('Ctrl Pts',(6.77915400078233,-36.2742356128,3.86377963564129));
#58757=CARTESIAN_POINT('Ctrl Pts',(6.78622239998195,-36.2742356128,3.86839527856917));
#58758=CARTESIAN_POINT('Ctrl Pts',(6.78794680506907,-36.2742356128,3.86952130978507));
#58759=CARTESIAN_POINT('Ctrl Pts',(6.78966580718133,-36.2742356128,3.87065644581633));
#58760=CARTESIAN_POINT('Ctrl Pts',(6.79137807575,-36.2742356128,3.87179976043));
#58761=CARTESIAN_POINT('',(10.0697218907767,-36.2742356128,2.85693873298755));
#58762=CARTESIAN_POINT('Ctrl Pts',(6.79137822377471,-36.2742356128,3.871799859269));
#58763=CARTESIAN_POINT('Ctrl Pts',(6.84151938457836,-36.2742356128,3.90528008500436));
#58764=CARTESIAN_POINT('Ctrl Pts',(6.89293658842097,-36.2742356128,3.93699461273041));
#58765=CARTESIAN_POINT('Ctrl Pts',(6.94552480855072,-36.2742356128,3.96671973257289));
#58766=CARTESIAN_POINT('Ctrl Pts',(6.99923060295532,-36.2742356128,3.9970765533775));
#58767=CARTESIAN_POINT('Ctrl Pts',(7.05415741161727,-36.2742356128,4.02535798824697));
#58768=CARTESIAN_POINT('Ctrl Pts',(7.11014444075754,-36.2742356128,4.05135152058415));
#58769=CARTESIAN_POINT('Ctrl Pts',(7.16613146989781,-36.2742356128,4.07734505292132));
#58770=CARTESIAN_POINT('Ctrl Pts',(7.22317817849455,-36.2742356128,4.10105026459671));
#58771=CARTESIAN_POINT('Ctrl Pts',(7.28108200924425,-36.2742356128,4.12228714148679));
#58772=CARTESIAN_POINT('Ctrl Pts',(7.32228977760065,-36.2742356128,4.13740055094812));
#58773=CARTESIAN_POINT('Ctrl Pts',(7.36394849294144,-36.2742356128,4.15127161584809));
#58774=CARTESIAN_POINT('Ctrl Pts',(7.40600132539777,-36.2742356128,4.16384980223352));
#58775=CARTESIAN_POINT('Ctrl Pts',(7.44515714624124,-36.2742356128,4.17556147975619));
#58776=CARTESIAN_POINT('Ctrl Pts',(7.48466292267703,-36.2742356128,4.18615486043004));
#58777=CARTESIAN_POINT('Ctrl Pts',(7.52447163694981,-36.2742356128,4.19559140467563));
#58778=CARTESIAN_POINT('Ctrl Pts',(7.54665857513635,-36.2742356128,4.20085075624466));
#58779=CARTESIAN_POINT('Ctrl Pts',(7.56894070102147,-36.2742356128,4.20575111356474));
#58780=CARTESIAN_POINT('Ctrl Pts',(7.59131211993716,-36.2742356128,4.21028649976423));
#58781=CARTESIAN_POINT('Ctrl Pts',(7.64363395123072,-36.2742356128,4.22089377114362));
#58782=CARTESIAN_POINT('Ctrl Pts',(7.69642743540918,-36.2742356128,4.22949690219201));
#58783=CARTESIAN_POINT('Ctrl Pts',(7.74944318305338,-36.2742356128,4.2360142679208));
#58784=CARTESIAN_POINT('Ctrl Pts',(7.77661534855966,-36.2742356128,4.23935461391453));
#58785=CARTESIAN_POINT('Ctrl Pts',(7.80384358768627,-36.2742356128,4.24214768847752));
#58786=CARTESIAN_POINT('Ctrl Pts',(7.83109967842394,-36.2742356128,4.24438822334609));
#58787=CARTESIAN_POINT('Ctrl Pts',(7.88206506202742,-36.2742356128,4.24857773534005));
#58788=CARTESIAN_POINT('Ctrl Pts',(7.93314926842083,-36.2742356128,4.25083710134914));
#58789=CARTESIAN_POINT('Ctrl Pts',(7.98424169231689,-36.2742356128,4.25114613036265));
#58790=CARTESIAN_POINT('Ctrl Pts',(8.02711337374753,-36.2742356128,4.25140543678051));
#58791=CARTESIAN_POINT('Ctrl Pts',(8.06998494434458,-36.2742356128,4.25029122347823));
#58792=CARTESIAN_POINT('Ctrl Pts',(8.11277137057046,-36.2742356128,4.24780005442864));
#58793=CARTESIAN_POINT('Ctrl Pts',(8.17236599933709,-36.2742356128,4.24433025552743));
#58794=CARTESIAN_POINT('Ctrl Pts',(8.23180807055249,-36.2742356128,4.23818575219096));
#58795=CARTESIAN_POINT('Ctrl Pts',(8.29083353584622,-36.2742356128,4.22939425851744));
#58796=CARTESIAN_POINT('Ctrl Pts',(8.3177647922131,-36.2742356128,4.22538300729238));
#58797=CARTESIAN_POINT('Ctrl Pts',(8.34460932033512,-36.2742356128,4.22082141375137));
#58798=CARTESIAN_POINT('Ctrl Pts',(8.37134222810931,-36.2742356128,4.21571574014083));
#58799=CARTESIAN_POINT('Ctrl Pts',(8.43003512594198,-36.2742356128,4.20450608116464));
#58800=CARTESIAN_POINT('Ctrl Pts',(8.48821811216381,-36.2742356128,4.19066508416442));
#58801=CARTESIAN_POINT('Ctrl Pts',(8.54565009870481,-36.2742356128,4.17428481086938));
#58802=CARTESIAN_POINT('Ctrl Pts',(8.57686224125639,-36.2742356128,4.165382743295));
#58803=CARTESIAN_POINT('Ctrl Pts',(8.60785268188324,-36.2742356128,4.15573155832944));
#58804=CARTESIAN_POINT('Ctrl Pts',(8.63858384203004,-36.2742356128,4.14535244828011));
#58805=CARTESIAN_POINT('Ctrl Pts',(8.69362110899052,-36.2742356128,4.12676421900829));
#58806=CARTESIAN_POINT('Ctrl Pts',(8.74784697441915,-36.2742356128,4.10583276078715));
#58807=CARTESIAN_POINT('Ctrl Pts',(8.80112173381191,-36.2742356128,4.08265814640246));
#58808=CARTESIAN_POINT('Ctrl Pts',(8.83233010313792,-36.2742356128,4.06908245065182));
#58809=CARTESIAN_POINT('Ctrl Pts',(8.86321143979697,-36.2742356128,4.05473785563392));
#58810=CARTESIAN_POINT('Ctrl Pts',(8.89373446130519,-36.2742356128,4.03965203931799));
#58811=CARTESIAN_POINT('Ctrl Pts',(8.94582066834934,-36.2742356128,4.01390875070386));
#58812=CARTESIAN_POINT('Ctrl Pts',(8.99689375602961,-36.2742356128,3.9859890850355));
#58813=CARTESIAN_POINT('Ctrl Pts',(9.04679963513679,-36.2742356128,3.95605823396275));
#58814=CARTESIAN_POINT('Ctrl Pts',(9.09476983987168,-36.2742356128,3.92728829584052));
#58815=CARTESIAN_POINT('Ctrl Pts',(9.14166035956096,-36.2742356128,3.89666034325123));
#58816=CARTESIAN_POINT('Ctrl Pts',(9.1873503799917,-36.2742356128,3.86436442020436));
#58817=CARTESIAN_POINT('Ctrl Pts',(9.22551933413715,-36.2742356128,3.83738475168506));
#58818=CARTESIAN_POINT('Ctrl Pts',(9.26285040628098,-36.2742356128,3.80924177810094));
#58819=CARTESIAN_POINT('Ctrl Pts',(9.29929148141267,-36.2742356128,3.78006969542373));
#58820=CARTESIAN_POINT('Ctrl Pts',(9.31548964669419,-36.2742356128,3.76710261870868));
#58821=CARTESIAN_POINT('Ctrl Pts',(9.33151223703318,-36.2742356128,3.7539324919993));
#58822=CARTESIAN_POINT('Ctrl Pts',(9.34735616692466,-36.2742356128,3.74057247286867));
#58823=CARTESIAN_POINT('Ctrl Pts',(9.35985966791103,-36.2742356128,3.7300291914024));
#58824=CARTESIAN_POINT('Ctrl Pts',(9.37224859113989,-36.2742356128,3.71937049533655));
#58825=CARTESIAN_POINT('Ctrl Pts',(9.38452406192343,-36.2742356128,3.70860159408074));
#58826=CARTESIAN_POINT('Ctrl Pts',(9.39168770892528,-36.2742356128,3.70231714205812));
#58827=CARTESIAN_POINT('Ctrl Pts',(9.39881333926506,-36.2742356128,3.69599462972722));
#58828=CARTESIAN_POINT('Ctrl Pts',(9.40590237578182,-36.2742356128,3.68963402760814));
#58829=CARTESIAN_POINT('Ctrl Pts',(9.42297207364796,-36.2742356128,3.67431832763075));
#58830=CARTESIAN_POINT('Ctrl Pts',(9.43983678219286,-36.2742356128,3.65877516180039));
#58831=CARTESIAN_POINT('Ctrl Pts',(9.45650176318101,-36.2742356128,3.64301685700775));
#58832=CARTESIAN_POINT('Ctrl Pts',(9.48789581907781,-36.2742356128,3.6133308284518));
#58833=CARTESIAN_POINT('Ctrl Pts',(9.51857758677638,-36.2742356128,3.58287990661514));
#58834=CARTESIAN_POINT('Ctrl Pts',(9.54843599458563,-36.2742356128,3.55188465040527));
#58835=CARTESIAN_POINT('Ctrl Pts',(9.55027669304462,-36.2742356128,3.54997386799831));
#58836=CARTESIAN_POINT('Ctrl Pts',(9.55211427802768,-36.2742356128,3.54806102126526));
#58837=CARTESIAN_POINT('Ctrl Pts',(9.55394872954341,-36.2742356128,3.54614616349359));
#58838=CARTESIAN_POINT('Ctrl Pts',(9.57108594124286,-36.2742356128,3.5282578068234));
#58839=CARTESIAN_POINT('Ctrl Pts',(9.5879480776674,-36.2742356128,3.51019559573715));
#58840=CARTESIAN_POINT('Ctrl Pts',(9.60454635841574,-36.2742356128,3.49197510524274));
#58841=CARTESIAN_POINT('Ctrl Pts',(9.61854592084375,-36.2742356128,3.47660731516778));
#58842=CARTESIAN_POINT('Ctrl Pts',(9.63236114002549,-36.2742356128,3.46112352843253));
#58843=CARTESIAN_POINT('Ctrl Pts',(9.64601709274984,-36.2742356128,3.44551111050629));
#58844=CARTESIAN_POINT('Ctrl Pts',(9.68829875030944,-36.2742356128,3.39717183152965));
#58845=CARTESIAN_POINT('Ctrl Pts',(9.72900438532371,-36.2742356128,3.34764921013495));
#58846=CARTESIAN_POINT('Ctrl Pts',(9.76826941329833,-36.2742356128003,3.29726609260588));
#58847=CARTESIAN_POINT('Ctrl Pts',(9.81596491101616,-36.2742356128007,3.23606537555359));
#58848=CARTESIAN_POINT('Ctrl Pts',(9.86154147949212,-36.2742356128015,3.17359603058158));
#58849=CARTESIAN_POINT('Ctrl Pts',(9.90528177456204,-36.2742356128018,3.11040354515293));
#58850=CARTESIAN_POINT('Ctrl Pts',(9.93627439098575,-36.2742356128021,3.06562788786437));
#58851=CARTESIAN_POINT('Ctrl Pts',(9.96634647662424,-36.2742356128019,3.02048840177962));
#58852=CARTESIAN_POINT('Ctrl Pts',(9.99557085703759,-36.2742356128013,2.97516792500639));
#58853=CARTESIAN_POINT('Ctrl Pts',(10.0186995539105,-36.2742356128008,2.93930048985124));
#58854=CARTESIAN_POINT('Ctrl Pts',(10.0412970933275,-36.2742356128,2.90331950713817));
#58855=CARTESIAN_POINT('Ctrl Pts',(10.0633762714066,-36.2742356128,2.86731153433696));
#58856=CARTESIAN_POINT('Ctrl Pts',(10.0654960521548,-36.2742356128,2.86385447596031));
#58857=CARTESIAN_POINT('Ctrl Pts',(10.0676108788123,-36.2742356128,2.86039749820118));
#58858=CARTESIAN_POINT('Ctrl Pts',(10.0697211371,-36.2742356128,2.85693996784));
#58859=CARTESIAN_POINT('Ctrl Pts',(10.0697226446839,-36.2742356128,2.856937497759));
#58860=CARTESIAN_POINT('Ctrl Pts',(10.0868108449264,-36.2742356128,2.82893953241251));
#58861=CARTESIAN_POINT('Ctrl Pts',(10.1038408998495,-36.2742356128,2.80049888209122));
#58862=CARTESIAN_POINT('Ctrl Pts',(10.1206769338313,-36.2742356128,2.77172242081127));
#58863=CARTESIAN_POINT('Ctrl Pts',(10.1387077474632,-36.2742356128,2.74090382001234));
#58864=CARTESIAN_POINT('Ctrl Pts',(10.1565160503317,-36.2742356128,2.70970000356903));
#58865=CARTESIAN_POINT('Ctrl Pts',(10.1739861629327,-36.2742356128,2.67820448201693));
#58866=CARTESIAN_POINT('Ctrl Pts',(10.1914562755336,-36.2742356128,2.64670896046483));
#58867=CARTESIAN_POINT('Ctrl Pts',(10.2085888545462,-36.2742356128,2.61492121305597));
#58868=CARTESIAN_POINT('Ctrl Pts',(10.2253115688178,-36.2742356128,2.58290332614455));
#58869=CARTESIAN_POINT('Ctrl Pts',(10.2442752584305,-36.2742356128,2.54659479036591));
#58870=CARTESIAN_POINT('Ctrl Pts',(10.2627110130504,-36.2742356128,2.50999195948853));
#58871=CARTESIAN_POINT('Ctrl Pts',(10.2805666141344,-36.2742356128,2.47314559857214));
#58872=CARTESIAN_POINT('Ctrl Pts',(10.3020309699668,-36.2742356128,2.42885230381732));
#58873=CARTESIAN_POINT('Ctrl Pts',(10.3226574690849,-36.2742356128,2.38420646027191));
#58874=CARTESIAN_POINT('Ctrl Pts',(10.3424227968145,-36.2742356128,2.33925109872417));
#58875=CARTESIAN_POINT('Ctrl Pts',(10.3489984711218,-36.2742356128,2.32429501907034));
#58876=CARTESIAN_POINT('Ctrl Pts',(10.3554792490116,-36.2742356128,2.30930442405224));
#58877=CARTESIAN_POINT('Ctrl Pts',(10.361865220952,-36.2742356128,2.29428036879782));
#58878=CARTESIAN_POINT('Ctrl Pts',(10.3772600090511,-36.2742356128,2.25806158343659));
#58879=CARTESIAN_POINT('Ctrl Pts',(10.3921036880258,-36.2742356127998,2.22164740241346));
#58880=CARTESIAN_POINT('Ctrl Pts',(10.4064058460514,-36.2742356128045,2.18503336929683));
#58881=CARTESIAN_POINT('Ctrl Pts',(10.4113914515429,-36.2742356128061,2.17227004195534));
#58882=CARTESIAN_POINT('Ctrl Pts',(10.4163112030396,-36.2742356128083,2.15948291732981));
#58883=CARTESIAN_POINT('Ctrl Pts',(10.421165387575,-36.2742356128107,2.14667321556));
#58884=CARTESIAN_POINT('Ctrl Pts',(10.4378552303633,-36.2742356128188,2.10263040937052));
#58885=CARTESIAN_POINT('Ctrl Pts',(10.4537741614886,-36.2742356128187,2.05830255688421));
#58886=CARTESIAN_POINT('Ctrl Pts',(10.4689365032872,-36.2742356128129,2.0137770819743));
#58887=CARTESIAN_POINT('Ctrl Pts',(10.4708347607409,-36.2742356128122,2.00820269143803));
#58888=CARTESIAN_POINT('Ctrl Pts',(10.4727211655238,-36.2742356128114,2.00262526829492));
#58889=CARTESIAN_POINT('Ctrl Pts',(10.474595753097,-36.2742356128106,1.99704503209008));
#58890=CARTESIAN_POINT('Ctrl Pts',(10.4914316861822,-36.2742356128035,1.94692815054836));
#58891=CARTESIAN_POINT('Ctrl Pts',(10.5073119424348,-36.2742356128015,1.89658674680565));
#58892=CARTESIAN_POINT('Ctrl Pts',(10.5222742679554,-36.2742356128006,1.84619520383189));
#58893=CARTESIAN_POINT('Ctrl Pts',(10.5347506131046,-36.2742356127999,1.80417618199789));
#58894=CARTESIAN_POINT('Ctrl Pts',(10.5465886100346,-36.2742356128,1.7621246630014));
#58895=CARTESIAN_POINT('Ctrl Pts',(10.5578330012303,-36.2742356128,1.7201184927425));
#58896=CARTESIAN_POINT('Ctrl Pts',(10.5600735080027,-36.2742356128,1.71174853234975));
#58897=CARTESIAN_POINT('Ctrl Pts',(10.5622905328157,-36.2742356128,1.70338023330578));
#58898=CARTESIAN_POINT('Ctrl Pts',(10.5644845660067,-36.2742356128,1.69501397367632));
#58899=CARTESIAN_POINT('Ctrl Pts',(10.5723485254795,-36.2742356128,1.66502722282281));
#58900=CARTESIAN_POINT('Ctrl Pts',(10.5799204299038,-36.2742356128,1.63505503132499));
#58901=CARTESIAN_POINT('Ctrl Pts',(10.5872260308627,-36.2742356128,1.60511296430495));
#58902=CARTESIAN_POINT('Ctrl Pts',(10.5921494614707,-36.2742356128,1.58493424251863));
#58903=CARTESIAN_POINT('Ctrl Pts',(10.5969522070739,-36.2742356128,1.56476783804686));
#58904=CARTESIAN_POINT('Ctrl Pts',(10.6016441629848,-36.2742356128,1.54460836878356));
#58905=CARTESIAN_POINT('Ctrl Pts',(10.6120299146714,-36.2742356128,1.4999849226388));
#58906=CARTESIAN_POINT('Ctrl Pts',(10.6218649372005,-36.2742356128,1.45542433019419));
#58907=CARTESIAN_POINT('Ctrl Pts',(10.6312389216324,-36.2742356128,1.41097928305949));
#58908=CARTESIAN_POINT('Ctrl Pts',(10.6323836951226,-36.2742356128,1.40555154716935));
#58909=CARTESIAN_POINT('Ctrl Pts',(10.6335215933023,-36.2742356128,1.40012560768293));
#58910=CARTESIAN_POINT('Ctrl Pts',(10.6346527727281,-36.2742356128,1.39470165565607));
#58911=CARTESIAN_POINT('Ctrl Pts',(10.640718224484,-36.2742356128,1.36561810038896));
#58912=CARTESIAN_POINT('Ctrl Pts',(10.6465847391207,-36.2742356128,1.33662012121641));
#58913=CARTESIAN_POINT('Ctrl Pts',(10.6522905078878,-36.2742356128,1.30767149194298));
#58914=CARTESIAN_POINT('Ctrl Pts',(10.6573180094971,-36.2742356128,1.28216410000387));
#58915=CARTESIAN_POINT('Ctrl Pts',(10.6622206989433,-36.2742356128,1.25669466508444));
#58916=CARTESIAN_POINT('Ctrl Pts',(10.6670160317365,-36.2742356128,1.23127687061149));
#58917=CARTESIAN_POINT('Ctrl Pts',(10.6707148031908,-36.2742356128,1.21167142992987));
#58918=CARTESIAN_POINT('Ctrl Pts',(10.6743495673088,-36.2742356128,1.19209726647813));
#58919=CARTESIAN_POINT('Ctrl Pts',(10.6779240565849,-36.2742356128,1.17258170994967));
#58920=CARTESIAN_POINT('Ctrl Pts',(10.680203543542,-36.2742356128,1.16013644766692));
#58921=CARTESIAN_POINT('Ctrl Pts',(10.6824557997336,-36.2742356128,1.14772960431328));
#58922=CARTESIAN_POINT('Ctrl Pts',(10.6846973978384,-36.2742356128,1.13527354112906));
#58923=CARTESIAN_POINT('Ctrl Pts',(10.6868705679382,-36.2742356128,1.1231977171823));
#58924=CARTESIAN_POINT('Ctrl Pts',(10.6890335643841,-36.2742356128,1.11107657302086));
#58925=CARTESIAN_POINT('Ctrl Pts',(10.6911936071295,-36.2742356128,1.0988763009671));
#58926=CARTESIAN_POINT('Ctrl Pts',(10.6937914461701,-36.2742356128,1.08420328437349));
#58927=CARTESIAN_POINT('Ctrl Pts',(10.6963904005884,-36.2742356128,1.06938558364541));
#58928=CARTESIAN_POINT('Ctrl Pts',(10.6989919881183,-36.2742356128,1.05442681683859));
#58929=CARTESIAN_POINT('Ctrl Pts',(10.7019588055677,-36.2742356128,1.03736802874348));
#58930=CARTESIAN_POINT('Ctrl Pts',(10.7049289097575,-36.2742356128,1.02012674418216));
#58931=CARTESIAN_POINT('Ctrl Pts',(10.7078909939529,-36.2742356128,1.00278497532506));
#58932=CARTESIAN_POINT('Ctrl Pts',(10.7117733770868,-36.2742356128,0.980055239611377));
#58933=CARTESIAN_POINT('Ctrl Pts',(10.7156412504301,-36.2742356128,0.95715796020661));
#58934=CARTESIAN_POINT('Ctrl Pts',(10.7194527266718,-36.2742356128,0.934361636596206));
#58935=CARTESIAN_POINT('Ctrl Pts',(10.7221988944412,-36.2742356128,0.917936890595001));
#58936=CARTESIAN_POINT('Ctrl Pts',(10.7249152575914,-36.2742356128,0.901567378438556));
#58937=CARTESIAN_POINT('Ctrl Pts',(10.7275884500151,-36.2742356128,0.88533375000401));
#58938=CARTESIAN_POINT('Ctrl Pts',(10.7299953053386,-36.2742356128,0.870717520109329));
#58939=CARTESIAN_POINT('Ctrl Pts',(10.7323669962552,-36.2742356128,0.85621239808682));
#58940=CARTESIAN_POINT('Ctrl Pts',(10.734699590284,-36.2742356128,0.841838560557644));
#58941=CARTESIAN_POINT('Ctrl Pts',(10.7368184926509,-36.2742356128,0.828781527063753));
#58942=CARTESIAN_POINT('Ctrl Pts',(10.7389050773595,-36.2742356128,0.815833125356652));
#58943=CARTESIAN_POINT('Ctrl Pts',(10.7409628459172,-36.2742356128,0.802967107192119));
#58944=CARTESIAN_POINT('Ctrl Pts',(10.7427047093747,-36.2742356128,0.792076258073006));
#58945=CARTESIAN_POINT('Ctrl Pts',(10.7444259863495,-36.2742356128,0.781244030786989));
#58946=CARTESIAN_POINT('Ctrl Pts',(10.7461333960947,-36.2742356128,0.770425450444427));
#58947=CARTESIAN_POINT('Ctrl Pts',(10.746986856985,-36.2742356128,0.765017706206505));
#58948=CARTESIAN_POINT('Ctrl Pts',(10.7478357689667,-36.2742356128,0.759620335417667));
#58949=CARTESIAN_POINT('Ctrl Pts',(10.7486843238,-36.2742356128,0.754206356986));
#58950=CARTESIAN_POINT('',(9.7282927137,-36.2742356128,2.648549352));
#58951=CARTESIAN_POINT('',(10.3535102277,-36.2742356128,0.692259222377));
#58952=CARTESIAN_POINT('Ctrl Pts',(9.7282927137,-36.2742356128,2.648549352));
#58953=CARTESIAN_POINT('Ctrl Pts',(9.74639969517236,-36.2742356128,2.61888218325925));
#58954=CARTESIAN_POINT('Ctrl Pts',(9.76450481782315,-36.2742356127996,2.58857606374712));
#58955=CARTESIAN_POINT('Ctrl Pts',(9.78240917986035,-36.2742356128004,2.55776271394264));
#58956=CARTESIAN_POINT('Ctrl Pts',(9.80080208211504,-36.2742356128013,2.52610858798629));
#58957=CARTESIAN_POINT('Ctrl Pts',(9.81898317367036,-36.2742356127996,2.49391916838793));
#58958=CARTESIAN_POINT('Ctrl Pts',(9.83679025426058,-36.2742356128305,2.46132086015645));
#58959=CARTESIAN_POINT('Ctrl Pts',(9.84954651385432,-36.2742356128527,2.43796877388881));
#58960=CARTESIAN_POINT('Ctrl Pts',(9.86211199597106,-36.2742356128914,2.41440650413952));
#58961=CARTESIAN_POINT('Ctrl Pts',(9.87444269048559,-36.2742356129957,2.39067568122307));
#58962=CARTESIAN_POINT('Ctrl Pts',(9.89313929948119,-36.2742356131537,2.35469344869838));
#58963=CARTESIAN_POINT('Ctrl Pts',(9.91130525476423,-36.274235613575,2.31830080564483));
#58964=CARTESIAN_POINT('Ctrl Pts',(9.92886336081567,-36.2742356142595,2.28157258436356));
#58965=CARTESIAN_POINT('Ctrl Pts',(9.94780805475828,-36.2742356149981,2.24194388470814));
#58966=CARTESIAN_POINT('Ctrl Pts',(9.96604538607517,-36.2742356160186,2.20192435360085));
#58967=CARTESIAN_POINT('Ctrl Pts',(9.98353502301114,-36.274235616299,2.16158375789261));
#58968=CARTESIAN_POINT('Ctrl Pts',(9.99047178660671,-36.2742356164103,2.14558381594087));
#58969=CARTESIAN_POINT('Ctrl Pts',(9.99729149635977,-36.2742356163983,2.12953312949594));
#58970=CARTESIAN_POINT('Ctrl Pts',(10.0039936507053,-36.2742356162252,2.11343521377528));
#58971=CARTESIAN_POINT('Ctrl Pts',(10.0138233241821,-36.2742356159713,2.08982530462801));
#58972=CARTESIAN_POINT('Ctrl Pts',(10.0234041182003,-36.2742356155042,2.06610086022346));
#58973=CARTESIAN_POINT('Ctrl Pts',(10.0327214232002,-36.2742356149673,2.04231132471509));
#58974=CARTESIAN_POINT('Ctrl Pts',(10.0420387282002,-36.2742356144305,2.01852178920672));
#58975=CARTESIAN_POINT('Ctrl Pts',(10.0510920659195,-36.274235613744,1.99467139543396));
#58976=CARTESIAN_POINT('Ctrl Pts',(10.0598800359898,-36.2742356133125,1.97078707699407));
#58977=CARTESIAN_POINT('Ctrl Pts',(10.0774557575172,-36.2742356124497,1.9230190342708));
#58978=CARTESIAN_POINT('Ctrl Pts',(10.0939547323721,-36.2742356128,1.87511365332179));
#58979=CARTESIAN_POINT('Ctrl Pts',(10.1094721884702,-36.2742356128,1.82712935861783));
#58980=CARTESIAN_POINT('Ctrl Pts',(10.1249269578322,-36.2742356128,1.77933890875558));
#58981=CARTESIAN_POINT('Ctrl Pts',(10.1394203301501,-36.2742356128,1.73144552171482));
#58982=CARTESIAN_POINT('Ctrl Pts',(10.1530321403974,-36.2742356128,1.68352654520081));
#58983=CARTESIAN_POINT('Ctrl Pts',(10.1649940560187,-36.2742356128,1.64141585284596));
#58984=CARTESIAN_POINT('Ctrl Pts',(10.1762640081837,-36.2742356128,1.59931829911508));
#58985=CARTESIAN_POINT('Ctrl Pts',(10.186907836536,-36.2742356128,1.55738467788051));
#58986=CARTESIAN_POINT('Ctrl Pts',(10.1883759287505,-36.2742356128,1.55160081695896));
#58987=CARTESIAN_POINT('Ctrl Pts',(10.1898321493012,-36.2742356128,1.54582000429803));
#58988=CARTESIAN_POINT('Ctrl Pts',(10.1912767070894,-36.2742356128,1.540042567223));
#58989=CARTESIAN_POINT('Ctrl Pts',(10.2018224412741,-36.2742356128,1.4978654275073));
#58990=CARTESIAN_POINT('Ctrl Pts',(10.2117463179877,-36.2742356128,1.45586806131404));
#58991=CARTESIAN_POINT('Ctrl Pts',(10.2211403601895,-36.2742356128,1.41414635375179));
#58992=CARTESIAN_POINT('Ctrl Pts',(10.2304712937462,-36.2742356128,1.37270493026578));
#58993=CARTESIAN_POINT('Ctrl Pts',(10.239280159291,-36.2742356128,1.33153562152515));
#58994=CARTESIAN_POINT('Ctrl Pts',(10.2476672649487,-36.2742356128,1.29068235424995));
#58995=CARTESIAN_POINT('Ctrl Pts',(10.2559444639923,-36.2742356128,1.25036443784098));
#58996=CARTESIAN_POINT('Ctrl Pts',(10.2638115094769,-36.2742356128,1.21035441433096));
#58997=CARTESIAN_POINT('Ctrl Pts',(10.2713651096502,-36.2742356128,1.17064400636089));
#58998=CARTESIAN_POINT('Ctrl Pts',(10.2787081573781,-36.2742356128,1.13204050414655));
#58999=CARTESIAN_POINT('Ctrl Pts',(10.2857555068467,-36.2742356128,1.09372008741171));
#59000=CARTESIAN_POINT('Ctrl Pts',(10.2925879832386,-36.2742356128,1.05562716733571));
#59001=CARTESIAN_POINT('Ctrl Pts',(10.2993020847495,-36.2742356128,1.01819421951903));
#59002=CARTESIAN_POINT('Ctrl Pts',(10.305809150057,-36.2742356128,0.980980968471632));
#59003=CARTESIAN_POINT('Ctrl Pts',(10.312170914478,-36.2742356128,0.943887867072484));
#59004=CARTESIAN_POINT('Ctrl Pts',(10.3183609260776,-36.2742356128,0.907796193012892));
#59005=CARTESIAN_POINT('Ctrl Pts',(10.3244137257131,-36.2742356128,0.87181819850963));
#59006=CARTESIAN_POINT('Ctrl Pts',(10.3303660898792,-36.2742356128,0.835818017326376));
#59007=CARTESIAN_POINT('Ctrl Pts',(10.3363184540454,-36.2742356128,0.799817836143121));
#59008=CARTESIAN_POINT('Ctrl Pts',(10.3421708065341,-36.2742356128,0.763795596254962));
#59009=CARTESIAN_POINT('Ctrl Pts',(10.3479336927262,-36.2742356128,0.727569928829446));
#59010=CARTESIAN_POINT('Ctrl Pts',(10.3497066699331,-36.2742356128,0.716424943399226));
#59011=CARTESIAN_POINT('Ctrl Pts',(10.3514709231525,-36.2742356128,0.705260646778015));
#59012=CARTESIAN_POINT('Ctrl Pts',(10.3532261841132,-36.2742356128,0.694070745754275));
#59013=CARTESIAN_POINT('Ctrl Pts',(10.3533208886531,-36.2742356128,0.693466998247719));
#59014=CARTESIAN_POINT('Ctrl Pts',(10.3534155669269,-36.2742356128,0.692863176355315));
#59015=CARTESIAN_POINT('Ctrl Pts',(10.3535102277,-36.2742356128,0.692259222377));
#59016=CARTESIAN_POINT('',(6.27496287808,-36.2742356128,2.72284550202));
#59017=CARTESIAN_POINT('Ctrl Pts',(6.27496287808,-36.2742356128,2.72284550202));
#59018=CARTESIAN_POINT('Ctrl Pts',(6.3028237745312,-36.2742356128,2.77462456613411));
#59019=CARTESIAN_POINT('Ctrl Pts',(6.33266102473065,-36.2742356127999,2.82510898731958));
#59020=CARTESIAN_POINT('Ctrl Pts',(6.36432894986973,-36.2742356128001,2.87430077751781));
#59021=CARTESIAN_POINT('Ctrl Pts',(6.39573177399559,-36.2742356128004,2.92308076955223));
#59022=CARTESIAN_POINT('Ctrl Pts',(6.42893480005577,-36.2742356128,2.97058986708201));
#59023=CARTESIAN_POINT('Ctrl Pts',(6.46383563974238,-36.2742356128075,3.01679807520185));
#59024=CARTESIAN_POINT('Ctrl Pts',(6.49827611330993,-36.2742356128148,3.0623967652232));
#59025=CARTESIAN_POINT('Ctrl Pts',(6.53436997488869,-36.2742356128281,3.1067288077039));
#59026=CARTESIAN_POINT('Ctrl Pts',(6.57205669686505,-36.2742356128823,3.14973170076718));
#59027=CARTESIAN_POINT('Ctrl Pts',(6.58927927620085,-36.274235612907,3.16938373465635));
#59028=CARTESIAN_POINT('Ctrl Pts',(6.60683503228447,-36.2742356129409,3.18875770411654));
#59029=CARTESIAN_POINT('Ctrl Pts',(6.62472081865607,-36.2742356129908,3.20784512271744));
#59030=CARTESIAN_POINT('Ctrl Pts',(6.66420229257168,-36.274235613101,3.24997910575575));
#59031=CARTESIAN_POINT('Ctrl Pts',(6.70530692684205,-36.2742356131351,3.29074285237302));
#59032=CARTESIAN_POINT('Ctrl Pts',(6.74801769993325,-36.2742356130925,3.32999680629123));
#59033=CARTESIAN_POINT('Ctrl Pts',(6.79038833604411,-36.2742356130502,3.3689381523968));
#59034=CARTESIAN_POINT('Ctrl Pts',(6.83433964290682,-36.2742356129557,3.40639378325257));
#59035=CARTESIAN_POINT('Ctrl Pts',(6.87988888863763,-36.2742356128945,3.4421893332177));
#59036=CARTESIAN_POINT('Ctrl Pts',(6.92507555314669,-36.2742356128338,3.47769994335494));
#59037=CARTESIAN_POINT('Ctrl Pts',(6.97183486114045,-36.2742356128077,3.51157688320459));
#59038=CARTESIAN_POINT('Ctrl Pts',(7.02021674223042,-36.2742356128022,3.54361067505602));
#59039=CARTESIAN_POINT('Ctrl Pts',(7.04458018405629,-36.2742356127995,3.55974178460886));
#59040=CARTESIAN_POINT('Ctrl Pts',(7.06935559487873,-36.2742356128,3.57540488225698));
#59041=CARTESIAN_POINT('Ctrl Pts',(7.09455249876125,-36.2742356128,3.59056931505338));
#59042=CARTESIAN_POINT('Ctrl Pts',(7.13528363996614,-36.2742356128,3.61508282895183));
#59043=CARTESIAN_POINT('Ctrl Pts',(7.17711751931734,-36.2742356128,3.63829389976814));
#59044=CARTESIAN_POINT('Ctrl Pts',(7.22005071711028,-36.2742356128,3.6600252280536));
#59045=CARTESIAN_POINT('Ctrl Pts',(7.22426457543557,-36.2742356128,3.66215814018973));
#59046=CARTESIAN_POINT('Ctrl Pts',(7.22848898600892,-36.2742356128,3.66427678146597));
#59047=CARTESIAN_POINT('Ctrl Pts',(7.23272392142221,-36.2742356128,3.66638097422168));
#59048=CARTESIAN_POINT('Ctrl Pts',(7.27455512514582,-36.2742356128,3.68716545078337));
#59049=CARTESIAN_POINT('Ctrl Pts',(7.31741530957928,-36.2742356128,3.70653801486018));
#59050=CARTESIAN_POINT('Ctrl Pts',(7.36116658604512,-36.2742356128,3.72429188348139));
#59051=CARTESIAN_POINT('Ctrl Pts',(7.38747354611457,-36.2742356128,3.73496700774345));
#59052=CARTESIAN_POINT('Ctrl Pts',(7.41410383714687,-36.2742356128,3.74505817719987));
#59053=CARTESIAN_POINT('Ctrl Pts',(7.44102886118993,-36.2742356128,3.75452639334412));
#59054=CARTESIAN_POINT('Ctrl Pts',(7.47566119449322,-36.2742356128,3.76670489378932));
#59055=CARTESIAN_POINT('Ctrl Pts',(7.51077587512702,-36.2742356128,3.77785011506413));
#59056=CARTESIAN_POINT('Ctrl Pts',(7.54628534309336,-36.2742356128,3.78788183369851));
#59057=CARTESIAN_POINT('Ctrl Pts',(7.58124771398936,-36.2742356128,3.79775899288185));
#59058=CARTESIAN_POINT('Ctrl Pts',(7.61659277102232,-36.2742356128,3.8065576335011));
#59059=CARTESIAN_POINT('Ctrl Pts',(7.65227357737817,-36.2742356128,3.81421987407179));
#59060=CARTESIAN_POINT('Ctrl Pts',(7.68579079235983,-36.2742356128,3.82141749628604));
#59061=CARTESIAN_POINT('Ctrl Pts',(7.71960063055048,-36.2742356128,3.8276112329845));
#59062=CARTESIAN_POINT('Ctrl Pts',(7.7536458617549,-36.2742356128,3.83275416322896));
#59063=CARTESIAN_POINT('Ctrl Pts',(7.80194884419358,-36.2742356128,3.84005089350494));
#59064=CARTESIAN_POINT('Ctrl Pts',(7.85071830221758,-36.2742356128,3.84522820662984));
#59065=CARTESIAN_POINT('Ctrl Pts',(7.89972755275133,-36.2742356128,3.84817846111999));
#59066=CARTESIAN_POINT('Ctrl Pts',(7.94648093156463,-36.2742356128,3.85099291684563));
#59067=CARTESIAN_POINT('Ctrl Pts',(7.9934519414373,-36.2742356128,3.85178034557181));
#59068=CARTESIAN_POINT('Ctrl Pts',(8.04043402108122,-36.2742356128,3.8504930204742));
#59069=CARTESIAN_POINT('Ctrl Pts',(8.07113530574063,-36.2742356128,3.84965179474365));
#59070=CARTESIAN_POINT('Ctrl Pts',(8.10184114058114,-36.2742356128,3.84792554187736));
#59071=CARTESIAN_POINT('Ctrl Pts',(8.13249320763682,-36.2742356128,3.84531308289118));
#59072=CARTESIAN_POINT('Ctrl Pts',(8.17723382114091,-36.2742356128,3.84149986476192));
#59073=CARTESIAN_POINT('Ctrl Pts',(8.22185515513467,-36.2742356128046,3.83579376812364));
#59074=CARTESIAN_POINT('Ctrl Pts',(8.26614133198898,-36.2742356128544,3.82822139707751));
#59075=CARTESIAN_POINT('Ctrl Pts',(8.29571833031613,-36.2742356128876,3.82316410783576));
#59076=CARTESIAN_POINT('Ctrl Pts',(8.3251465213504,-36.2742356129346,3.81727535696549));
#59077=CARTESIAN_POINT('Ctrl Pts',(8.35436952870322,-36.2742356129424,3.81057315013535));
#59078=CARTESIAN_POINT('Ctrl Pts',(8.39085630599924,-36.2742356129521,3.80220502001613));
#59079=CARTESIAN_POINT('Ctrl Pts',(8.42702490644852,-36.2742356128792,3.79256699905163));
#59080=CARTESIAN_POINT('Ctrl Pts',(8.46274259986607,-36.274235612827,3.78172063018468));
#59081=CARTESIAN_POINT('Ctrl Pts',(8.49846029328184,-36.2742356127748,3.77087426131826));
#59082=CARTESIAN_POINT('Ctrl Pts',(8.53373640609619,-36.2742356128,3.75881047120901));
#59083=CARTESIAN_POINT('Ctrl Pts',(8.56844925695303,-36.2742356128,3.74561879250407));
#59084=CARTESIAN_POINT('Ctrl Pts',(8.61269289485571,-36.2742356128,3.72880519634176));
#59085=CARTESIAN_POINT('Ctrl Pts',(8.65603418238756,-36.2742356128,3.71015491345561));
#59086=CARTESIAN_POINT('Ctrl Pts',(8.69832444168997,-36.2742356128,3.6898583383386));
#59087=CARTESIAN_POINT('Ctrl Pts',(8.74129416914554,-36.2742356128,3.66923566268124));
#59088=CARTESIAN_POINT('Ctrl Pts',(8.78317866197519,-36.2742356128,3.64691408634317));
#59089=CARTESIAN_POINT('Ctrl Pts',(8.82386994827566,-36.2742356128,3.62311913239659));
#59090=CARTESIAN_POINT('Ctrl Pts',(8.86657743538069,-36.2742356128,3.59814516914229));
#59091=CARTESIAN_POINT('Ctrl Pts',(8.90796835167006,-36.2742356128,3.57155084765688));
#59092=CARTESIAN_POINT('Ctrl Pts',(8.94799791375628,-36.2742356128,3.54359600071795));
#59093=CARTESIAN_POINT('Ctrl Pts',(8.965002670958,-36.2742356128,3.53172064260677));
#59094=CARTESIAN_POINT('Ctrl Pts',(8.98176208440896,-36.2742356128,3.5196000334607));
#59095=CARTESIAN_POINT('Ctrl Pts',(8.99827512664272,-36.2742356128,3.50725452876548));
#59096=CARTESIAN_POINT('Ctrl Pts',(9.03434720067447,-36.2742356128,3.48028627221884));
#59097=CARTESIAN_POINT('Ctrl Pts',(9.06926218434382,-36.2742356128,3.45222818843661));
#59098=CARTESIAN_POINT('Ctrl Pts',(9.1030036175438,-36.2742356128,3.42331618990479));
#59099=CARTESIAN_POINT('Ctrl Pts',(9.10943887321986,-36.2742356128,3.41780201682401));
#59100=CARTESIAN_POINT('Ctrl Pts',(9.1158315930112,-36.2742356128,3.41225677682403));
#59101=CARTESIAN_POINT('Ctrl Pts',(9.12218187857283,-36.2742356128,3.40668208887777));
#59102=CARTESIAN_POINT('Ctrl Pts',(9.15591769209004,-36.2742356128,3.37706662810103));
#59103=CARTESIAN_POINT('Ctrl Pts',(9.18846346570522,-36.2742356126279,3.34660965236935));
#59104=CARTESIAN_POINT('Ctrl Pts',(9.21980647110474,-36.2742356130288,3.31558795797188));
#59105=CARTESIAN_POINT('Ctrl Pts',(9.22444834338276,-36.2742356130882,3.3109936715783));
#59106=CARTESIAN_POINT('Ctrl Pts',(9.22906391970104,-36.2742356131663,3.30638696037994));
#59107=CARTESIAN_POINT('Ctrl Pts',(9.2336532445861,-36.2742356132749,3.30176868004118));
#59108=CARTESIAN_POINT('Ctrl Pts',(9.25144261015871,-36.274235613696,3.28386707592281));
#59109=CARTESIAN_POINT('Ctrl Pts',(9.26883694920177,-36.2742356146205,3.26579252621011));
#59110=CARTESIAN_POINT('Ctrl Pts',(9.28584062583539,-36.2742356162734,3.24760004211036));
#59111=CARTESIAN_POINT('Ctrl Pts',(9.302844302469,-36.2742356179262,3.22940755801061));
#59112=CARTESIAN_POINT('Ctrl Pts',(9.31949202128959,-36.2742356204437,3.21105852851475));
#59113=CARTESIAN_POINT('Ctrl Pts',(9.33581316077557,-36.2742356244168,3.19257010082136));
#59114=CARTESIAN_POINT('Ctrl Pts',(9.36434739707762,-36.2742356313629,3.16024679612132));
#59115=CARTESIAN_POINT('Ctrl Pts',(9.39191683705234,-36.2742356357654,3.1274880628538));
#59116=CARTESIAN_POINT('Ctrl Pts',(9.41852620590725,-36.2742356356124,3.09454044363916));
#59117=CARTESIAN_POINT('Ctrl Pts',(9.44522459013014,-36.2742356354589,3.06148260593477));
#59118=CARTESIAN_POINT('Ctrl Pts',(9.47095736863029,-36.2742356315576,3.02823551422887));
#59119=CARTESIAN_POINT('Ctrl Pts',(9.49576670903768,-36.2742356276487,2.99501198544618));
#59120=CARTESIAN_POINT('Ctrl Pts',(9.50279286499792,-36.2742356265416,2.98560288020825));
#59121=CARTESIAN_POINT('Ctrl Pts',(9.50974513768581,-36.2742356254317,2.9761953997071));
#59122=CARTESIAN_POINT('Ctrl Pts',(9.51662486506729,-36.2742356243793,2.96679371865397));
#59123=CARTESIAN_POINT('Ctrl Pts',(9.52548491478471,-36.2742356230239,2.95468577353649));
#59124=CARTESIAN_POINT('Ctrl Pts',(9.53422639106844,-36.2742356219228,2.9425842244868));
#59125=CARTESIAN_POINT('Ctrl Pts',(9.54287330530364,-36.2742356208252,2.93046924908954));
#59126=CARTESIAN_POINT('Ctrl Pts',(9.56654480644426,-36.2742356178206,2.89730370053265));
#59127=CARTESIAN_POINT('Ctrl Pts',(9.58948819545112,-36.2742356158232,2.86405994531656));
#59128=CARTESIAN_POINT('Ctrl Pts',(9.61179276518404,-36.2742356146377,2.83081476039708));
#59129=CARTESIAN_POINT('Ctrl Pts',(9.63351607564837,-36.274235613483,2.79843594824792));
#59130=CARTESIAN_POINT('Ctrl Pts',(9.65463408372118,-36.2742356130699,2.76605589156097));
#59131=CARTESIAN_POINT('Ctrl Pts',(9.6752305983474,-36.2742356129102,2.73369667930163));
#59132=CARTESIAN_POINT('Ctrl Pts',(9.6928921026444,-36.2742356127732,2.70594866577907));
#59133=CARTESIAN_POINT('Ctrl Pts',(9.71017038222493,-36.2742356128,2.67821523964025));
#59134=CARTESIAN_POINT('Ctrl Pts',(9.72711381130454,-36.2742356128,2.65048002401181));
#59135=CARTESIAN_POINT('Ctrl Pts',(9.72750687873562,-36.2742356128,2.6498365999501));
#59136=CARTESIAN_POINT('Ctrl Pts',(9.72789975796667,-36.2742356128,2.64919318798333));
#59137=CARTESIAN_POINT('Ctrl Pts',(9.7282927137,-36.2742356128,2.648549352));
#59138=CARTESIAN_POINT('',(2.29653436395,-36.2742356128,-2.09683572989));
#59139=CARTESIAN_POINT('Ctrl Pts',(2.29653436395,-36.2742356128,-2.09683572989));
#59140=CARTESIAN_POINT('Ctrl Pts',(2.36844264581072,-36.2742356128,-2.06297361352936));
#59141=CARTESIAN_POINT('Ctrl Pts',(2.44020262706449,-36.2742356128,-2.02814938203184));
#59142=CARTESIAN_POINT('Ctrl Pts',(2.51175434855808,-36.2742356128,-1.99251485917145));
#59143=CARTESIAN_POINT('Ctrl Pts',(2.57619685221496,-36.2742356128,-1.96042090221547));
#59144=CARTESIAN_POINT('Ctrl Pts',(2.64046968487184,-36.2742356128,-1.9276691645241));
#59145=CARTESIAN_POINT('Ctrl Pts',(2.70449947469043,-36.2742356128,-1.89434968461788));
#59146=CARTESIAN_POINT('Ctrl Pts',(2.77206180084746,-36.2742356128,-1.85919196232666));
#59147=CARTESIAN_POINT('Ctrl Pts',(2.8393023230107,-36.2742356128,-1.82343113570922));
#59148=CARTESIAN_POINT('Ctrl Pts',(2.90642539048409,-36.2742356128,-1.78697407945998));
#59149=CARTESIAN_POINT('Ctrl Pts',(2.97354845795748,-36.2742356128,-1.75051702321074));
#59150=CARTESIAN_POINT('Ctrl Pts',(3.04052116237677,-36.2742356127993,-1.71337921672418));
#59151=CARTESIAN_POINT('Ctrl Pts',(3.10725339275564,-36.2742356128007,-1.67558113763683));
#59152=CARTESIAN_POINT('Ctrl Pts',(3.18601825695535,-36.2742356128024,-1.63096760457458));
#59153=CARTESIAN_POINT('Ctrl Pts',(3.2644395547577,-36.2742356128047,-1.58543858736672));
#59154=CARTESIAN_POINT('Ctrl Pts',(3.34237246387412,-36.2742356128046,-1.53896639731643));
#59155=CARTESIAN_POINT('Ctrl Pts',(3.42432560316084,-36.2742356128045,-1.49009690293556));
#59156=CARTESIAN_POINT('Ctrl Pts',(3.50573833803178,-36.2742356128027,-1.44018399272549));
#59157=CARTESIAN_POINT('Ctrl Pts',(3.58639477785833,-36.2742356128016,-1.3891592543171));
#59158=CARTESIAN_POINT('Ctrl Pts',(3.67575424130866,-36.2742356128003,-1.33262882405423));
#59159=CARTESIAN_POINT('Ctrl Pts',(3.76418511993075,-36.2742356128,-1.27473314069746));
#59160=CARTESIAN_POINT('Ctrl Pts',(3.85134110464983,-36.2742356128,-1.21534305390097));
#59161=CARTESIAN_POINT('Ctrl Pts',(3.86555391974856,-36.2742356128,-1.2056581157403));
#59162=CARTESIAN_POINT('Ctrl Pts',(3.87973273588502,-36.2742356128,-1.19593337885312));
#59163=CARTESIAN_POINT('Ctrl Pts',(3.89387594729535,-36.2742356128,-1.18616822317099));
#59164=CARTESIAN_POINT('Ctrl Pts',(4.00029785279444,-36.2742356128,-1.11268940389601));
#59165=CARTESIAN_POINT('Ctrl Pts',(4.10478398479914,-36.2742356128,-1.03687102559339));
#59166=CARTESIAN_POINT('Ctrl Pts',(4.20661656305114,-36.2742356128,-0.958414504056867));
#59167=CARTESIAN_POINT('Ctrl Pts',(4.30226608179997,-36.2742356128,-0.884721697133083));
#59168=CARTESIAN_POINT('Ctrl Pts',(4.39557138891166,-36.2742356128,-0.808698586640645));
#59169=CARTESIAN_POINT('Ctrl Pts',(4.48591276345593,-36.2742356128,-0.730108100871267));
#59170=CARTESIAN_POINT('Ctrl Pts',(4.52584144204364,-36.2742356128,-0.695373027797972));
#59171=CARTESIAN_POINT('Ctrl Pts',(4.56519106650209,-36.2742356128,-0.660136818345033));
#59172=CARTESIAN_POINT('Ctrl Pts',(4.60390869426853,-36.2742356128,-0.62438174071118));
#59173=CARTESIAN_POINT('Ctrl Pts',(4.6414702406575,-36.2742356128,-0.589694284772853));
#59174=CARTESIAN_POINT('Ctrl Pts',(4.67843073789759,-36.2742356128,-0.554524122905242));
#59175=CARTESIAN_POINT('Ctrl Pts',(4.71474137816731,-36.2742356128,-0.518860225151488));
#59176=CARTESIAN_POINT('Ctrl Pts',(4.78288652012131,-36.2742356128,-0.451928842035981));
#59177=CARTESIAN_POINT('Ctrl Pts',(4.84874492792749,-36.2742356128,-0.38325236142979));
#59178=CARTESIAN_POINT('Ctrl Pts',(4.91203343390612,-36.2742356128,-0.31276532051731));
#59179=CARTESIAN_POINT('Ctrl Pts',(4.97022521348273,-36.2742356128,-0.247954715742227));
#59180=CARTESIAN_POINT('Ctrl Pts',(5.02624407407463,-36.2742356128,-0.181613289617387));
#59181=CARTESIAN_POINT('Ctrl Pts',(5.07989426308131,-36.2742356128,-0.113725674955232));
#59182=CARTESIAN_POINT('Ctrl Pts',(5.12228748281073,-36.2742356128,-0.0600823492081344));
#59183=CARTESIAN_POINT('Ctrl Pts',(5.16320211219051,-36.2742356128,-0.00547418087444934));
#59184=CARTESIAN_POINT('Ctrl Pts',(5.20255537839219,-36.2742356128,0.050087718179765));
#59185=CARTESIAN_POINT('Ctrl Pts',(5.24837168523952,-36.2742356128,0.114774623786097));
#59186=CARTESIAN_POINT('Ctrl Pts',(5.29207438973777,-36.2742356128,0.180759277690909));
#59187=CARTESIAN_POINT('Ctrl Pts',(5.3336564943449,-36.2742356128,0.248044031897748));
#59188=CARTESIAN_POINT('Ctrl Pts',(5.37190124235283,-36.2742356128,0.309928549137294));
#59189=CARTESIAN_POINT('Ctrl Pts',(5.4083506840884,-36.2742356128,0.372912084581407));
#59190=CARTESIAN_POINT('Ctrl Pts',(5.44302947502448,-36.2742356128,0.436970376903849));
#59191=CARTESIAN_POINT('Ctrl Pts',(5.47645187793625,-36.2742356128,0.498707882683309));
#59192=CARTESIAN_POINT('Ctrl Pts',(5.50822844774793,-36.2742356128,0.561443272406974));
#59193=CARTESIAN_POINT('Ctrl Pts',(5.53842875337963,-36.2742356128,0.625137406042214));
#59194=CARTESIAN_POINT('Ctrl Pts',(5.56568797441512,-36.2742356128,0.682628627773582));
#59195=CARTESIAN_POINT('Ctrl Pts',(5.59166287037293,-36.2742356128,0.740900588750238));
#59196=CARTESIAN_POINT('Ctrl Pts',(5.61645139047291,-36.2742356128,0.799915459049706));
#59197=CARTESIAN_POINT('Ctrl Pts',(5.61912590323811,-36.2742356128,0.80628276227378));
#59198=CARTESIAN_POINT('Ctrl Pts',(5.62178665546896,-36.2742356128,0.812658706960601));
#59199=CARTESIAN_POINT('Ctrl Pts',(5.62443380765283,-36.2742356128,0.819043240976538));
#59200=CARTESIAN_POINT('Ctrl Pts',(5.63821488896908,-36.2742356128,0.852281142059808));
#59201=CARTESIAN_POINT('Ctrl Pts',(5.65162223151371,-36.2742356127983,0.885738848242016));
#59202=CARTESIAN_POINT('Ctrl Pts',(5.66468821373837,-36.2742356128112,0.919432993579274));
#59203=CARTESIAN_POINT('Ctrl Pts',(5.6830074126935,-36.2742356128293,0.966673969530669));
#59204=CARTESIAN_POINT('Ctrl Pts',(5.70065416799746,-36.27423561289,1.01437731418511));
#59205=CARTESIAN_POINT('Ctrl Pts',(5.71770208500406,-36.2742356129396,1.06248232003904));
#59206=CARTESIAN_POINT('Ctrl Pts',(5.73056789567574,-36.274235612977,1.09878645604799));
#59207=CARTESIAN_POINT('Ctrl Pts',(5.74309182301036,-36.2742356129966,1.13531530657873));
#59208=CARTESIAN_POINT('Ctrl Pts',(5.75531496840173,-36.2742356129631,1.17205239280299));
#59209=CARTESIAN_POINT('Ctrl Pts',(5.76290164272989,-36.2742356129423,1.19485440488948));
#59210=CARTESIAN_POINT('Ctrl Pts',(5.77037267378017,-36.2742356129007,1.21773704710012));
#59211=CARTESIAN_POINT('Ctrl Pts',(5.77774191173509,-36.2742356128602,1.24070637318723));
#59212=CARTESIAN_POINT('Ctrl Pts',(5.78763874363087,-36.2742356128057,1.27155400769627));
#59213=CARTESIAN_POINT('Ctrl Pts',(5.79735016193852,-36.2742356128004,1.30254774097663));
#59214=CARTESIAN_POINT('Ctrl Pts',(5.80690585556745,-36.2742356128,1.33367294521436));
#59215=CARTESIAN_POINT('Ctrl Pts',(5.80850125226195,-36.2742356128,1.3388695379354));
#59216=CARTESIAN_POINT('Ctrl Pts',(5.81009235283591,-36.2742356128,1.34406990458954));
#59217=CARTESIAN_POINT('Ctrl Pts',(5.81167935047957,-36.2742356128,1.34927411502766));
#59218=CARTESIAN_POINT('Ctrl Pts',(5.81722554825276,-36.2742356128,1.36746165327525));
#59219=CARTESIAN_POINT('Ctrl Pts',(5.8227208660317,-36.2742356128002,1.3856941788767));
#59220=CARTESIAN_POINT('Ctrl Pts',(5.82817327291951,-36.2742356128001,1.4039704504895));
#59221=CARTESIAN_POINT('Ctrl Pts',(5.83362567980732,-36.2742356127999,1.42224672210229));
#59222=CARTESIAN_POINT('Ctrl Pts',(5.83903086091247,-36.2742356128,1.44055010200303));
#59223=CARTESIAN_POINT('Ctrl Pts',(5.84436868428059,-36.2742356128,1.45878260789149));
#59224=CARTESIAN_POINT('Ctrl Pts',(5.85055639832583,-36.2742356128,1.47991810170344));
#59225=CARTESIAN_POINT('Ctrl Pts',(5.85665292951415,-36.2742356128,1.50095559806678));
#59226=CARTESIAN_POINT('Ctrl Pts',(5.86265812636259,-36.2742356128,1.52184723319947));
#59227=CARTESIAN_POINT('Ctrl Pts',(5.86821793006266,-36.2742356128,1.5411893785517));
#59228=CARTESIAN_POINT('Ctrl Pts',(5.873699232103,-36.2742356128,1.56040582099944));
#59229=CARTESIAN_POINT('Ctrl Pts',(5.87911331224062,-36.2742356128,1.57949901445499));
#59230=CARTESIAN_POINT('Ctrl Pts',(5.88408849546304,-36.2742356128,1.59704440228229));
#59231=CARTESIAN_POINT('Ctrl Pts',(5.88900683553615,-36.2742356128,1.61448547798691));
#59232=CARTESIAN_POINT('Ctrl Pts',(5.89388893987974,-36.2742356128,1.63186539882874));
#59233=CARTESIAN_POINT('Ctrl Pts',(5.89775638947452,-36.2742356128,1.64563322579158));
#59234=CARTESIAN_POINT('Ctrl Pts',(5.9016012789473,-36.2742356128,1.65936330446299));
#59235=CARTESIAN_POINT('Ctrl Pts',(5.90544038108676,-36.2742356128,1.67309959908521));
#59236=CARTESIAN_POINT('Ctrl Pts',(5.91404763889229,-36.2742356128,1.70389633874233));
#59237=CARTESIAN_POINT('Ctrl Pts',(5.92261916147267,-36.2742356128,1.73470121369864));
#59238=CARTESIAN_POINT('Ctrl Pts',(5.93129769863563,-36.2742356128,1.76582075309313));
#59239=CARTESIAN_POINT('Ctrl Pts',(5.93719226432172,-36.2742356128,1.78695751446628));
#59240=CARTESIAN_POINT('Ctrl Pts',(5.94313728997873,-36.2742356128,1.80824316276458));
#59241=CARTESIAN_POINT('Ctrl Pts',(5.94917528826636,-36.2742356128,1.82976108353145));
#59242=CARTESIAN_POINT('Ctrl Pts',(5.95444651401515,-36.2742356128,1.84854641810812));
#59243=CARTESIAN_POINT('Ctrl Pts',(5.9597888214508,-36.2742356128,1.86750955556035));
#59244=CARTESIAN_POINT('Ctrl Pts',(5.96522247846992,-36.2742356128,1.88667386362928));
#59245=CARTESIAN_POINT('Ctrl Pts',(5.97042798694682,-36.2742356128,1.90503350019741));
#59246=CARTESIAN_POINT('Ctrl Pts',(5.97571464628148,-36.2742356128,1.923568373342));
#59247=CARTESIAN_POINT('Ctrl Pts',(5.98109356255906,-36.2742356128,1.94227142362813));
#59248=CARTESIAN_POINT('Ctrl Pts',(5.98616571138456,-36.2742356128,1.95990781163764));
#59249=CARTESIAN_POINT('Ctrl Pts',(5.9913199976955,-36.2742356128,1.97769414502198));
#59250=CARTESIAN_POINT('Ctrl Pts',(5.99655425212487,-36.2742356128,1.99557925311492));
#59251=CARTESIAN_POINT('Ctrl Pts',(5.99687082384823,-36.2742356128,1.99666095817301));
#59252=CARTESIAN_POINT('Ctrl Pts',(5.99718768412742,-36.2742356128,1.99774300894027));
#59253=CARTESIAN_POINT('Ctrl Pts',(5.99750483090687,-36.2742356128,1.99882538789166));
#59254=CARTESIAN_POINT('Ctrl Pts',(6.00306576003192,-36.2742356128,2.01780408490275));
#59255=CARTESIAN_POINT('Ctrl Pts',(6.00871842800908,-36.2742356127999,2.03689599014484));
#59256=CARTESIAN_POINT('Ctrl Pts',(6.01445248808947,-36.2742356128001,2.0560106258512));
#59257=CARTESIAN_POINT('Ctrl Pts',(6.02403404969531,-36.2742356128006,2.08795100614474));
#59258=CARTESIAN_POINT('Ctrl Pts',(6.033867889391,-36.274235612802,2.12004423096413));
#59259=CARTESIAN_POINT('Ctrl Pts',(6.04400556249464,-36.2742356128029,2.15218869532583));
#59260=CARTESIAN_POINT('Ctrl Pts',(6.05513800463166,-36.274235612804,2.18748736651728));
#59261=CARTESIAN_POINT('Ctrl Pts',(6.06663691963859,-36.2742356128046,2.22284858676531));
#59262=CARTESIAN_POINT('Ctrl Pts',(6.07859889464087,-36.2742356128046,2.25819895240145));
#59263=CARTESIAN_POINT('Ctrl Pts',(6.09350733550585,-36.2742356128046,2.30225679699158));
#59264=CARTESIAN_POINT('Ctrl Pts',(6.10913487702226,-36.2742356128037,2.34629959452671));
#59265=CARTESIAN_POINT('Ctrl Pts',(6.12571299890265,-36.2742356128028,2.3902587946028));
#59266=CARTESIAN_POINT('Ctrl Pts',(6.14230562759224,-36.2742356128019,2.43425646150481));
#59267=CARTESIAN_POINT('Ctrl Pts',(6.15985227139991,-36.274235612801,2.47817620018358));
#59268=CARTESIAN_POINT('Ctrl Pts',(6.17860954326941,-36.2742356128006,2.52194911231665));
#59269=CARTESIAN_POINT('Ctrl Pts',(6.19307525815561,-36.2742356128002,2.55570703143523));
#59270=CARTESIAN_POINT('Ctrl Pts',(6.20826173241701,-36.2742356128001,2.58937838989207));
#59271=CARTESIAN_POINT('Ctrl Pts',(6.22428655479659,-36.2742356128,2.62289850029955));
#59272=CARTESIAN_POINT('Ctrl Pts',(6.23622615528486,-36.2742356128,2.64787329983915));
#59273=CARTESIAN_POINT('Ctrl Pts',(6.24863117121475,-36.2742356128,2.6727636320365));
#59274=CARTESIAN_POINT('Ctrl Pts',(6.26154754770469,-36.2742356128,2.69752366658337));
#59275=CARTESIAN_POINT('Ctrl Pts',(6.26508870643922,-36.2742356128,2.70431188715524));
#59276=CARTESIAN_POINT('Ctrl Pts',(6.26866844515828,-36.2742356128,2.71109052393618));
#59277=CARTESIAN_POINT('Ctrl Pts',(6.27228786163123,-36.2742356128,2.71785869834249));
#59278=CARTESIAN_POINT('Ctrl Pts',(6.27317711432132,-36.2742356128,2.71952156785276));
#59279=CARTESIAN_POINT('Ctrl Pts',(6.27406873921778,-36.2742356128,2.72118376295094));
#59280=CARTESIAN_POINT('Ctrl Pts',(6.27496287808,-36.2742356128,2.72284550202));
#59281=CARTESIAN_POINT('',(1.05996676265,-36.2742356128,-2.50526930112));
#59282=CARTESIAN_POINT('Origin',(0.442943622457021,-36.2742356127953,1.44025631334163));
#59283=CARTESIAN_POINT('',(0.417273426056,-36.2742356128,-3.28965091665));
#59284=CARTESIAN_POINT('Ctrl Pts',(0.417273426056,-36.2742356128,-3.28965091665));
#59285=CARTESIAN_POINT('Ctrl Pts',(0.417273426056,-36.2742356128,-3.24819118647009));
#59286=CARTESIAN_POINT('Ctrl Pts',(0.420519754893996,-36.2742356128,-3.20677004886387));
#59287=CARTESIAN_POINT('Ctrl Pts',(0.426943681519379,-36.2742356128,-3.16585830441977));
#59288=CARTESIAN_POINT('Ctrl Pts',(0.433369261721254,-36.2742356128,-3.12493602892469));
#59289=CARTESIAN_POINT('Ctrl Pts',(0.442974473167372,-36.2742356128,-3.08452446703945));
#59290=CARTESIAN_POINT('Ctrl Pts',(0.455636754962494,-36.2742356128,-3.0450968409));
#59291=CARTESIAN_POINT('Ctrl Pts',(0.467430703587185,-36.2742356128,-3.00837301776875));
#59292=CARTESIAN_POINT('Ctrl Pts',(0.481876462427866,-36.2742356128,-2.97250363953337));
#59293=CARTESIAN_POINT('Ctrl Pts',(0.498828968976865,-36.2742356128,-2.93785972150366));
#59294=CARTESIAN_POINT('Ctrl Pts',(0.515153014164737,-36.2742356128,-2.90450011879433));
#59295=CARTESIAN_POINT('Ctrl Pts',(0.53380145888552,-36.2742356128,-2.8722773944409));
#59296=CARTESIAN_POINT('Ctrl Pts',(0.554600533471897,-36.2742356128,-2.84150610599439));
#59297=CARTESIAN_POINT('Ctrl Pts',(0.574684449539934,-36.2742356128,-2.81179286217199));
#59298=CARTESIAN_POINT('Ctrl Pts',(0.596772989945446,-36.2742356128,-2.78343431295931));
#59299=CARTESIAN_POINT('Ctrl Pts',(0.620667862166697,-36.2742356128,-2.75668878505484));
#59300=CARTESIAN_POINT('Ctrl Pts',(0.629100264263006,-36.2742356128,-2.74725039829636));
#59301=CARTESIAN_POINT('Ctrl Pts',(0.637757237276887,-36.2742356128,-2.73801262565806));
#59302=CARTESIAN_POINT('Ctrl Pts',(0.646628795601126,-36.2742356128,-2.72898588795116));
#59303=CARTESIAN_POINT('Ctrl Pts',(0.673012364687384,-36.2742356128,-2.70214082317122));
#59304=CARTESIAN_POINT('Ctrl Pts',(0.701296621816972,-36.2742356127994,
-2.67716443387045));
#59305=CARTESIAN_POINT('Ctrl Pts',(0.731194309592696,-36.2742356128018,
-2.65430179476602));
#59306=CARTESIAN_POINT('Ctrl Pts',(0.742439371406182,-36.2742356128027,
-2.64570274216111));
#59307=CARTESIAN_POINT('Ctrl Pts',(0.753912541590767,-36.274235612804,-2.63740218614734));
#59308=CARTESIAN_POINT('Ctrl Pts',(0.765597959533844,-36.2742356128064,
-2.62941138371186));
#59309=CARTESIAN_POINT('Ctrl Pts',(0.797606714508346,-36.2742356128127,
-2.60752293791959));
#59310=CARTESIAN_POINT('Ctrl Pts',(0.83120590246872,-36.2742356128134,-2.58796315035183));
#59311=CARTESIAN_POINT('Ctrl Pts',(0.866047905424978,-36.2742356128085,
-2.5709319957786));
#59312=CARTESIAN_POINT('Ctrl Pts',(0.877736613138201,-36.2742356128068,
-2.56521842678329));
#59313=CARTESIAN_POINT('Ctrl Pts',(0.889564957491781,-36.2742356128049,
-2.55978907221658));
#59314=CARTESIAN_POINT('Ctrl Pts',(0.901519043131815,-36.2742356128032,
-2.55465043725105));
#59315=CARTESIAN_POINT('Ctrl Pts',(0.940012174823359,-36.274235612798,-2.53810361314431));
#59316=CARTESIAN_POINT('Ctrl Pts',(0.979809990161025,-36.2742356128,-2.52457520198315));
#59317=CARTESIAN_POINT('Ctrl Pts',(1.02045143135846,-36.2742356128,-2.51424729380737));
#59318=CARTESIAN_POINT('Ctrl Pts',(1.03008167823426,-36.2742356128,-2.51180003055801));
#59319=CARTESIAN_POINT('Ctrl Pts',(1.03975907726387,-36.2742356128,-2.50953240002355));
#59320=CARTESIAN_POINT('Ctrl Pts',(1.04947705709931,-36.2742356128,-2.50744672775021));
#59321=CARTESIAN_POINT('Ctrl Pts',(1.05296820937862,-36.2742356128,-2.50669745684882));
#59322=CARTESIAN_POINT('Ctrl Pts',(1.05646717145,-36.2742356128,-2.50597114875333));
#59323=CARTESIAN_POINT('Ctrl Pts',(1.05996676265,-36.2742356128,-2.50526930112));
#59324=CARTESIAN_POINT('',(0.417273580719025,-36.2742356128,-7.9503178894794));
#59325=CARTESIAN_POINT('',(0.417273426056,-36.2742356128,0.915007091638));
#59326=CARTESIAN_POINT('',(2.08574076971679,-36.2742356128,-9.317281773533));
#59327=CARTESIAN_POINT('Ctrl Pts',(2.08574076953038,-36.2742356128,-9.31728177257901));
#59328=CARTESIAN_POINT('Ctrl Pts',(2.03330044437365,-36.2742356128,-9.32752871414683));
#59329=CARTESIAN_POINT('Ctrl Pts',(1.98026066869069,-36.2742356128,-9.3347827687861));
#59330=CARTESIAN_POINT('Ctrl Pts',(1.92697417280592,-36.2742356128,-9.33898117872619));
#59331=CARTESIAN_POINT('Ctrl Pts',(1.87250923120824,-36.2742356128,-9.34327243767263));
#59332=CARTESIAN_POINT('Ctrl Pts',(1.81778687287914,-36.2742356128,-9.34437149963258));
#59333=CARTESIAN_POINT('Ctrl Pts',(1.76318602342788,-36.2742356128,-9.34226540624991));
#59334=CARTESIAN_POINT('Ctrl Pts',(1.75574898470314,-36.2742356128,-9.34197854078531));
#59335=CARTESIAN_POINT('Ctrl Pts',(1.74831419900645,-36.2742356128,-9.34163229076523));
#59336=CARTESIAN_POINT('Ctrl Pts',(1.74088262153701,-36.2742356128,-9.34122669715811));
#59337=CARTESIAN_POINT('Ctrl Pts',(1.68259407240854,-36.2742356128,-9.33804547984701));
#59338=CARTESIAN_POINT('Ctrl Pts',(1.62450457226369,-36.2742356128,-9.33120851843907));
#59339=CARTESIAN_POINT('Ctrl Pts',(1.56707106712167,-36.2742356128,-9.32077143204654));
#59340=CARTESIAN_POINT('Ctrl Pts',(1.51078881778076,-36.2742356128,-9.3105435572671));
#59341=CARTESIAN_POINT('Ctrl Pts',(1.45513695060325,-36.2742356128,-9.29685901434515));
#59342=CARTESIAN_POINT('Ctrl Pts',(1.40053396527419,-36.2742356128,-9.27982447959625));
#59343=CARTESIAN_POINT('Ctrl Pts',(1.3442556203685,-36.2742356128,-9.26226728164948));
#59344=CARTESIAN_POINT('Ctrl Pts',(1.28909210804698,-36.2742356128,-9.24115151949635));
#59345=CARTESIAN_POINT('Ctrl Pts',(1.23548138966384,-36.2742356128,-9.21664740185734));
#59346=CARTESIAN_POINT('Ctrl Pts',(1.1818706712807,-36.2742356128,-9.19214328421834));
#59347=CARTESIAN_POINT('Ctrl Pts',(1.12981326798746,-36.2742356128,-9.1642512489844));
#59348=CARTESIAN_POINT('Ctrl Pts',(1.07971883490905,-36.2742356128,-9.13318920782522));
#59349=CARTESIAN_POINT('Ctrl Pts',(1.02860460246243,-36.2742356128,-9.10149481995598));
#59350=CARTESIAN_POINT('Ctrl Pts',(0.979533727061269,-36.2742356127831,
-9.06649723223452));
#59351=CARTESIAN_POINT('Ctrl Pts',(0.932909924660566,-36.2742356128878,
-9.02849863344844));
#59352=CARTESIAN_POINT('Ctrl Pts',(0.887156901283107,-36.2742356129905,
-8.99120972329846));
#59353=CARTESIAN_POINT('Ctrl Pts',(0.843760705446356,-36.2742356132368,
-8.95103091589256));
#59354=CARTESIAN_POINT('Ctrl Pts',(0.803067537737909,-36.2742356136497,
-8.90828164242417));
#59355=CARTESIAN_POINT('Ctrl Pts',(0.763525064799684,-36.2742356140509,
-8.86674120493933));
#59356=CARTESIAN_POINT('Ctrl Pts',(0.726535097662597,-36.2742356146066,
-8.82277372740761));
#59357=CARTESIAN_POINT('Ctrl Pts',(0.692378156264808,-36.2742356150751,
-8.77670324089393));
#59358=CARTESIAN_POINT('Ctrl Pts',(0.658532619600355,-36.2742356155394,
-8.73105277347389));
#59359=CARTESIAN_POINT('Ctrl Pts',(0.627468960880158,-36.2742356158936,
-8.6833374757917));
#59360=CARTESIAN_POINT('Ctrl Pts',(0.599419561563431,-36.2742356158468,
-8.63390270394093));
#59361=CARTESIAN_POINT('Ctrl Pts',(0.570615857250581,-36.2742356157988,
-8.58313853123675));
#59362=CARTESIAN_POINT('Ctrl Pts',(0.544992286373528,-36.2742356148864,
-8.53056909660664));
#59363=CARTESIAN_POINT('Ctrl Pts',(0.522753564674736,-36.2742356141856,
-8.4765995297206));
#59364=CARTESIAN_POINT('Ctrl Pts',(0.502029446455075,-36.2742356135326,
-8.42630564594621));
#59365=CARTESIAN_POINT('Ctrl Pts',(0.484244625968573,-36.2742356131106,
-8.37479614579619));
#59366=CARTESIAN_POINT('Ctrl Pts',(0.469521955598608,-36.2742356129622,
-8.32242775617462));
#59367=CARTESIAN_POINT('Ctrl Pts',(0.468445962520008,-36.2742356129513,
-8.31860045967512));
#59368=CARTESIAN_POINT('Ctrl Pts',(0.467386305746146,-36.2742356129416,
-8.31476858813491));
#59369=CARTESIAN_POINT('Ctrl Pts',(0.466343023886594,-36.2742356129328,
-8.31093228675359));
#59370=CARTESIAN_POINT('Ctrl Pts',(0.450543397904615,-36.2742356128,-8.25283473006365));
#59371=CARTESIAN_POINT('Ctrl Pts',(0.438503293447399,-36.2742356128062,
-8.19372526762956));
#59372=CARTESIAN_POINT('Ctrl Pts',(0.430309059876441,-36.2742356128021,
-8.13408616006745));
#59373=CARTESIAN_POINT('Ctrl Pts',(0.422791149948173,-36.2742356127983,
-8.07936945777046));
#59374=CARTESIAN_POINT('Ctrl Pts',(0.41851018184678,-36.2742356128,-8.0242069294277));
#59375=CARTESIAN_POINT('Ctrl Pts',(0.417493303474974,-36.2742356128,-7.9690017292704));
#59376=CARTESIAN_POINT('Ctrl Pts',(0.417401823410547,-36.2742356128,-7.96403537792779));
#59377=CARTESIAN_POINT('Ctrl Pts',(0.417336732786752,-36.2742356128,-7.95906870352496));
#59378=CARTESIAN_POINT('Ctrl Pts',(0.417298034990758,-36.2742356128,-7.95410201315234));
#59379=CARTESIAN_POINT('Ctrl Pts',(0.417288206348154,-36.2742356128,-7.95284055049421));
#59380=CARTESIAN_POINT('Ctrl Pts',(0.417280080432586,-36.2742356128,-7.9515790775042));
#59381=CARTESIAN_POINT('Ctrl Pts',(0.417273658050834,-36.2742356128,-7.95031788947841));
#59382=CARTESIAN_POINT('',(2.11953888391737,-36.2742356128,-9.31090074964532));
#59383=CARTESIAN_POINT('Origin',(2.09997707267667,-36.2742356127977,-9.34384840219991));
#59384=CARTESIAN_POINT('Ctrl Pts',(10.3535102269266,-36.2742356128,0.692259222255781));
#59385=CARTESIAN_POINT('Ctrl Pts',(10.3562093920332,-36.2742356128,0.675037953476251));
#59386=CARTESIAN_POINT('Ctrl Pts',(10.3588778370901,-36.2742356128,0.657806411951718));
#59387=CARTESIAN_POINT('Ctrl Pts',(10.3615152739502,-36.2742356128,0.640566949063097));
#59388=CARTESIAN_POINT('Ctrl Pts',(10.3727685745492,-36.2742356128,0.56701036047497));
#59389=CARTESIAN_POINT('Ctrl Pts',(10.3834624844301,-36.2742356128,0.493289697396397));
#59390=CARTESIAN_POINT('Ctrl Pts',(10.3935931754126,-36.2742356128,0.419366129654924));
#59391=CARTESIAN_POINT('Ctrl Pts',(10.4061289190632,-36.2742356128,0.327892912621584));
#59392=CARTESIAN_POINT('Ctrl Pts',(10.4178057955057,-36.2742356127957,0.236089364064904));
#59393=CARTESIAN_POINT('Ctrl Pts',(10.428558083588,-36.2742356128043,0.143938604015692));
#59394=CARTESIAN_POINT('Ctrl Pts',(10.4400001246915,-36.2742356128135,0.0458764263548748));
#59395=CARTESIAN_POINT('Ctrl Pts',(10.4503948687392,-36.2742356127897,-0.0525792420430679));
#59396=CARTESIAN_POINT('Ctrl Pts',(10.4596079894754,-36.2742356131329,-0.151426466320893));
#59397=CARTESIAN_POINT('Ctrl Pts',(10.4695724147274,-36.2742356135041,-0.25833440836185));
#59398=CARTESIAN_POINT('Ctrl Pts',(10.4781541249895,-36.2742356141501,-0.365700880393748));
#59399=CARTESIAN_POINT('Ctrl Pts',(10.4851266846754,-36.2742356175533,-0.473491504220951));
#59400=CARTESIAN_POINT('Ctrl Pts',(10.4918461373707,-36.2742356208329,-0.577369280882969));
#59401=CARTESIAN_POINT('Ctrl Pts',(10.4970697073588,-36.2742356265035,-0.681640880070512));
#59402=CARTESIAN_POINT('Ctrl Pts',(10.5005608005868,-36.2742356409383,-0.786244887940372));
#59403=CARTESIAN_POINT('Ctrl Pts',(10.5045127180508,-36.2742356572785,-0.904656622749569));
#59404=CARTESIAN_POINT('Ctrl Pts',(10.5062623540639,-36.2742356782692,-1.02352896187271));
#59405=CARTESIAN_POINT('Ctrl Pts',(10.5054484661738,-36.2742356903982,-1.14275590241697));
#59406=CARTESIAN_POINT('Ctrl Pts',(10.5046492533298,-36.2742357023086,-1.2598330863741));
#59407=CARTESIAN_POINT('Ctrl Pts',(10.501376236877,-36.2742357042772,-1.37725221277007));
#59408=CARTESIAN_POINT('Ctrl Pts',(10.4952861980909,-36.2742356908098,-1.4948647931778));
#59409=CARTESIAN_POINT('Ctrl Pts',(10.4934120668053,-36.2742356866653,-1.53105855552529));
#59410=CARTESIAN_POINT('Ctrl Pts',(10.4912712575296,-36.2742356811994,-1.56727028837258));
#59411=CARTESIAN_POINT('Ctrl Pts',(10.4888541645596,-36.2742356747649,-1.60349471863259));
#59412=CARTESIAN_POINT('Ctrl Pts',(10.4818861663663,-36.2742356562156,-1.70792254484433));
#59413=CARTESIAN_POINT('Ctrl Pts',(10.4726172291219,-36.2742356337617,-1.81245827726364));
#59414=CARTESIAN_POINT('Ctrl Pts',(10.4608100921849,-36.2742356232957,-1.91693269295077));
#59415=CARTESIAN_POINT('Ctrl Pts',(10.4571364571787,-36.2742356200393,-1.94943853012084));
#59416=CARTESIAN_POINT('Ctrl Pts',(10.4532173571464,-36.2742356177031,-1.98193815780485));
#59417=CARTESIAN_POINT('Ctrl Pts',(10.449046400631,-36.274235616125,-2.01442572802847));
#59418=CARTESIAN_POINT('Ctrl Pts',(10.4365783728994,-36.2742356114077,-2.11153916591473));
#59419=CARTESIAN_POINT('Ctrl Pts',(10.421841819238,-36.2742356128118,-2.20856774744078));
#59420=CARTESIAN_POINT('Ctrl Pts',(10.4047260362417,-36.274235612802,-2.3053166118921));
#59421=CARTESIAN_POINT('Ctrl Pts',(10.397713265999,-36.274235612798,-2.34495707460304));
#59422=CARTESIAN_POINT('Ctrl Pts',(10.3903015981004,-36.2742356128,-2.38455030881704));
#59423=CARTESIAN_POINT('Ctrl Pts',(10.3824857480538,-36.2742356128,-2.42408179319258));
#59424=CARTESIAN_POINT('Ctrl Pts',(10.3633959928289,-36.2742356128,-2.52063512467945));
#59425=CARTESIAN_POINT('Ctrl Pts',(10.3418892837525,-36.2742356128,-2.61683237280929));
#59426=CARTESIAN_POINT('Ctrl Pts',(10.3179031203684,-36.2742356128,-2.71246883714195));
#59427=CARTESIAN_POINT('Ctrl Pts',(10.2957385119174,-36.2742356128,-2.80084248621773));
#59428=CARTESIAN_POINT('Ctrl Pts',(10.271456816493,-36.2742356128,-2.88873703944073));
#59429=CARTESIAN_POINT('Ctrl Pts',(10.2450543902945,-36.2742356128,-2.97597002930809));
#59430=CARTESIAN_POINT('Ctrl Pts',(10.2428845586102,-36.2742356128,-2.98313910172208));
#59431=CARTESIAN_POINT('Ctrl Pts',(10.2407004304474,-36.2742356128,-2.99030369449288));
#59432=CARTESIAN_POINT('Ctrl Pts',(10.2385020185913,-36.2742356128,-2.99746370019166));
#59433=CARTESIAN_POINT('Ctrl Pts',(10.2115899242788,-36.2742356128,-3.08511367720213));
#59434=CARTESIAN_POINT('Ctrl Pts',(10.1825218137777,-36.2742356128,-3.17211436346743));
#59435=CARTESIAN_POINT('Ctrl Pts',(10.1513609907264,-36.2742356128,-3.25830680597497));
#59436=CARTESIAN_POINT('Ctrl Pts',(10.1191814800406,-36.2742356128,-3.34731699098008));
#59437=CARTESIAN_POINT('Ctrl Pts',(10.0847703883543,-36.2742356128,-3.43546527477735));
#59438=CARTESIAN_POINT('Ctrl Pts',(10.0482313430007,-36.2742356128,-3.52262013151324));
#59439=CARTESIAN_POINT('Ctrl Pts',(10.0440330941911,-36.2742356128,-3.53263401583891));
#59440=CARTESIAN_POINT('Ctrl Pts',(10.0398067869187,-36.2742356128,-3.5426348306343));
#59441=CARTESIAN_POINT('Ctrl Pts',(10.0355526038407,-36.2742356128,-3.55262241101358));
#59442=CARTESIAN_POINT('Ctrl Pts',(9.99574377590588,-36.2742356128,-3.64608192169306));
#59443=CARTESIAN_POINT('Ctrl Pts',(9.95348996234073,-36.2742356127974,-3.7383821453158));
#59444=CARTESIAN_POINT('Ctrl Pts',(9.90894409633191,-36.274235612804,-3.82944201792403));
#59445=CARTESIAN_POINT('Ctrl Pts',(9.86082512674903,-36.2742356128112,-3.9278059657568));
#59446=CARTESIAN_POINT('Ctrl Pts',(9.81003197512694,-36.274235612815,-4.02472257560848));
#59447=CARTESIAN_POINT('Ctrl Pts',(9.75678784892353,-36.2742356129677,-4.12014431547425));
#59448=CARTESIAN_POINT('Ctrl Pts',(9.70038315635778,-36.2742356131295,-4.22123028091305));
#59449=CARTESIAN_POINT('Ctrl Pts',(9.64122859138951,-36.2742356134239,-4.32063899789456));
#59450=CARTESIAN_POINT('Ctrl Pts',(9.57961405954658,-36.2742356145569,-4.418370168869));
#59451=CARTESIAN_POINT('Ctrl Pts',(9.51096163102881,-36.2742356158192,-4.52726464600931));
#59452=CARTESIAN_POINT('Ctrl Pts',(9.43925643293375,-36.2742356180243,-4.63407677905874));
#59453=CARTESIAN_POINT('Ctrl Pts',(9.36491343540478,-36.2742356238331,-4.73886931201533));
#59454=CARTESIAN_POINT('Ctrl Pts',(9.34738694186789,-36.2742356252025,-4.76357433754059));
#59455=CARTESIAN_POINT('Ctrl Pts',(9.32971384400554,-36.2742356267831,-4.78816734894402));
#59456=CARTESIAN_POINT('Ctrl Pts',(9.31189953928727,-36.2742356286321,-4.81264955991275));
#59457=CARTESIAN_POINT('Ctrl Pts',(9.23439860673501,-36.2742356366765,-4.91915914370095));
#59458=CARTESIAN_POINT('Ctrl Pts',(9.15429593033449,-36.2742356347254,-5.02353989346411));
#59459=CARTESIAN_POINT('Ctrl Pts',(9.07199160966919,-36.2742356291196,-5.12593022601556));
#59460=CARTESIAN_POINT('Ctrl Pts',(8.99453182595689,-36.2742356238438,-5.2222937334178));
#59461=CARTESIAN_POINT('Ctrl Pts',(8.91512306183019,-36.2742356177619,-5.31689571089193));
#59462=CARTESIAN_POINT('Ctrl Pts',(8.83405735451404,-36.2742356153905,-5.40985684740955));
#59463=CARTESIAN_POINT('Ctrl Pts',(8.82923042275601,-36.2742356152493,-5.41539207404207));
#59464=CARTESIAN_POINT('Ctrl Pts',(8.82439760074115,-36.2742356151174,-5.42092148120503));
#59465=CARTESIAN_POINT('Ctrl Pts',(8.81955894387271,-36.2742356149942,-5.42644509335966));
#59466=CARTESIAN_POINT('Ctrl Pts',(8.74513530805297,-36.2742356131003,-5.51140406246664));
#59467=CARTESIAN_POINT('Ctrl Pts',(8.66932164913453,-36.2742356129864,-5.59500897384072));
#59468=CARTESIAN_POINT('Ctrl Pts',(8.59233223129399,-36.274235612874,-5.67732225807105));
#59469=CARTESIAN_POINT('Ctrl Pts',(8.52142141683534,-36.2742356127705,-5.75313659969431));
#59470=CARTESIAN_POINT('Ctrl Pts',(8.44951333249385,-36.2742356128003,-5.82785570799169));
#59471=CARTESIAN_POINT('Ctrl Pts',(8.37673301404561,-36.2742356128001,-5.90151430451527));
#59472=CARTESIAN_POINT('Ctrl Pts',(8.34543794122704,-36.2742356127999,-5.93318703130553));
#59473=CARTESIAN_POINT('Ctrl Pts',(8.31398102395895,-36.2742356128,-5.96466344924576));
#59474=CARTESIAN_POINT('Ctrl Pts',(8.28236940694129,-36.2742356128,-5.99594511180429));
#59475=CARTESIAN_POINT('Ctrl Pts',(8.20001179535807,-36.2742356128,-6.07744309443625));
#59476=CARTESIAN_POINT('Ctrl Pts',(8.11660321287264,-36.2742356128,-6.15762467605));
#59477=CARTESIAN_POINT('Ctrl Pts',(8.0323151898841,-36.2742356128,-6.23653007960427));
#59478=CARTESIAN_POINT('Ctrl Pts',(7.94850474427214,-36.2742356128,-6.31498840379551));
#59479=CARTESIAN_POINT('Ctrl Pts',(7.86382513325578,-36.2742356128,-6.39218413842518));
#59480=CARTESIAN_POINT('Ctrl Pts',(7.77839945421262,-36.2742356128,-6.46813409547328));
#59481=CARTESIAN_POINT('Ctrl Pts',(7.69733765843861,-36.2742356128,-6.54020422679956));
#59482=CARTESIAN_POINT('Ctrl Pts',(7.61560400991131,-36.2742356128,-6.6111518590271));
#59483=CARTESIAN_POINT('Ctrl Pts',(7.53326120006503,-36.2742356128,-6.68098237572902));
#59484=CARTESIAN_POINT('Ctrl Pts',(7.44973420875221,-36.2742356128,-6.75181713316343));
#59485=CARTESIAN_POINT('Ctrl Pts',(7.36558032122966,-36.2742356128,-6.8215019053945));
#59486=CARTESIAN_POINT('Ctrl Pts',(7.28083955628857,-36.2742356128,-6.89002539244422));
#59487=CARTESIAN_POINT('Ctrl Pts',(7.23551914769524,-36.2742356128,-6.92667260035523));
#59488=CARTESIAN_POINT('Ctrl Pts',(7.1900300427837,-36.2742356128,-6.96298776645332));
#59489=CARTESIAN_POINT('Ctrl Pts',(7.14437232377622,-36.2742356128,-6.99897053618122));
#59490=CARTESIAN_POINT('Ctrl Pts',(7.06326365371102,-36.2742356128,-7.06289213939169));
#59491=CARTESIAN_POINT('Ctrl Pts',(6.98159496509443,-36.2742356128,-7.12578783863602));
#59492=CARTESIAN_POINT('Ctrl Pts',(6.89932083587377,-36.2742356128,-7.18767259991881));
#59493=CARTESIAN_POINT('Ctrl Pts',(6.84868300071105,-36.2742356128,-7.22576124784017));
#59494=CARTESIAN_POINT('Ctrl Pts',(6.79781491836607,-36.2742356128,-7.26346724760522));
#59495=CARTESIAN_POINT('Ctrl Pts',(6.74669690171385,-36.2742356128,-7.30079801871496));
#59496=CARTESIAN_POINT('Ctrl Pts',(6.63653183176793,-36.2742356128,-7.38125002526323));
#59497=CARTESIAN_POINT('Ctrl Pts',(6.52520299962451,-36.2742356128,-7.45996077864774));
#59498=CARTESIAN_POINT('Ctrl Pts',(6.41266159909594,-36.2742356128,-7.53683581128796));
#59499=CARTESIAN_POINT('Ctrl Pts',(6.29028365174599,-36.2742356128,-7.62043001442375));
#59500=CARTESIAN_POINT('Ctrl Pts',(6.16647232408381,-36.2742356128,-7.70185249404446));
#59501=CARTESIAN_POINT('Ctrl Pts',(6.04121534251757,-36.2742356128,-7.78095113049375));
#59502=CARTESIAN_POINT('Ctrl Pts',(5.89675184985328,-36.2742356128,-7.87217850276126));
#59503=CARTESIAN_POINT('Ctrl Pts',(5.75036379756427,-36.2742356128,-7.9603131905575));
#59504=CARTESIAN_POINT('Ctrl Pts',(5.60211169574243,-36.2742356128,-8.04509917799797));
#59505=CARTESIAN_POINT('Ctrl Pts',(5.4664708448076,-36.2742356128,-8.12267273913099));
#59506=CARTESIAN_POINT('Ctrl Pts',(5.3292712661405,-36.2742356128,-8.19744131634106));
#59507=CARTESIAN_POINT('Ctrl Pts',(5.19057678671885,-36.2742356128,-8.26924053097918));
#59508=CARTESIAN_POINT('Ctrl Pts',(5.14691539854509,-36.2742356128,-8.29184311324459));
#59509=CARTESIAN_POINT('Ctrl Pts',(5.10310589926147,-36.2742356128,-8.31415178850976));
#59510=CARTESIAN_POINT('Ctrl Pts',(5.05915024981415,-36.2742356128,-8.33616259114357));
#59511=CARTESIAN_POINT('Ctrl Pts',(4.9149063727951,-36.2742356128,-8.40839274922615));
#59512=CARTESIAN_POINT('Ctrl Pts',(4.76907703785031,-36.2742356128,-8.4774166113732));
#59513=CARTESIAN_POINT('Ctrl Pts',(4.62172660701796,-36.2742356128,-8.54311658750294));
#59514=CARTESIAN_POINT('Ctrl Pts',(4.47177917813589,-36.2742356128,-8.6099745019496));
#59515=CARTESIAN_POINT('Ctrl Pts',(4.32025603921681,-36.2742356128001,-8.67339068051086));
#59516=CARTESIAN_POINT('Ctrl Pts',(4.16724319798237,-36.2742356128002,-8.73329245421995));
#59517=CARTESIAN_POINT('Ctrl Pts',(4.00592103591442,-36.2742356128003,-8.79644717750001));
#59518=CARTESIAN_POINT('Ctrl Pts',(3.84294213456988,-36.2742356128004,-8.855695593392));
#59519=CARTESIAN_POINT('Ctrl Pts',(3.67843820111028,-36.2742356128005,-8.91100547987655));
#59520=CARTESIAN_POINT('Ctrl Pts',(3.52009056743237,-36.2742356128007,-8.96424548125302));
#59521=CARTESIAN_POINT('Ctrl Pts',(3.36032959080013,-36.2742356128008,-9.01383705874524));
#59522=CARTESIAN_POINT('Ctrl Pts',(3.19930855420316,-36.2742356128008,-9.05979054692544));
#59523=CARTESIAN_POINT('Ctrl Pts',(3.03944143838186,-36.2742356128008,-9.10541471984443));
#59524=CARTESIAN_POINT('Ctrl Pts',(2.87833180211124,-36.2742356128008,-9.14745333097509));
#59525=CARTESIAN_POINT('Ctrl Pts',(2.71617158796638,-36.2742356128006,-9.18594575578493));
#59526=CARTESIAN_POINT('Ctrl Pts',(2.5569407515265,-36.2742356128005,-9.2237428259935));
#59527=CARTESIAN_POINT('Ctrl Pts',(2.39669662428977,-36.2742356128002,-9.2581212331758));
#59528=CARTESIAN_POINT('Ctrl Pts',(2.23566714738507,-36.2742356128001,-9.28913817160275));
#59529=CARTESIAN_POINT('Ctrl Pts',(2.21107200779576,-36.2742356128001,-9.29387560194722));
#59530=CARTESIAN_POINT('Ctrl Pts',(2.18645864179448,-36.2742356128,-9.29853464335292));
#59531=CARTESIAN_POINT('Ctrl Pts',(2.16182796614964,-36.2742356128,-9.30311552892602));
#59532=CARTESIAN_POINT('Ctrl Pts',(2.14773674018185,-36.2742356128,-9.30573625661834));
#59533=CARTESIAN_POINT('Ctrl Pts',(2.13364445853742,-36.2742356128,-9.30833065550249));
#59534=CARTESIAN_POINT('Ctrl Pts',(2.11954062634,-36.2742356128,-9.3109005156));
#59535=CARTESIAN_POINT('',(-2.08574139433879,-36.2742356128,-9.31728165005513));
#59536=CARTESIAN_POINT('',(-2.11953809613257,-36.2742356128,-9.31090088400518));
#59537=CARTESIAN_POINT('Origin',(-2.11596805996584,-36.2742356128,-9.34083853594215));
#59538=CARTESIAN_POINT('',(-0.417295449791195,-36.2742356130695,-7.95031783857217));
#59539=CARTESIAN_POINT('Ctrl Pts',(-0.417317472604425,-36.2742356128,-7.95031777923111));
#59540=CARTESIAN_POINT('Ctrl Pts',(-0.417546231264646,-36.2742356128,-7.98699548713484));
#59541=CARTESIAN_POINT('Ctrl Pts',(-0.419189898479267,-36.2742356128,-8.02382064895258));
#59542=CARTESIAN_POINT('Ctrl Pts',(-0.422268169047606,-36.2742356128,-8.06057389439151));
#59543=CARTESIAN_POINT('Ctrl Pts',(-0.425579935577801,-36.2742356128,-8.10011498261571));
#59544=CARTESIAN_POINT('Ctrl Pts',(-0.430552260190847,-36.2742356128,-8.13957291541615));
#59545=CARTESIAN_POINT('Ctrl Pts',(-0.437183115066485,-36.2742356128,-8.17873091302802));
#59546=CARTESIAN_POINT('Ctrl Pts',(-0.444221005381981,-36.2742356128,-8.22029262676411));
#59547=CARTESIAN_POINT('Ctrl Pts',(-0.453127236965292,-36.2742356128,-8.26151691063071));
#59548=CARTESIAN_POINT('Ctrl Pts',(-0.463870525352078,-36.2742356128,-8.30220140912958));
#59549=CARTESIAN_POINT('Ctrl Pts',(-0.475525438127585,-36.2742356128,-8.34633820079412));
#59550=CARTESIAN_POINT('Ctrl Pts',(-0.489342347521156,-36.2742356128,-8.38984042100709));
#59551=CARTESIAN_POINT('Ctrl Pts',(-0.50524902702277,-36.2742356128,-8.43250571146025));
#59552=CARTESIAN_POINT('Ctrl Pts',(-0.523707995997356,-36.2742356128,-8.48201681606801));
#59553=CARTESIAN_POINT('Ctrl Pts',(-0.544981258452666,-36.2742356128,-8.53040226246549));
#59554=CARTESIAN_POINT('Ctrl Pts',(-0.568913005101385,-36.2742356128,-8.57740254193819));
#59555=CARTESIAN_POINT('Ctrl Pts',(-0.597130208862658,-36.2742356128,-8.63281915996381));
#59556=CARTESIAN_POINT('Ctrl Pts',(-0.629042639893959,-36.2742356128,-8.68631556893906));
#59557=CARTESIAN_POINT('Ctrl Pts',(-0.664342184627549,-36.2742356128,-8.73748510336353));
#59558=CARTESIAN_POINT('Ctrl Pts',(-0.691469202170332,-36.2742356128,-8.77680790110681));
#59559=CARTESIAN_POINT('Ctrl Pts',(-0.720595035674572,-36.2742356128,-8.81475797815996));
#59560=CARTESIAN_POINT('Ctrl Pts',(-0.751569999107162,-36.2742356128,-8.8511190844982));
#59561=CARTESIAN_POINT('Ctrl Pts',(-0.766075428722424,-36.2742356128,-8.86814681949038));
#59562=CARTESIAN_POINT('Ctrl Pts',(-0.780986324397503,-36.2742356128,-8.88482547557127));
#59563=CARTESIAN_POINT('Ctrl Pts',(-0.796287350366606,-36.2742356128,-8.90112867589867));
#59564=CARTESIAN_POINT('Ctrl Pts',(-0.841225815081245,-36.2742356128,-8.94901048422498));
#59565=CARTESIAN_POINT('Ctrl Pts',(-0.889533606854501,-36.2742356128,-8.99364989843403));
#59566=CARTESIAN_POINT('Ctrl Pts',(-0.940722367446665,-36.2742356128,-9.03468164511675));
#59567=CARTESIAN_POINT('Ctrl Pts',(-0.990589460005256,-36.2742356128,-9.07465397275269));
#59568=CARTESIAN_POINT('Ctrl Pts',(-1.04319010310048,-36.2742356128,-9.11120153033691));
#59569=CARTESIAN_POINT('Ctrl Pts',(-1.09803239553826,-36.2742356128,-9.14401237848499));
#59570=CARTESIAN_POINT('Ctrl Pts',(-1.15083837102938,-36.2742356128,-9.17560494630327));
#59571=CARTESIAN_POINT('Ctrl Pts',(-1.20572210860661,-36.2742356128,-9.20373244016034));
#59572=CARTESIAN_POINT('Ctrl Pts',(-1.26221438398181,-36.2742356128,-9.22815264079006));
#59573=CARTESIAN_POINT('Ctrl Pts',(-1.31652092227226,-36.2742356128,-9.2516280018328));
#59574=CARTESIAN_POINT('Ctrl Pts',(-1.37231353359154,-36.2742356128,-9.27167690323985));
#59575=CARTESIAN_POINT('Ctrl Pts',(-1.42915351048309,-36.2742356128,-9.28812676549147));
#59576=CARTESIAN_POINT('Ctrl Pts',(-1.48289927719425,-36.2742356128,-9.30368114301511));
#59577=CARTESIAN_POINT('Ctrl Pts',(-1.53758114708514,-36.2742356128,-9.31601746172819));
#59578=CARTESIAN_POINT('Ctrl Pts',(-1.59281351672207,-36.2742356128,-9.32503325122765));
#59579=CARTESIAN_POINT('Ctrl Pts',(-1.64655555550598,-36.2742356128,-9.33380576836086));
#59580=CARTESIAN_POINT('Ctrl Pts',(-1.70081857799357,-36.2742356128,-9.33943422361108));
#59581=CARTESIAN_POINT('Ctrl Pts',(-1.75523679570936,-36.2742356128,-9.3418704259924));
#59582=CARTESIAN_POINT('Ctrl Pts',(-1.81052478073578,-36.2742356128,-9.34434556623831));
#59583=CARTESIAN_POINT('Ctrl Pts',(-1.86597282268321,-36.2742356128,-9.3435249016013));
#59584=CARTESIAN_POINT('Ctrl Pts',(-1.92118875397118,-36.2742356128,-9.33941424583912));
#59585=CARTESIAN_POINT('Ctrl Pts',(-1.97252446862824,-36.2742356128,-9.33559246023598));
#59586=CARTESIAN_POINT('Ctrl Pts',(-2.02365935968099,-36.2742356128,-9.32892702411511));
#59587=CARTESIAN_POINT('Ctrl Pts',(-2.07427344695003,-36.2742356128,-9.31947306843533));
#59588=CARTESIAN_POINT('Ctrl Pts',(-2.07809911928149,-36.2742356128,-9.31875848997272));
#59589=CARTESIAN_POINT('Ctrl Pts',(-2.08192181451298,-36.2742356128,-9.31802800517262));
#59590=CARTESIAN_POINT('Ctrl Pts',(-2.08574139369,-36.2742356128,-9.31728165018));
#59591=CARTESIAN_POINT('',(-0.417273456068905,-36.2742356128057,-3.28965270484013));
#59592=CARTESIAN_POINT('',(-0.417273426056,-36.2742356128,0.915007091638));
#59593=CARTESIAN_POINT('',(-1.05996478409,-36.2742356128,-2.50526963826));
#59594=CARTESIAN_POINT('Ctrl Pts',(-1.05996478409,-36.2742356128,-2.50526963826));
#59595=CARTESIAN_POINT('Ctrl Pts',(-1.01931967505232,-36.2742356128,-2.51342106522695));
#59596=CARTESIAN_POINT('Ctrl Pts',(-0.9793504971128,-36.2742356128,-2.52474706012613));
#59597=CARTESIAN_POINT('Ctrl Pts',(-0.940505223089573,-36.2742356128,-2.53908773691866));
#59598=CARTESIAN_POINT('Ctrl Pts',(-0.902843959426671,-36.2742356128,-2.55299130751685));
#59599=CARTESIAN_POINT('Ctrl Pts',(-0.86624009095651,-36.2742356128,-2.56972849573662));
#59600=CARTESIAN_POINT('Ctrl Pts',(-0.831094331796187,-36.2742356128,-2.58910597838381));
#59601=CARTESIAN_POINT('Ctrl Pts',(-0.811886969644185,-36.2742356128,-2.59969588555015));
#59602=CARTESIAN_POINT('Ctrl Pts',(-0.793114883117866,-36.2742356128,-2.61107353370296));
#59603=CARTESIAN_POINT('Ctrl Pts',(-0.774840964085916,-36.2742356128,-2.62320119611295));
#59604=CARTESIAN_POINT('Ctrl Pts',(-0.743411052499667,-36.2742356128,-2.64405995972176));
#59605=CARTESIAN_POINT('Ctrl Pts',(-0.713455797872463,-36.2742356128,-2.66714014311122));
#59606=CARTESIAN_POINT('Ctrl Pts',(-0.685276497880166,-36.2742356128,-2.69221820140988));
#59607=CARTESIAN_POINT('Ctrl Pts',(-0.658305885066703,-36.2742356128,-2.71622059326032));
#59608=CARTESIAN_POINT('Ctrl Pts',(-0.632962377549237,-36.2742356128,-2.74205330272653));
#59609=CARTESIAN_POINT('Ctrl Pts',(-0.609482897196851,-36.2742356128,-2.76948226806354));
#59610=CARTESIAN_POINT('Ctrl Pts',(-0.590134228562073,-36.2742356128,-2.79208557756339));
#59611=CARTESIAN_POINT('Ctrl Pts',(-0.57205081595477,-36.2742356128,-2.81577241456369));
#59612=CARTESIAN_POINT('Ctrl Pts',(-0.555345443066818,-36.2742356128,-2.8403938476929));
#59613=CARTESIAN_POINT('Ctrl Pts',(-0.534212430985569,-36.2742356128,-2.87154101497058));
#59614=CARTESIAN_POINT('Ctrl Pts',(-0.515285354405834,-36.2742356127994,
-2.90418431450337));
#59615=CARTESIAN_POINT('Ctrl Pts',(-0.498748018357097,-36.2742356128018,
-2.9379939067206));
#59616=CARTESIAN_POINT('Ctrl Pts',(-0.492528026848015,-36.2742356128027,
-2.9507103065021));
#59617=CARTESIAN_POINT('Ctrl Pts',(-0.486645558484015,-36.274235612804,
-2.96359166617615));
#59618=CARTESIAN_POINT('Ctrl Pts',(-0.481108531718049,-36.2742356128064,
-2.97662022125917));
#59619=CARTESIAN_POINT('Ctrl Pts',(-0.465941480447615,-36.2742356128127,
-3.01230810417467));
#59620=CARTESIAN_POINT('Ctrl Pts',(-0.453370359796223,-36.2742356128134,
-3.04909747252491));
#59621=CARTESIAN_POINT('Ctrl Pts',(-0.44352288631122,-36.2742356128085,
-3.08660817285071));
#59622=CARTESIAN_POINT('Ctrl Pts',(-0.440219280518529,-36.2742356128068,
-3.0991921688445));
#59623=CARTESIAN_POINT('Ctrl Pts',(-0.437221797877176,-36.2742356128049,
-3.11185718865161));
#59624=CARTESIAN_POINT('Ctrl Pts',(-0.434534084237162,-36.2742356128032,
-3.12458832905277));
#59625=CARTESIAN_POINT('Ctrl Pts',(-0.425879427376572,-36.274235612798,
-3.16558363821654));
#59626=CARTESIAN_POINT('Ctrl Pts',(-0.420440800887583,-36.2742356128,-3.20726463195048));
#59627=CARTESIAN_POINT('Ctrl Pts',(-0.418306079453427,-36.2742356128,-3.24914344852297));
#59628=CARTESIAN_POINT('Ctrl Pts',(-0.417800243602732,-36.2742356128,-3.25906690104849));
#59629=CARTESIAN_POINT('Ctrl Pts',(-0.417479805275784,-36.2742356128,-3.26900126298853));
#59630=CARTESIAN_POINT('Ctrl Pts',(-0.41734575245625,-36.2742356128,-3.2789396340017));
#59631=CARTESIAN_POINT('Ctrl Pts',(-0.417297594428668,-36.2742356128,-3.28250996058665));
#59632=CARTESIAN_POINT('Ctrl Pts',(-0.41727348657,-36.2742356128,-3.28608342917333));
#59633=CARTESIAN_POINT('Ctrl Pts',(-0.41727348535,-36.2742356128,-3.28965270484));
#59634=CARTESIAN_POINT('',(-2.29653265536,-36.2742356128,-2.09683653367));
#59635=CARTESIAN_POINT('Origin',(-0.442148072512747,-36.2742356127947,1.43999152964127));
#59636=CARTESIAN_POINT('',(-6.27496294130418,-36.2742356128,2.72284562885154));
#59637=CARTESIAN_POINT('Ctrl Pts',(-6.2749628032,-36.2742356128,2.72284536858));
#59638=CARTESIAN_POINT('Ctrl Pts',(-6.24453537274772,-36.2742356128,2.66629639399008));
#59639=CARTESIAN_POINT('Ctrl Pts',(-6.2168833111465,-36.2742356128,2.6090079890714));
#59640=CARTESIAN_POINT('Ctrl Pts',(-6.19141504098666,-36.2742356128,2.551348392481));
#59641=CARTESIAN_POINT('Ctrl Pts',(-6.17072302935005,-36.2742356128,2.50450213884372));
#59642=CARTESIAN_POINT('Ctrl Pts',(-6.1514737587113,-36.2742356128,2.45741434061633));
#59643=CARTESIAN_POINT('Ctrl Pts',(-6.1333727111274,-36.2742356128,2.41026966734787));
#59644=CARTESIAN_POINT('Ctrl Pts',(-6.11724305155994,-36.2742356128,2.36825952806092));
#59645=CARTESIAN_POINT('Ctrl Pts',(-6.10202552397655,-36.2742356128,2.32620538526914));
#59646=CARTESIAN_POINT('Ctrl Pts',(-6.08752271510141,-36.2742356128,2.28420045422166));
#59647=CARTESIAN_POINT('Ctrl Pts',(-6.07444612368462,-36.2742356128,2.24632632062948));
#59648=CARTESIAN_POINT('Ctrl Pts',(-6.06195079512164,-36.2742356128,2.208492564208));
#59649=CARTESIAN_POINT('Ctrl Pts',(-6.04989771094152,-36.2742356128,2.17072599038824));
#59650=CARTESIAN_POINT('Ctrl Pts',(-6.04164302161129,-36.2742356128,2.14486113046605));
#59651=CARTESIAN_POINT('Ctrl Pts',(-6.03359587134105,-36.2742356128,2.11902695315767));
#59652=CARTESIAN_POINT('Ctrl Pts',(-6.0257127381864,-36.2742356128,2.09321776497177));
#59653=CARTESIAN_POINT('Ctrl Pts',(-6.01988428400105,-36.2742356128,2.07413554627123));
#59654=CARTESIAN_POINT('Ctrl Pts',(-6.01414698874104,-36.2742356127997,
2.05507173915977));
#59655=CARTESIAN_POINT('Ctrl Pts',(-6.00849032434624,-36.2742356128003,
2.03604835176757));
#59656=CARTESIAN_POINT('Ctrl Pts',(-6.00026038362399,-36.274235612801,2.00837102469864));
#59657=CARTESIAN_POINT('Ctrl Pts',(-5.9922193766253,-36.2742356128019,1.98084599545624));
#59658=CARTESIAN_POINT('Ctrl Pts',(-5.98436613823573,-36.2742356128016,
1.95363294374715));
#59659=CARTESIAN_POINT('Ctrl Pts',(-5.97824034356331,-36.2742356128013,
1.93240583221554));
#59660=CARTESIAN_POINT('Ctrl Pts',(-5.97222942790735,-36.2742356128007,
1.91137021894081));
#59661=CARTESIAN_POINT('Ctrl Pts',(-5.9663261063212,-36.2742356128004,1.8905682486979));
#59662=CARTESIAN_POINT('Ctrl Pts',(-5.96115895320338,-36.2742356128001,
1.8723603696541));
#59663=CARTESIAN_POINT('Ctrl Pts',(-5.95607439962134,-36.2742356128,1.85433193430266));
#59664=CARTESIAN_POINT('Ctrl Pts',(-5.95105754275361,-36.2742356128,1.83647095674252));
#59665=CARTESIAN_POINT('Ctrl Pts',(-5.94895269411707,-36.2742356128,1.82897728983993));
#59666=CARTESIAN_POINT('Ctrl Pts',(-5.9468596177166,-36.2742356128,1.82151253845821));
#59667=CARTESIAN_POINT('Ctrl Pts',(-5.94477649645998,-36.2742356128,1.81407306760198));
#59668=CARTESIAN_POINT('Ctrl Pts',(-5.93757006918152,-36.2742356128,1.78833668497644));
#59669=CARTESIAN_POINT('Ctrl Pts',(-5.93048994125108,-36.2742356128,1.76293068499097));
#59670=CARTESIAN_POINT('Ctrl Pts',(-5.92345520647712,-36.2742356128,1.73768612585181));
#59671=CARTESIAN_POINT('Ctrl Pts',(-5.91531260482293,-36.2742356128,1.70846592130808));
#59672=CARTESIAN_POINT('Ctrl Pts',(-5.90722899374801,-36.2742356128,1.6794554850506));
#59673=CARTESIAN_POINT('Ctrl Pts',(-5.89907507031516,-36.2742356128,1.65035466102641));
#59674=CARTESIAN_POINT('Ctrl Pts',(-5.89290045814991,-36.2742356128,1.62831787057597));
#59675=CARTESIAN_POINT('Ctrl Pts',(-5.886685159316,-36.2742356128,1.6062273279421));
#59676=CARTESIAN_POINT('Ctrl Pts',(-5.88038345128574,-36.2742356128,1.5839833454214));
#59677=CARTESIAN_POINT('Ctrl Pts',(-5.87491371948055,-36.2742356128,1.56467610076913));
#59678=CARTESIAN_POINT('Ctrl Pts',(-5.86937880076088,-36.2742356128,1.54525279633991));
#59679=CARTESIAN_POINT('Ctrl Pts',(-5.86376008203665,-36.2742356128,1.52568667108676));
#59680=CARTESIAN_POINT('Ctrl Pts',(-5.86063563574475,-36.2742356128,1.51480637782159));
#59681=CARTESIAN_POINT('Ctrl Pts',(-5.85748549226303,-36.2742356128,1.50388266814331));
#59682=CARTESIAN_POINT('Ctrl Pts',(-5.85430841249731,-36.2742356128,1.4929178587057));
#59683=CARTESIAN_POINT('Ctrl Pts',(-5.84903277585167,-36.2742356128,1.47471046237093));
#59684=CARTESIAN_POINT('Ctrl Pts',(-5.84368586733359,-36.2742356128,1.45639984537539));
#59685=CARTESIAN_POINT('Ctrl Pts',(-5.83827687493929,-36.2742356128,1.438048312437));
#59686=CARTESIAN_POINT('Ctrl Pts',(-5.83316400341666,-36.2742356128,1.42070145311135));
#59687=CARTESIAN_POINT('Ctrl Pts',(-5.82799788376965,-36.2742356128,1.40332542183888));
#59688=CARTESIAN_POINT('Ctrl Pts',(-5.82279354468847,-36.2742356128,1.38599962836736));
#59689=CARTESIAN_POINT('Ctrl Pts',(-5.82249212631315,-36.2742356128,1.38499617481874));
#59690=CARTESIAN_POINT('Ctrl Pts',(-5.8221905835966,-36.2742356128,1.38399290398093));
#59691=CARTESIAN_POINT('Ctrl Pts',(-5.82188892091261,-36.2742356128,1.38298983663647));
#59692=CARTESIAN_POINT('Ctrl Pts',(-5.81355730601708,-36.2742356128,1.35528614217218));
#59693=CARTESIAN_POINT('Ctrl Pts',(-5.80513063484038,-36.2742356128,1.32772641991473));
#59694=CARTESIAN_POINT('Ctrl Pts',(-5.79657009907114,-36.2742356128,1.30026398785058));
#59695=CARTESIAN_POINT('Ctrl Pts',(-5.78691018700546,-36.2742356128,1.26927472666409));
#59696=CARTESIAN_POINT('Ctrl Pts',(-5.77708000240597,-36.2742356128,1.23841018151499));
#59697=CARTESIAN_POINT('Ctrl Pts',(-5.76704602152116,-36.2742356128,1.20766721886827));
#59698=CARTESIAN_POINT('Ctrl Pts',(-5.7529866774042,-36.2742356128,1.16459100654669));
#59699=CARTESIAN_POINT('Ctrl Pts',(-5.73852780525219,-36.2742356128,1.12175735602248));
#59700=CARTESIAN_POINT('Ctrl Pts',(-5.72361628682829,-36.2742356128,1.0792503575753));
#59701=CARTESIAN_POINT('Ctrl Pts',(-5.71260137263102,-36.2742356128,1.04785107767843));
#59702=CARTESIAN_POINT('Ctrl Pts',(-5.7013407996525,-36.2742356128,1.01663358324319));
#59703=CARTESIAN_POINT('Ctrl Pts',(-5.68981205327961,-36.2742356128,0.985611834769589));
#59704=CARTESIAN_POINT('Ctrl Pts',(-5.68573367726689,-36.2742356128,0.974637670644965));
#59705=CARTESIAN_POINT('Ctrl Pts',(-5.68162165873323,-36.2742356128,0.963687599243863));
#59706=CARTESIAN_POINT('Ctrl Pts',(-5.67747462183944,-36.2742356128,0.952760543386742));
#59707=CARTESIAN_POINT('Ctrl Pts',(-5.65389160120622,-36.2742356128,0.890621481126485));
#59708=CARTESIAN_POINT('Ctrl Pts',(-5.62917129836967,-36.2742356128,0.829225266724225));
#59709=CARTESIAN_POINT('Ctrl Pts',(-5.60316923875744,-36.2742356128,0.768629253667028));
#59710=CARTESIAN_POINT('Ctrl Pts',(-5.57625830207163,-36.2742356128,0.705915165048141));
#59711=CARTESIAN_POINT('Ctrl Pts',(-5.54797443819125,-36.2742356128,0.644058001660994));
#59712=CARTESIAN_POINT('Ctrl Pts',(-5.51820998035682,-36.2742356128,0.583101326837146));
#59713=CARTESIAN_POINT('Ctrl Pts',(-5.48778020704284,-36.2742356128,0.520782106806925));
#59714=CARTESIAN_POINT('Ctrl Pts',(-5.45580305455407,-36.2742356128,0.459403793931162));
#59715=CARTESIAN_POINT('Ctrl Pts',(-5.42221613166309,-36.2742356128,0.398996157173145));
#59716=CARTESIAN_POINT('Ctrl Pts',(-5.38743512568233,-36.2742356128,0.336440906661415));
#59717=CARTESIAN_POINT('Ctrl Pts',(-5.35092793674563,-36.2742356128,0.274926244750017));
#59718=CARTESIAN_POINT('Ctrl Pts',(-5.3126795256956,-36.2742356128,0.214472196036214));
#59719=CARTESIAN_POINT('Ctrl Pts',(-5.30231556565285,-36.2742356128,0.198091297376847));
#59720=CARTESIAN_POINT('Ctrl Pts',(-5.2918240555852,-36.2742356128,0.181788215678701));
#59721=CARTESIAN_POINT('Ctrl Pts',(-5.28120533345534,-36.2742356128,0.165563244497791));
#59722=CARTESIAN_POINT('Ctrl Pts',(-5.23908934623629,-36.2742356128,0.101211746216937));
#59723=CARTESIAN_POINT('Ctrl Pts',(-5.19496806917432,-36.2742356128,0.0380905722805007));
#59724=CARTESIAN_POINT('Ctrl Pts',(-5.14890045052453,-36.2742356128,-0.0237928430699731));
#59725=CARTESIAN_POINT('Ctrl Pts',(-5.10113638619278,-36.2742356128,-0.0879551227471305));
#59726=CARTESIAN_POINT('Ctrl Pts',(-5.05128029700902,-36.2742356128,-0.150787036013723));
#59727=CARTESIAN_POINT('Ctrl Pts',(-4.99945322518508,-36.2742356128,-0.212299321910926));
#59728=CARTESIAN_POINT('Ctrl Pts',(-4.94375172282346,-36.2742356128,-0.278410074797206));
#59729=CARTESIAN_POINT('Ctrl Pts',(-4.88577370413207,-36.2742356128,-0.34299678500102));
#59730=CARTESIAN_POINT('Ctrl Pts',(-4.82572895436385,-36.2742356128,-0.406090623479409));
#59731=CARTESIAN_POINT('Ctrl Pts',(-4.79084535329308,-36.2742356128,-0.442745623292039));
#59732=CARTESIAN_POINT('Ctrl Pts',(-4.75526528057978,-36.2742356128,-0.478897064056129));
#59733=CARTESIAN_POINT('Ctrl Pts',(-4.71903753054964,-36.2742356128,-0.514552888056171));
#59734=CARTESIAN_POINT('Ctrl Pts',(-4.64444432098229,-36.2742356128,-0.587968497629466));
#59735=CARTESIAN_POINT('Ctrl Pts',(-4.56710094042078,-36.2742356127999,
-0.659284698548609));
#59736=CARTESIAN_POINT('Ctrl Pts',(-4.48745667359651,-36.2742356128001,
-0.728608343046159));
#59737=CARTESIAN_POINT('Ctrl Pts',(-4.39811945811274,-36.2742356128004,
-0.806368885186153));
#59738=CARTESIAN_POINT('Ctrl Pts',(-4.3058889383997,-36.2742356127994,-0.881623702287833));
#59739=CARTESIAN_POINT('Ctrl Pts',(-4.21137879892378,-36.2742356128104,
-0.954588341667663));
#59740=CARTESIAN_POINT('Ctrl Pts',(-4.1488246595336,-36.2742356128176,-1.00288199828091));
#59741=CARTESIAN_POINT('Ctrl Pts',(-4.0852713916205,-36.2742356128302,-1.05017372938662));
#59742=CARTESIAN_POINT('Ctrl Pts',(-4.02088678663867,-36.2742356128628,
-1.09653320575464));
#59743=CARTESIAN_POINT('Ctrl Pts',(-3.93246496197258,-36.2742356129075,
-1.1602004363322));
#59744=CARTESIAN_POINT('Ctrl Pts',(-3.84242717112692,-36.2742356129842,
-1.22214574970036));
#59745=CARTESIAN_POINT('Ctrl Pts',(-3.75117549355878,-36.2742356130422,
-1.28253353257367));
#59746=CARTESIAN_POINT('Ctrl Pts',(-3.66800942582536,-36.2742356130951,
-1.33757048723089));
#59747=CARTESIAN_POINT('Ctrl Pts',(-3.58383519756554,-36.2742356131249,
-1.39131473192463));
#59748=CARTESIAN_POINT('Ctrl Pts',(-3.498919466185,-36.2742356130898,-1.44387055986142));
#59749=CARTESIAN_POINT('Ctrl Pts',(-3.41958194559884,-36.2742356130569,
-1.4929739357974));
#59750=CARTESIAN_POINT('Ctrl Pts',(-3.33959721867197,-36.274235612958,-1.54104048394551));
#59751=CARTESIAN_POINT('Ctrl Pts',(-3.25914673123784,-36.2742356128737,
-1.58812608964871));
#59752=CARTESIAN_POINT('Ctrl Pts',(-3.25349026788856,-36.2742356128678,
-1.59143667248585));
#59753=CARTESIAN_POINT('Ctrl Pts',(-3.24783148609435,-36.274235612862,-1.59474239134763));
#59754=CARTESIAN_POINT('Ctrl Pts',(-3.24217044152485,-36.2742356128564,
-1.59804325870171));
#59755=CARTESIAN_POINT('Ctrl Pts',(-3.17540989463343,-36.2742356127911,
-1.6369702989447));
#59756=CARTESIAN_POINT('Ctrl Pts',(-3.10833928979081,-36.2742356128,-1.67522511318535));
#59757=CARTESIAN_POINT('Ctrl Pts',(-3.04105812388561,-36.2742356128,-1.71280864441373));
#59758=CARTESIAN_POINT('Ctrl Pts',(-3.00580358073116,-36.2742356128,-1.73250197472039));
#59759=CARTESIAN_POINT('Ctrl Pts',(-2.9704911135997,-36.2742356128,-1.75200976423252));
#59760=CARTESIAN_POINT('Ctrl Pts',(-2.93513275915533,-36.2742356128,-1.77132942170696));
#59761=CARTESIAN_POINT('Ctrl Pts',(-2.90681919636723,-36.2742356128,-1.78679983438716));
#59762=CARTESIAN_POINT('Ctrl Pts',(-2.87847617925005,-36.2742356128,-1.80214958270991));
#59763=CARTESIAN_POINT('Ctrl Pts',(-2.85010907686803,-36.2742356128,-1.81737646356693));
#59764=CARTESIAN_POINT('Ctrl Pts',(-2.83489978685648,-36.2742356128,-1.82554049963262));
#59765=CARTESIAN_POINT('Ctrl Pts',(-2.81968183312169,-36.2742356128,-1.83367014577044));
#59766=CARTESIAN_POINT('Ctrl Pts',(-2.80444614119178,-36.2742356128,-1.84177010461572));
#59767=CARTESIAN_POINT('Ctrl Pts',(-2.7312492107695,-36.2742356128,-1.88068478776555));
#59768=CARTESIAN_POINT('Ctrl Pts',(-2.65771102048995,-36.2742356128,-1.91888207960992));
#59769=CARTESIAN_POINT('Ctrl Pts',(-2.58393848667699,-36.2742356128,-1.95625204730452));
#59770=CARTESIAN_POINT('Ctrl Pts',(-2.53620979668164,-36.2742356128,-1.98042933268493));
#59771=CARTESIAN_POINT('Ctrl Pts',(-2.48838235857969,-36.2742356128,-2.00425958104195));
#59772=CARTESIAN_POINT('Ctrl Pts',(-2.44047714007376,-36.2742356128,-2.02770384416305));
#59773=CARTESIAN_POINT('Ctrl Pts',(-2.41652453082079,-36.2742356128,-2.0394259757236));
#59774=CARTESIAN_POINT('Ctrl Pts',(-2.39255237409675,-36.2742356128,-2.05105149240143));
#59775=CARTESIAN_POINT('Ctrl Pts',(-2.36856266117483,-36.2742356128,-2.06257479271213));
#59776=CARTESIAN_POINT('Ctrl Pts',(-2.35274440118297,-36.2742356128,-2.07017298952559));
#59777=CARTESIAN_POINT('Ctrl Pts',(-2.33692076087942,-36.2742356128,-2.07772567107306));
#59778=CARTESIAN_POINT('Ctrl Pts',(-2.32108130896673,-36.2742356128,-2.0852362535285));
#59779=CARTESIAN_POINT('Ctrl Pts',(-2.31289890863895,-36.2742356128,-2.08911609688949));
#59780=CARTESIAN_POINT('Ctrl Pts',(-2.30471404262477,-36.2742356128,-2.09298385940345));
#59781=CARTESIAN_POINT('Ctrl Pts',(-2.29653265536,-36.2742356128,-2.09683653367));
#59782=CARTESIAN_POINT('',(-9.72829200583979,-36.2742356128,2.64855052067506));
#59783=CARTESIAN_POINT('Ctrl Pts',(-9.72829200283952,-36.2742356128,2.64855051884389));
#59784=CARTESIAN_POINT('Ctrl Pts',(-9.70881714164152,-36.2742356128,2.68045885667498));
#59785=CARTESIAN_POINT('Ctrl Pts',(-9.68889475699523,-36.2742356127939,
2.71236488661939));
#59786=CARTESIAN_POINT('Ctrl Pts',(-9.66845938327075,-36.2742356128061,
2.74429101374004));
#59787=CARTESIAN_POINT('Ctrl Pts',(-9.64722469389298,-36.2742356128187,
2.7774659094666));
#59788=CARTESIAN_POINT('Ctrl Pts',(-9.62543546500888,-36.2742356127916,
2.81066258335515));
#59789=CARTESIAN_POINT('Ctrl Pts',(-9.60300164534709,-36.2742356132359,
2.84385119710766));
#59790=CARTESIAN_POINT('Ctrl Pts',(-9.58651192372458,-36.2742356135625,
2.86824610667128));
#59791=CARTESIAN_POINT('Ctrl Pts',(-9.56967353061277,-36.2742356141378,
2.89263545845183));
#59792=CARTESIAN_POINT('Ctrl Pts',(-9.55244862998868,-36.2742356157403,
2.91698968329831));
#59793=CARTESIAN_POINT('Ctrl Pts',(-9.53980531242101,-36.2742356169165,
2.93486602439127));
#59794=CARTESIAN_POINT('Ctrl Pts',(-9.52696074018631,-36.2742356188376,
2.95271192605641));
#59795=CARTESIAN_POINT('Ctrl Pts',(-9.51385958563359,-36.2742356221257,
2.97056761705111));
#59796=CARTESIAN_POINT('Ctrl Pts',(-9.48902877144369,-36.2742356283578,
3.0044097752775));
#59797=CARTESIAN_POINT('Ctrl Pts',(-9.46324980492634,-36.2742356393454,
3.03832837506574));
#59798=CARTESIAN_POINT('Ctrl Pts',(-9.43647539801905,-36.2742356478859,
3.072103909518));
#59799=CARTESIAN_POINT('Ctrl Pts',(-9.4100087918541,-36.2742356563283,3.10549115770071));
#59800=CARTESIAN_POINT('Ctrl Pts',(-9.38256837684105,-36.2742356607735,
3.13873761718217));
#59801=CARTESIAN_POINT('Ctrl Pts',(-9.35414272876498,-36.2742356533727,
3.17159442011749));
#59802=CARTESIAN_POINT('Ctrl Pts',(-9.34981362475727,-36.2742356522455,
3.17659836996191));
#59803=CARTESIAN_POINT('Ctrl Pts',(-9.34546175267801,-36.2742356508755,
3.18159322937679));
#59804=CARTESIAN_POINT('Ctrl Pts',(-9.34108716705853,-36.2742356492836,
3.18657806784048));
#59805=CARTESIAN_POINT('Ctrl Pts',(-9.32533707496848,-36.2742356435521,
3.20452529111746));
#59806=CARTESIAN_POINT('Ctrl Pts',(-9.30928255086254,-36.2742356380445,
3.2223449918369));
#59807=CARTESIAN_POINT('Ctrl Pts',(-9.29289822512316,-36.2742356335668,
3.24001817562276));
#59808=CARTESIAN_POINT('Ctrl Pts',(-9.27651389938378,-36.2742356290892,
3.25769135940861));
#59809=CARTESIAN_POINT('Ctrl Pts',(-9.25978052146042,-36.2742356248894,
3.27524193625796));
#59810=CARTESIAN_POINT('Ctrl Pts',(-9.24266879473122,-36.2742356217968,
3.29264736551428));
#59811=CARTESIAN_POINT('Ctrl Pts',(-9.21166804126147,-36.2742356161942,
3.32418021020898));
#59812=CARTESIAN_POINT('Ctrl Pts',(-9.17946812786415,-36.274235614416,3.35518678266736));
#59813=CARTESIAN_POINT('Ctrl Pts',(-9.14603905518141,-36.2742356135611,
3.38542077511821));
#59814=CARTESIAN_POINT('Ctrl Pts',(-9.11365966829153,-36.2742356127332,
3.41470540852945));
#59815=CARTESIAN_POINT('Ctrl Pts',(-9.08012671258212,-36.2742356128071,
3.44326464800626));
#59816=CARTESIAN_POINT('Ctrl Pts',(-9.04545810927638,-36.2742356128011,
3.47085541290006));
#59817=CARTESIAN_POINT('Ctrl Pts',(-9.03688320628073,-36.2742356127996,
3.4776796893341));
#59818=CARTESIAN_POINT('Ctrl Pts',(-9.02823906549762,-36.2742356128,3.48444464576843));
#59819=CARTESIAN_POINT('Ctrl Pts',(-9.0195264422119,-36.2742356128,3.49114647591936));
#59820=CARTESIAN_POINT('Ctrl Pts',(-8.98770603560951,-36.2742356128,3.51562302602248));
#59821=CARTESIAN_POINT('Ctrl Pts',(-8.95495184342817,-36.2742356128,3.53927487380998));
#59822=CARTESIAN_POINT('Ctrl Pts',(-8.92126202698245,-36.2742356128,3.56194807661424));
#59823=CARTESIAN_POINT('Ctrl Pts',(-8.91092880879014,-36.2742356128,3.56890231906528));
#59824=CARTESIAN_POINT('Ctrl Pts',(-8.90050794619933,-36.2742356128,3.57576445922664));
#59825=CARTESIAN_POINT('Ctrl Pts',(-8.89000034786166,-36.2742356128,3.58252999939621));
#59826=CARTESIAN_POINT('Ctrl Pts',(-8.85417163483683,-36.2742356128,3.60559907659196));
#59827=CARTESIAN_POINT('Ctrl Pts',(-8.81731612594884,-36.2742356128,3.6275536106033));
#59828=CARTESIAN_POINT('Ctrl Pts',(-8.77950365203068,-36.2742356128,3.64821448776519));
#59829=CARTESIAN_POINT('Ctrl Pts',(-8.77007157519482,-36.2742356128,3.65336820982287));
#59830=CARTESIAN_POINT('Ctrl Pts',(-8.76058020706037,-36.2742356128,3.65844147391791));
#59831=CARTESIAN_POINT('Ctrl Pts',(-8.75103111774342,-36.2742356128,3.66343159406543));
#59832=CARTESIAN_POINT('Ctrl Pts',(-8.71119259904518,-36.2742356128,3.68425022799007));
#59833=CARTESIAN_POINT('Ctrl Pts',(-8.67032239058182,-36.2742356128,3.70363224949672));
#59834=CARTESIAN_POINT('Ctrl Pts',(-8.62855784922379,-36.2742356128,3.72139135357447));
#59835=CARTESIAN_POINT('Ctrl Pts',(-8.62017492022797,-36.2742356128,3.72495593979216));
#59836=CARTESIAN_POINT('Ctrl Pts',(-8.6117561124818,-36.2742356128,3.72845521369156));
#59837=CARTESIAN_POINT('Ctrl Pts',(-8.60330275640969,-36.2742356128,3.7318877882704));
#59838=CARTESIAN_POINT('Ctrl Pts',(-8.56260230061348,-36.2742356128,3.74841463852037));
#59839=CARTESIAN_POINT('Ctrl Pts',(-8.52106780561381,-36.2742356127477,
3.76340465617139));
#59840=CARTESIAN_POINT('Ctrl Pts',(-8.47888591381473,-36.2742356128523,
3.77670246412333));
#59841=CARTESIAN_POINT('Ctrl Pts',(-8.46865840584675,-36.2742356128777,
3.77992667790285));
#59842=CARTESIAN_POINT('Ctrl Pts',(-8.4583930024119,-36.2742356129174,3.78305158595824));
#59843=CARTESIAN_POINT('Ctrl Pts',(-8.44809265827065,-36.2742356129926,
3.78607533346085));
#59844=CARTESIAN_POINT('Ctrl Pts',(-8.40414425667525,-36.2742356133133,
3.79897673439904));
#59845=CARTESIAN_POINT('Ctrl Pts',(-8.35956591318086,-36.2742356136175,
3.81004533329349));
#59846=CARTESIAN_POINT('Ctrl Pts',(-8.31455927271245,-36.2742356135546,
3.81918158877721));
#59847=CARTESIAN_POINT('Ctrl Pts',(-8.2708985149816,-36.2742356134935,3.82804463283228));
#59848=CARTESIAN_POINT('Ctrl Pts',(-8.22683534940045,-36.2742356132172,
3.83508870122784));
#59849=CARTESIAN_POINT('Ctrl Pts',(-8.18256835517632,-36.2742356130434,
3.84026882783139));
#59850=CARTESIAN_POINT('Ctrl Pts',(-8.14029162176882,-36.2742356128773,
3.84521605398202));
#59851=CARTESIAN_POINT('Ctrl Pts',(-8.0978294896405,-36.2742356128133,3.84846295530726));
#59852=CARTESIAN_POINT('Ctrl Pts',(-8.05536002370458,-36.2742356128032,
3.85001759540461));
#59853=CARTESIAN_POINT('Ctrl Pts',(-8.03833269714543,-36.2742356127992,
3.85064089885419));
#59854=CARTESIAN_POINT('Ctrl Pts',(-8.02130420979561,-36.2742356128,3.85099274476445));
#59855=CARTESIAN_POINT('Ctrl Pts',(-8.0042860115659,-36.2742356128,3.85107605173954));
#59856=CARTESIAN_POINT('Ctrl Pts',(-7.9599310512507,-36.2742356128,3.85129317681496));
#59857=CARTESIAN_POINT('Ctrl Pts',(-7.91563944625556,-36.2742356129104,
3.84967518465513));
#59858=CARTESIAN_POINT('Ctrl Pts',(-7.87158021912379,-36.2742356132959,
3.84626457629435));
#59859=CARTESIAN_POINT('Ctrl Pts',(-7.84149821150494,-36.2742356135591,
3.84393593928973));
#59860=CARTESIAN_POINT('Ctrl Pts',(-7.81152457443802,-36.2742356137885,
3.84077293715099));
#59861=CARTESIAN_POINT('Ctrl Pts',(-7.78171169682192,-36.2742356135375,
3.83680279283792));
#59862=CARTESIAN_POINT('Ctrl Pts',(-7.74497551896622,-36.2742356132282,
3.83191068113117));
#59863=CARTESIAN_POINT('Ctrl Pts',(-7.70847517960959,-36.2742356128376,
3.82578856669653));
#59864=CARTESIAN_POINT('Ctrl Pts',(-7.67230948527672,-36.2742356128125,
3.81848117117423));
#59865=CARTESIAN_POINT('Ctrl Pts',(-7.63614379094206,-36.2742356127875,
3.81117377565156));
#59866=CARTESIAN_POINT('Ctrl Pts',(-7.60030599244742,-36.2742356128,3.8026864810845));
#59867=CARTESIAN_POINT('Ctrl Pts',(-7.56485464772436,-36.2742356128,3.79308618073687));
#59868=CARTESIAN_POINT('Ctrl Pts',(-7.51614449460733,-36.2742356128,3.77989536657861));
#59869=CARTESIAN_POINT('Ctrl Pts',(-7.46815457775148,-36.2742356128,3.76459822919188));
#59870=CARTESIAN_POINT('Ctrl Pts',(-7.42109393627412,-36.2742356128,3.74740524786678));
#59871=CARTESIAN_POINT('Ctrl Pts',(-7.37554524515301,-36.2742356128,3.7307646375554));
#59872=CARTESIAN_POINT('Ctrl Pts',(-7.33086784647416,-36.2742356128,3.71234961793179));
#59873=CARTESIAN_POINT('Ctrl Pts',(-7.28720664579929,-36.2742356128,3.69236808034837));
#59874=CARTESIAN_POINT('Ctrl Pts',(-7.25324153041755,-36.2742356128,3.67682395377753));
#59875=CARTESIAN_POINT('Ctrl Pts',(-7.2198880141248,-36.2742356128,3.66033091549968));
#59876=CARTESIAN_POINT('Ctrl Pts',(-7.18720047173584,-36.2742356128,3.64299101963176));
#59877=CARTESIAN_POINT('Ctrl Pts',(-7.16357818122735,-36.2742356128,3.63046000543972));
#59878=CARTESIAN_POINT('Ctrl Pts',(-7.14030418161754,-36.2742356127951,
3.61748764102144));
#59879=CARTESIAN_POINT('Ctrl Pts',(-7.11736987557029,-36.2742356128049,
3.60409577182642));
#59880=CARTESIAN_POINT('Ctrl Pts',(-7.08175075284689,-36.27423561282,3.58329694619941));
#59881=CARTESIAN_POINT('Ctrl Pts',(-7.04694106975427,-36.2742356128032,
3.56149027437102));
#59882=CARTESIAN_POINT('Ctrl Pts',(-7.0129444202984,-36.2742356128006,3.53877467325613));
#59883=CARTESIAN_POINT('Ctrl Pts',(-7.00316458010594,-36.2742356127999,
3.53224006021823));
#59884=CARTESIAN_POINT('Ctrl Pts',(-6.99345173196612,-36.2742356128,3.5256300856373));
#59885=CARTESIAN_POINT('Ctrl Pts',(-6.98380523431276,-36.2742356128,3.51894671931244));
#59886=CARTESIAN_POINT('Ctrl Pts',(-6.93692149920594,-36.2742356128,3.48646434201277));
#59887=CARTESIAN_POINT('Ctrl Pts',(-6.89160109645423,-36.2742356127441,
3.45225020263866));
#59888=CARTESIAN_POINT('Ctrl Pts',(-6.84780885039552,-36.2742356131978,
3.41649930066148));
#59889=CARTESIAN_POINT('Ctrl Pts',(-6.80350698393218,-36.2742356136568,
3.38033235724384));
#59890=CARTESIAN_POINT('Ctrl Pts',(-6.76076867429983,-36.274235614773,3.34259238553588));
#59891=CARTESIAN_POINT('Ctrl Pts',(-6.71957759739078,-36.2742356160617,
3.30343121875042));
#59892=CARTESIAN_POINT('Ctrl Pts',(-6.67781355062949,-36.2742356173683,
3.26372531825973));
#59893=CARTESIAN_POINT('Ctrl Pts',(-6.6376396712846,-36.2742356186979,3.22255810360343));
#59894=CARTESIAN_POINT('Ctrl Pts',(-6.5990654582959,-36.2742356185244,3.18004119693173));
#59895=CARTESIAN_POINT('Ctrl Pts',(-6.57718261135267,-36.274235618426,3.15592169094288));
#59896=CARTESIAN_POINT('Ctrl Pts',(-6.55581508439785,-36.2742356178269,
3.1313670070968));
#59897=CARTESIAN_POINT('Ctrl Pts',(-6.53496908430346,-36.2742356168316,
3.10639158569407));
#59898=CARTESIAN_POINT('Ctrl Pts',(-6.49664188907379,-36.2742356150015,
3.06047208805849));
#59899=CARTESIAN_POINT('Ctrl Pts',(-6.46006641236599,-36.2742356135502,
3.01310950800297));
#59900=CARTESIAN_POINT('Ctrl Pts',(-6.42534220694393,-36.2742356130965,
2.96437182473463));
#59901=CARTESIAN_POINT('Ctrl Pts',(-6.40199804386673,-36.2742356127915,
2.93160677187331));
#59902=CARTESIAN_POINT('Ctrl Pts',(-6.37949136823164,-36.2742356128032,
2.89821949802322));
#59903=CARTESIAN_POINT('Ctrl Pts',(-6.35786343822196,-36.2742356128012,
2.86422329401434));
#59904=CARTESIAN_POINT('Ctrl Pts',(-6.33095671764626,-36.2742356127988,
2.82192953952689));
#59905=CARTESIAN_POINT('Ctrl Pts',(-6.30539306828795,-36.2742356128,2.77867851495301));
#59906=CARTESIAN_POINT('Ctrl Pts',(-6.28127323414043,-36.2742356128,2.73448936390555));
#59907=CARTESIAN_POINT('Ctrl Pts',(-6.27915867338878,-36.2742356128,2.73061534703287));
#59908=CARTESIAN_POINT('Ctrl Pts',(-6.27705587738,-36.2742356128,2.72673532671));
#59909=CARTESIAN_POINT('Ctrl Pts',(-6.27496307903,-36.2742356128,2.72284588841));
#59910=CARTESIAN_POINT('',(-10.3535103411566,-36.2742356128,0.692258559169219));
#59911=CARTESIAN_POINT('Ctrl Pts',(-10.3535102174,-36.2742356128,0.692259289483));
#59912=CARTESIAN_POINT('Ctrl Pts',(-10.3480579903016,-36.2742356128,0.727045462316002));
#59913=CARTESIAN_POINT('Ctrl Pts',(-10.3425213376762,-36.2742356128,0.761582529081522));
#59914=CARTESIAN_POINT('Ctrl Pts',(-10.3368982634255,-36.2742356128,0.796052242175564));
#59915=CARTESIAN_POINT('Ctrl Pts',(-10.3310793079616,-36.2742356128,0.831722716439654));
#59916=CARTESIAN_POINT('Ctrl Pts',(-10.3251675908898,-36.2742356128,0.867321117622198));
#59917=CARTESIAN_POINT('Ctrl Pts',(-10.3191354058366,-36.2742356128,0.902998219346001));
#59918=CARTESIAN_POINT('Ctrl Pts',(-10.3129769350349,-36.2742356128,0.939422232753249));
#59919=CARTESIAN_POINT('Ctrl Pts',(-10.3066925671242,-36.2742356128,0.975928187824864));
#59920=CARTESIAN_POINT('Ctrl Pts',(-10.3002309954935,-36.2742356128,1.01262505579727));
#59921=CARTESIAN_POINT('Ctrl Pts',(-10.293530416437,-36.2742356128,1.05067930622249));
#59922=CARTESIAN_POINT('Ctrl Pts',(-10.2866389091829,-36.2742356128,1.08893886185183));
#59923=CARTESIAN_POINT('Ctrl Pts',(-10.2794814194908,-36.2742356128,1.1274708876644));
#59924=CARTESIAN_POINT('Ctrl Pts',(-10.2737499087197,-36.2742356128,1.15832621969877));
#59925=CARTESIAN_POINT('Ctrl Pts',(-10.2678473908321,-36.2742356128,1.18935513968225));
#59926=CARTESIAN_POINT('Ctrl Pts',(-10.2617301906119,-36.2742356128,1.22056871200232));
#59927=CARTESIAN_POINT('Ctrl Pts',(-10.2537209481499,-36.2742356128,1.26143660251052));
#59928=CARTESIAN_POINT('Ctrl Pts',(-10.2453441318077,-36.2742356128,1.30261904015665));
#59929=CARTESIAN_POINT('Ctrl Pts',(-10.2364970665051,-36.2742356128,1.34409448776794));
#59930=CARTESIAN_POINT('Ctrl Pts',(-10.2273826990709,-36.2742356128,1.38682306002305));
#59931=CARTESIAN_POINT('Ctrl Pts',(-10.217768515935,-36.2742356128,1.42986240026419));
#59932=CARTESIAN_POINT('Ctrl Pts',(-10.207546645515,-36.2742356128,1.47313438920396));
#59933=CARTESIAN_POINT('Ctrl Pts',(-10.2056609342062,-36.2742356128,1.48111712382525));
#59934=CARTESIAN_POINT('Ctrl Pts',(-10.2037545714597,-36.2742356128,1.4891076361342));
#59935=CARTESIAN_POINT('Ctrl Pts',(-10.2018269270533,-36.2742356128,1.49710525066367));
#59936=CARTESIAN_POINT('Ctrl Pts',(-10.191131512178,-36.2742356128,1.54147951654082));
#59937=CARTESIAN_POINT('Ctrl Pts',(-10.179777778705,-36.2742356128,1.58608219549579));
#59938=CARTESIAN_POINT('Ctrl Pts',(-10.16766492246,-36.2742356128,1.6307873871189));
#59939=CARTESIAN_POINT('Ctrl Pts',(-10.1669020529659,-36.2742356128,1.63360292675943));
#59940=CARTESIAN_POINT('Ctrl Pts',(-10.1661361802017,-36.2742356128,1.63641885774768));
#59941=CARTESIAN_POINT('Ctrl Pts',(-10.1653672823159,-36.2742356128,1.63923514258223));
#59942=CARTESIAN_POINT('Ctrl Pts',(-10.1523898092668,-36.2742356128,1.68676845124615));
#59943=CARTESIAN_POINT('Ctrl Pts',(-10.1385595407206,-36.2742356128,1.73436882358064));
#59944=CARTESIAN_POINT('Ctrl Pts',(-10.123819450048,-36.2742356128,1.78185933117367));
#59945=CARTESIAN_POINT('Ctrl Pts',(-10.1070954365052,-36.2742356128,1.8357417603786));
#59946=CARTESIAN_POINT('Ctrl Pts',(-10.0891534135,-36.2742356127716,1.88957161512486));
#59947=CARTESIAN_POINT('Ctrl Pts',(-10.069899218258,-36.274235614767,1.94320888333938));
#59948=CARTESIAN_POINT('Ctrl Pts',(-10.0549879588562,-36.2742356163123,
1.98474784198701));
#59949=CARTESIAN_POINT('Ctrl Pts',(-10.0392893023929,-36.2742356190629,
2.02617198779279));
#59950=CARTESIAN_POINT('Ctrl Pts',(-10.0227819439559,-36.2742356205281,
2.06741497935644));
#59951=CARTESIAN_POINT('Ctrl Pts',(-10.0055355624289,-36.2742356220589,
2.11050439130175));
#59952=CARTESIAN_POINT('Ctrl Pts',(-9.98745291704985,-36.2742356220055,
2.15327460749465));
#59953=CARTESIAN_POINT('Ctrl Pts',(-9.96854770915045,-36.2742356203452,
2.19566393769648));
#59954=CARTESIAN_POINT('Ctrl Pts',(-9.96662228141052,-36.2742356201761,
2.19998113921482));
#59955=CARTESIAN_POINT('Ctrl Pts',(-9.96468836454892,-36.274235619993,2.20429437570766));
#59956=CARTESIAN_POINT('Ctrl Pts',(-9.96274600376888,-36.2742356197975,
2.20860357150312));
#59957=CARTESIAN_POINT('Ctrl Pts',(-9.94548075860643,-36.2742356180606,
2.24690712593345));
#59958=CARTESIAN_POINT('Ctrl Pts',(-9.92754090731581,-36.2742356158519,
2.28489765236143));
#59959=CARTESIAN_POINT('Ctrl Pts',(-9.90897813049164,-36.2742356146521,
2.32250503559895));
#59960=CARTESIAN_POINT('Ctrl Pts',(-9.90494782982202,-36.2742356143916,
2.33067025049546));
#59961=CARTESIAN_POINT('Ctrl Pts',(-9.90088834402933,-36.2742356141686,
2.33881733230838));
#59962=CARTESIAN_POINT('Ctrl Pts',(-9.89680051537798,-36.2742356139816,
2.34694543639459));
#59963=CARTESIAN_POINT('Ctrl Pts',(-9.87951639572504,-36.2742356131909,
2.38131261162618));
#59964=CARTESIAN_POINT('Ctrl Pts',(-9.86170905446685,-36.2742356130057,
2.41536635168401));
#59965=CARTESIAN_POINT('Ctrl Pts',(-9.84349333770681,-36.2742356129026,
2.44899524721528));
#59966=CARTESIAN_POINT('Ctrl Pts',(-9.82538061717865,-36.2742356128,2.48243399653557));
#59967=CARTESIAN_POINT('Ctrl Pts',(-9.80686377000502,-36.2742356128048,
2.51545283764242));
#59968=CARTESIAN_POINT('Ctrl Pts',(-9.78810607413667,-36.2742356128016,
2.54792653892519));
#59969=CARTESIAN_POINT('Ctrl Pts',(-9.76934837826831,-36.2742356127984,
2.58040024020796));
#59970=CARTESIAN_POINT('Ctrl Pts',(-9.75034951548812,-36.2742356128,2.61232893171438));
#59971=CARTESIAN_POINT('Ctrl Pts',(-9.73132840842276,-36.2742356128,2.64356954426823));
#59972=CARTESIAN_POINT('Ctrl Pts',(-9.73031636916408,-36.2742356128,2.64523173597248));
#59973=CARTESIAN_POINT('Ctrl Pts',(-9.72930457700097,-36.2742356128,2.64689149083652));
#59974=CARTESIAN_POINT('Ctrl Pts',(-9.72829200824,-36.2742356128,2.64855052214));
#59975=CARTESIAN_POINT('Ctrl Pts',(-2.11953809549828,-36.2742356128,-9.31090088052415));
#59976=CARTESIAN_POINT('Ctrl Pts',(-2.1432042809605,-36.2742356128,-9.30658861277567));
#59977=CARTESIAN_POINT('Ctrl Pts',(-2.16685412882638,-36.2742356128,-9.30220459811138));
#59978=CARTESIAN_POINT('Ctrl Pts',(-2.19048902654178,-36.2742356128,-9.29774821966819));
#59979=CARTESIAN_POINT('Ctrl Pts',(-2.35462317202845,-36.2742356128,-9.26680059820831));
#59980=CARTESIAN_POINT('Ctrl Pts',(-2.51797534469943,-36.2742356128001,
-9.23237423419211));
#59981=CARTESIAN_POINT('Ctrl Pts',(-2.68029691391768,-36.2742356128001,
-9.19440935897591));
#59982=CARTESIAN_POINT('Ctrl Pts',(-2.84229564204318,-36.2742356128001,
-9.1565199920354));
#59983=CARTESIAN_POINT('Ctrl Pts',(-3.00326827555196,-36.2742356128001,
-9.11510506553852));
#59984=CARTESIAN_POINT('Ctrl Pts',(-3.16301674313939,-36.2742356128001,
-9.07011799870195));
#59985=CARTESIAN_POINT('Ctrl Pts',(-3.31930702526653,-36.2742356128001,
-9.0261047979862));
#59986=CARTESIAN_POINT('Ctrl Pts',(-3.47442608318702,-36.2742356128,-8.97867151143555));
#59987=CARTESIAN_POINT('Ctrl Pts',(-3.62822837685435,-36.2742356128,-8.9278017362869));
#59988=CARTESIAN_POINT('Ctrl Pts',(-3.78139308336189,-36.2742356128,-8.8771428417089));
#59989=CARTESIAN_POINT('Ctrl Pts',(-3.93325229434668,-36.2742356128,-8.82307493906309));
#59990=CARTESIAN_POINT('Ctrl Pts',(-4.08369592329912,-36.2742356128,-8.7656231571103));
#59991=CARTESIAN_POINT('Ctrl Pts',(-4.22435201933401,-36.2742356128,-8.71190906222974));
#59992=CARTESIAN_POINT('Ctrl Pts',(-4.36377126817408,-36.2742356128,-8.65523679979434));
#59993=CARTESIAN_POINT('Ctrl Pts',(-4.50188619308555,-36.2742356128,-8.59567086336398));
#59994=CARTESIAN_POINT('Ctrl Pts',(-4.51149689899936,-36.2742356128,-8.59152597679303));
#59995=CARTESIAN_POINT('Ctrl Pts',(-4.52110129710902,-36.2742356128,-8.58736709855662));
#59996=CARTESIAN_POINT('Ctrl Pts',(-4.53069936809608,-36.2742356128,-8.58319425943421));
#59997=CARTESIAN_POINT('Ctrl Pts',(-4.653905380685,-36.2742356128,-8.52962944728182));
#59998=CARTESIAN_POINT('Ctrl Pts',(-4.77607707362801,-36.2742356128,-8.47375564208602));
#59999=CARTESIAN_POINT('Ctrl Pts',(-4.89716285107826,-36.2742356128,-8.41561384004806));
#60000=CARTESIAN_POINT('Ctrl Pts',(-5.02947170663252,-36.2742356128,-8.35208304849275));
#60001=CARTESIAN_POINT('Ctrl Pts',(-5.1604834473911,-36.2742356128,-8.28584521369305));
#60002=CARTESIAN_POINT('Ctrl Pts',(-5.29014337296856,-36.2742356128,-8.21701574955886));
#60003=CARTESIAN_POINT('Ctrl Pts',(-5.37098118845278,-36.2742356128,-8.174103311527));
#60004=CARTESIAN_POINT('Ctrl Pts',(-5.45129383189978,-36.2742356128,-8.13018468581161));
#60005=CARTESIAN_POINT('Ctrl Pts',(-5.53107177181599,-36.2742356128,-8.08529551782231));
#60006=CARTESIAN_POINT('Ctrl Pts',(-5.60994290563681,-36.2742356128,-8.04091658826725));
#60007=CARTESIAN_POINT('Ctrl Pts',(-5.68829912285867,-36.2742356128,-7.99558484614536));
#60008=CARTESIAN_POINT('Ctrl Pts',(-5.76613073017276,-36.2742356128,-7.94933895772168));
#60009=CARTESIAN_POINT('Ctrl Pts',(-5.89632002798005,-36.2742356128,-7.87198324134728));
#60010=CARTESIAN_POINT('Ctrl Pts',(-6.02503595167037,-36.2742356128,-7.79207291887174));
#60011=CARTESIAN_POINT('Ctrl Pts',(-6.1522441308659,-36.2742356128,-7.70979855315438));
#60012=CARTESIAN_POINT('Ctrl Pts',(-6.27232259158325,-36.2742356128,-7.63213547162681));
#60013=CARTESIAN_POINT('Ctrl Pts',(-6.39105751633973,-36.2742356128,-7.55236760087967));
#60014=CARTESIAN_POINT('Ctrl Pts',(-6.50845458459874,-36.2742356128,-7.47062987547745));
#60015=CARTESIAN_POINT('Ctrl Pts',(-6.61234621683071,-36.2742356128,-7.39829531182181));
#60016=CARTESIAN_POINT('Ctrl Pts',(-6.71520102544753,-36.2742356127886,
-7.32441168797259));
#60017=CARTESIAN_POINT('Ctrl Pts',(-6.81708760544559,-36.2742356128114,
-7.24900408693246));
#60018=CARTESIAN_POINT('Ctrl Pts',(-6.86842159421278,-36.2742356128229,
-7.21101112510345));
#60019=CARTESIAN_POINT('Ctrl Pts',(-6.919510141846,-36.2742356128435,-7.17263064176347));
#60020=CARTESIAN_POINT('Ctrl Pts',(-6.97036425874489,-36.2742356129319,
-7.13386121169139));
#60021=CARTESIAN_POINT('Ctrl Pts',(-7.06478009632977,-36.274235613096,-7.0618818236662));
#60022=CARTESIAN_POINT('Ctrl Pts',(-7.15843501790257,-36.2742356129223,
-6.98854451497165));
#60023=CARTESIAN_POINT('Ctrl Pts',(-7.25136378947047,-36.2742356128455,
-6.91383222628363));
#60024=CARTESIAN_POINT('Ctrl Pts',(-7.30783258389914,-36.2742356127988,
-6.86843280046494));
#60025=CARTESIAN_POINT('Ctrl Pts',(-7.36403369072445,-36.2742356128,-6.8225248802803));
#60026=CARTESIAN_POINT('Ctrl Pts',(-7.41997923973695,-36.2742356128,-6.7760961334252));
#60027=CARTESIAN_POINT('Ctrl Pts',(-7.52440937719628,-36.2742356128,-6.68943042897284));
#60028=CARTESIAN_POINT('Ctrl Pts',(-7.62796140085615,-36.2742356128,-6.60095511075596));
#60029=CARTESIAN_POINT('Ctrl Pts',(-7.73046643660877,-36.2742356128,-6.51068806246407));
#60030=CARTESIAN_POINT('Ctrl Pts',(-7.83073696140362,-36.2742356128,-6.42238874880153));
#60031=CARTESIAN_POINT('Ctrl Pts',(-7.93000558009221,-36.2742356128,-6.33237534185209));
#60032=CARTESIAN_POINT('Ctrl Pts',(-8.02807297507958,-36.2742356128,-6.2406374376305));
#60033=CARTESIAN_POINT('Ctrl Pts',(-8.12407285064597,-36.2742356128,-6.15083361046521));
#60034=CARTESIAN_POINT('Ctrl Pts',(-8.21892155557018,-36.2742356128,-6.05937754589244));
#60035=CARTESIAN_POINT('Ctrl Pts',(-8.31239309349182,-36.2742356128,-5.96622819442902));
#60036=CARTESIAN_POINT('Ctrl Pts',(-8.4031368230666,-36.2742356128,-5.87579724884696));
#60037=CARTESIAN_POINT('Ctrl Pts',(-8.4925824812243,-36.2742356128,-5.7837706089873));
#60038=CARTESIAN_POINT('Ctrl Pts',(-8.58048747027233,-36.2742356128,-5.6900772537884));
#60039=CARTESIAN_POINT('Ctrl Pts',(-8.66700528995599,-36.2742356128,-5.59786241025743));
#60040=CARTESIAN_POINT('Ctrl Pts',(-8.75203065067016,-36.2742356128,-5.50403327768024));
#60041=CARTESIAN_POINT('Ctrl Pts',(-8.83529796619582,-36.2742356128,-5.4084859080225));
#60042=CARTESIAN_POINT('Ctrl Pts',(-8.91673430633736,-36.2742356128,-5.31503954139046));
#60043=CARTESIAN_POINT('Ctrl Pts',(-8.99648900098376,-36.2742356128,-5.21994983342886));
#60044=CARTESIAN_POINT('Ctrl Pts',(-9.07428130247451,-36.2742356128,-5.12308174646508));
#60045=CARTESIAN_POINT('Ctrl Pts',(-9.11371256086522,-36.2742356128,-5.07398137928625));
#60046=CARTESIAN_POINT('Ctrl Pts',(-9.15263911624697,-36.2742356128,-5.02442347780941));
#60047=CARTESIAN_POINT('Ctrl Pts',(-9.19102120553304,-36.2742356128,-4.97438641806384));
#60048=CARTESIAN_POINT('Ctrl Pts',(-9.27135473353872,-36.2742356128,-4.86965909302337));
#60049=CARTESIAN_POINT('Ctrl Pts',(-9.34931008261837,-36.2742356128,-4.76281768826537));
#60050=CARTESIAN_POINT('Ctrl Pts',(-9.4243664421214,-36.2742356128,-4.65380960606161));
#60051=CARTESIAN_POINT('Ctrl Pts',(-9.47733401721219,-36.2742356128,-4.57688216356558));
#60052=CARTESIAN_POINT('Ctrl Pts',(-9.52885782823991,-36.2742356128,-4.49887605020695));
#60053=CARTESIAN_POINT('Ctrl Pts',(-9.57876242917955,-36.2742356128,-4.41978698025841));
#60054=CARTESIAN_POINT('Ctrl Pts',(-9.61242567371991,-36.2742356128,-4.36643729602053));
#60055=CARTESIAN_POINT('Ctrl Pts',(-9.64535662293559,-36.2742356128,-4.31258838992345));
#60056=CARTESIAN_POINT('Ctrl Pts',(-9.6775073418473,-36.2742356128,-4.25823628901775));
#60057=CARTESIAN_POINT('Ctrl Pts',(-9.73227334817142,-36.2742356128,-4.1656521228563));
#60058=CARTESIAN_POINT('Ctrl Pts',(-9.78477154511798,-36.2742356128,-4.07160923888473));
#60059=CARTESIAN_POINT('Ctrl Pts',(-9.83477068606681,-36.2742356128,-3.97613665347847));
#60060=CARTESIAN_POINT('Ctrl Pts',(-9.86501146635147,-36.2742356128,-3.91839235180268));
#60061=CARTESIAN_POINT('Ctrl Pts',(-9.89433851557226,-36.2742356128,-3.86012577086578));
#60062=CARTESIAN_POINT('Ctrl Pts',(-9.92270588308633,-36.2742356128,-3.80135120370847));
#60063=CARTESIAN_POINT('Ctrl Pts',(-9.96655495577847,-36.2742356128,-3.71049997239656));
#60064=CARTESIAN_POINT('Ctrl Pts',(-10.0081226102412,-36.2742356128,-3.61840409165624));
#60065=CARTESIAN_POINT('Ctrl Pts',(-10.0472459446408,-36.2742356128,-3.52517965095815));
#60066=CARTESIAN_POINT('Ctrl Pts',(-10.0837578615216,-36.2742356128,-3.43817778666758));
#60067=CARTESIAN_POINT('Ctrl Pts',(-10.1181408830724,-36.2742356128,-3.3501931104458));
#60068=CARTESIAN_POINT('Ctrl Pts',(-10.1502938375145,-36.2742356128,-3.26135920624506));
#60069=CARTESIAN_POINT('Ctrl Pts',(-10.1525934918653,-36.2742356128,-3.25500559806695));
#60070=CARTESIAN_POINT('Ctrl Pts',(-10.1548817525012,-36.2742356128,-3.24864766298652));
#60071=CARTESIAN_POINT('Ctrl Pts',(-10.1571585890232,-36.2742356128,-3.24228545796934));
#60072=CARTESIAN_POINT('Ctrl Pts',(-10.1873913807981,-36.2742356128,-3.1578054271638));
#60073=CARTESIAN_POINT('Ctrl Pts',(-10.2156163880341,-36.2742356128,-3.07254357398699));
#60074=CARTESIAN_POINT('Ctrl Pts',(-10.2417876145186,-36.2742356128,-2.98665974253318));
#60075=CARTESIAN_POINT('Ctrl Pts',(-10.2689167782626,-36.2742356128,-2.89763233192031));
#60076=CARTESIAN_POINT('Ctrl Pts',(-10.2938392644185,-36.2742356128,-2.80793667316511));
#60077=CARTESIAN_POINT('Ctrl Pts',(-10.3165575839241,-36.2742356128,-2.7177359139567));
#60078=CARTESIAN_POINT('Ctrl Pts',(-10.3213777705173,-36.2742356128,-2.69859785710684));
#60079=CARTESIAN_POINT('Ctrl Pts',(-10.326098911838,-36.2742356128,-2.67943700760276));
#60080=CARTESIAN_POINT('Ctrl Pts',(-10.330721313039,-36.2742356128,-2.66025483528842));
#60081=CARTESIAN_POINT('Ctrl Pts',(-10.3528699418875,-36.2742356128,-2.56834182371183));
#60082=CARTESIAN_POINT('Ctrl Pts',(-10.3727493785979,-36.2742356128,-2.47593200036486));
#60083=CARTESIAN_POINT('Ctrl Pts',(-10.3904135773074,-36.2742356128,-2.38322042713068));
#60084=CARTESIAN_POINT('Ctrl Pts',(-10.398691197646,-36.2742356128,-2.33977485584547));
#60085=CARTESIAN_POINT('Ctrl Pts',(-10.4064831129282,-36.2742356128,-2.29626280366837));
#60086=CARTESIAN_POINT('Ctrl Pts',(-10.4137985541644,-36.2742356128,-2.25270313971161));
#60087=CARTESIAN_POINT('Ctrl Pts',(-10.430672018222,-36.2742356128,-2.15223039987303));
#60088=CARTESIAN_POINT('Ctrl Pts',(-10.4449859145385,-36.2742356121164,
-2.05149538873562));
#60089=CARTESIAN_POINT('Ctrl Pts',(-10.4569090914569,-36.2742356176125,
-1.95069270481178));
#60090=CARTESIAN_POINT('Ctrl Pts',(-10.4611862193506,-36.2742356195841,
-1.91453237823736));
#60091=CARTESIAN_POINT('Ctrl Pts',(-10.465156138689,-36.2742356223624,-1.87836308786589));
#60092=CARTESIAN_POINT('Ctrl Pts',(-10.4688279745932,-36.2742356259991,
-1.84219295236756));
#60093=CARTESIAN_POINT('Ctrl Pts',(-10.48024327157,-36.2742356373051,-1.7297443437734));
#60094=CARTESIAN_POINT('Ctrl Pts',(-10.4887947228398,-36.2742356503102,
-1.61726739875892));
#60095=CARTESIAN_POINT('Ctrl Pts',(-10.4947633362093,-36.2742356548179,
-1.50495659874232));
#60096=CARTESIAN_POINT('Ctrl Pts',(-10.5011033567854,-36.274235659606,-1.38565706651662));
#60097=CARTESIAN_POINT('Ctrl Pts',(-10.5045307178127,-36.2742356547264,
-1.26654556817452));
#60098=CARTESIAN_POINT('Ctrl Pts',(-10.5054136103061,-36.2742356439644,
-1.14780685036128));
#60099=CARTESIAN_POINT('Ctrl Pts',(-10.5057246075479,-36.2742356401736,
-1.10598135743335));
#60100=CARTESIAN_POINT('Ctrl Pts',(-10.5057200383727,-36.2742356357964,
-1.06420166036534));
#60101=CARTESIAN_POINT('Ctrl Pts',(-10.5054162157459,-36.2742356314567,
-1.02247432570434));
#60102=CARTESIAN_POINT('Ctrl Pts',(-10.5045830083842,-36.2742356195555,
-0.908040707645507));
#60103=CARTESIAN_POINT('Ctrl Pts',(-10.5014747563221,-36.2742356163105,
-0.79393675611565));
#60104=CARTESIAN_POINT('Ctrl Pts',(-10.496415029551,-36.2742356145671,-0.680268028397453));
#60105=CARTESIAN_POINT('Ctrl Pts',(-10.4917546355556,-36.2742356129613,
-0.575570466636018));
#60106=CARTESIAN_POINT('Ctrl Pts',(-10.4854396323409,-36.2742356129067,
-0.4712417088829));
#60107=CARTESIAN_POINT('Ctrl Pts',(-10.4776986870203,-36.2742356128358,
-0.367328990181301));
#60108=CARTESIAN_POINT('Ctrl Pts',(-10.4719656657543,-36.2742356127833,
-0.290370194909717));
#60109=CARTESIAN_POINT('Ctrl Pts',(-10.4654501123239,-36.2742356128,-0.21363890449008));
#60110=CARTESIAN_POINT('Ctrl Pts',(-10.4582308198287,-36.2742356128,-0.137142046369777));
#60111=CARTESIAN_POINT('Ctrl Pts',(-10.4493364654897,-36.2742356128,-0.0428959464369612));
#60112=CARTESIAN_POINT('Ctrl Pts',(-10.4393783264163,-36.2742356128,0.0509843559394398));
#60113=CARTESIAN_POINT('Ctrl Pts',(-10.4284676904419,-36.2742356128,0.14450999181293));
#60114=CARTESIAN_POINT('Ctrl Pts',(-10.4180812512127,-36.2742356128,0.233542229314824));
#60115=CARTESIAN_POINT('Ctrl Pts',(-10.4068319117135,-36.2742356128,0.322253206188292));
#60116=CARTESIAN_POINT('Ctrl Pts',(-10.3947746327428,-36.2742356128,0.41067344725918));
#60117=CARTESIAN_POINT('Ctrl Pts',(-10.3853531073324,-36.2742356128,0.479764786197444));
#60118=CARTESIAN_POINT('Ctrl Pts',(-10.3754375603691,-36.2742356128,0.548679007393723));
#60119=CARTESIAN_POINT('Ctrl Pts',(-10.3650337459782,-36.2742356128,0.617439519286842));
#60120=CARTESIAN_POINT('Ctrl Pts',(-10.3621231885442,-36.2742356128,0.636675869680322));
#60121=CARTESIAN_POINT('Ctrl Pts',(-10.3591742392757,-36.2742356128,0.655900638740825));
#60122=CARTESIAN_POINT('Ctrl Pts',(-10.3561866610074,-36.2742356128,0.675114926906024));
#60123=CARTESIAN_POINT('Ctrl Pts',(-10.3552979558047,-36.2742356128,0.680830538791121));
#60124=CARTESIAN_POINT('Ctrl Pts',(-10.3544061621333,-36.2742356128,0.686543110974668));
#60125=CARTESIAN_POINT('Ctrl Pts',(-10.3535104648,-36.2742356128,0.692257829523));
#60126=CARTESIAN_POINT('',(-5.5398869008,-36.2742356128,5.60697988192));
#60127=CARTESIAN_POINT('',(-2.46701990945003E-5,-36.2742356128,10.9643459861));
#60128=CARTESIAN_POINT('Ctrl Pts',(-5.5398869008,-36.2742356128,5.60697988192));
#60129=CARTESIAN_POINT('Ctrl Pts',(-5.5346953901423,-36.2742356128,5.76156714385257));
#60130=CARTESIAN_POINT('Ctrl Pts',(-5.52304547085452,-36.2742356128,5.91594818570587));
#60131=CARTESIAN_POINT('Ctrl Pts',(-5.50496486738705,-36.2742356128,6.06957376603556));
#60132=CARTESIAN_POINT('Ctrl Pts',(-5.48674534930841,-36.2742356128,6.22437966303974));
#60133=CARTESIAN_POINT('Ctrl Pts',(-5.46199605025368,-36.2742356128,6.37841824757372));
#60134=CARTESIAN_POINT('Ctrl Pts',(-5.43079794581926,-36.2742356128,6.53113717557828));
#60135=CARTESIAN_POINT('Ctrl Pts',(-5.3993756059117,-36.2742356128,6.68495376646011));
#60136=CARTESIAN_POINT('Ctrl Pts',(-5.36141153554192,-36.2742356128,6.83743145494455));
#60137=CARTESIAN_POINT('Ctrl Pts',(-5.31704005924504,-36.2742356128,6.98801872521846));
#60138=CARTESIAN_POINT('Ctrl Pts',(-5.27237815171884,-36.2742356128,7.13959165677023));
#60139=CARTESIAN_POINT('Ctrl Pts',(-5.22122480697047,-36.2742356128,7.28924912531629));
#60140=CARTESIAN_POINT('Ctrl Pts',(-5.16376732938617,-36.2742356128,7.43644486626614));
#60141=CARTESIAN_POINT('Ctrl Pts',(-5.10582843211048,-36.2742356128,7.58487391802533));
#60142=CARTESIAN_POINT('Ctrl Pts',(-5.04147943369501,-36.2742356128,7.73079958280341));
#60143=CARTESIAN_POINT('Ctrl Pts',(-4.97096161827184,-36.2742356128,7.87368154053936));
#60144=CARTESIAN_POINT('Ctrl Pts',(-4.90018282130001,-36.2742356128,8.01709229450049));
#60145=CARTESIAN_POINT('Ctrl Pts',(-4.82318962125999,-36.2742356128,8.15743654403781));
#60146=CARTESIAN_POINT('Ctrl Pts',(-4.7402732528861,-36.2742356128,8.29419125952485));
#60147=CARTESIAN_POINT('Ctrl Pts',(-4.6570241839819,-36.2742356128,8.43149470100239));
#60148=CARTESIAN_POINT('Ctrl Pts',(-4.56780448001639,-36.2742356128,8.56517951035103));
#60149=CARTESIAN_POINT('Ctrl Pts',(-4.47295403381865,-36.2742356128,8.69474326837329));
#60150=CARTESIAN_POINT('Ctrl Pts',(-4.41538891090186,-36.2742356128,8.77337604191411));
#60151=CARTESIAN_POINT('Ctrl Pts',(-4.35575066660558,-36.2742356128,8.85049143545389));
#60152=CARTESIAN_POINT('Ctrl Pts',(-4.29412294654456,-36.2742356128,8.92598250047464));
#60153=CARTESIAN_POINT('Ctrl Pts',(-4.19173460457658,-36.2742356128,9.05140341452465));
#60154=CARTESIAN_POINT('Ctrl Pts',(-4.0838526562137,-36.2742356128,9.17233904229695));
#60155=CARTESIAN_POINT('Ctrl Pts',(-3.97089095617117,-36.2742356128,9.28832809052255));
#60156=CARTESIAN_POINT('Ctrl Pts',(-3.85796902574901,-36.2742356128,9.40427630331089));
#60157=CARTESIAN_POINT('Ctrl Pts',(-3.73997114015286,-36.2742356128,9.51528119940368));
#60158=CARTESIAN_POINT('Ctrl Pts',(-3.61734836254789,-36.2742356128001,
9.62091792946744));
#60159=CARTESIAN_POINT('Ctrl Pts',(-3.49495417070753,-36.2742356128001,
9.72635773810123));
#60160=CARTESIAN_POINT('Ctrl Pts',(-3.36795254093104,-36.2742356128002,
9.8264491681409));
#60161=CARTESIAN_POINT('Ctrl Pts',(-3.23682616443467,-36.2742356128003,
9.92080875803141));
#60162=CARTESIAN_POINT('Ctrl Pts',(-3.10613251965052,-36.2742356128004,
10.0148569507188));
#60163=CARTESIAN_POINT('Ctrl Pts',(-2.9713415378996,-36.2742356128006,10.1032108784461));
#60164=CARTESIAN_POINT('Ctrl Pts',(-2.83296166688316,-36.2742356128007,
10.1855326471265));
#60165=CARTESIAN_POINT('Ctrl Pts',(-2.69559582751787,-36.2742356128008,
10.2672511714303));
#60166=CARTESIAN_POINT('Ctrl Pts',(-2.55469374396532,-36.2742356128009,
10.3430254623245));
#60167=CARTESIAN_POINT('Ctrl Pts',(-2.41077935977487,-36.2742356128009,
10.412568804815));
#60168=CARTESIAN_POINT('Ctrl Pts',(-2.26762762952295,-36.274235612801,10.481743612191));
#60169=CARTESIAN_POINT('Ctrl Pts',(-2.12149566208515,-36.274235612801,10.5447531729252));
#60170=CARTESIAN_POINT('Ctrl Pts',(-1.97292210274691,-36.2742356128009,
10.6013612096786));
#60171=CARTESIAN_POINT('Ctrl Pts',(-1.82570947854556,-36.2742356128008,
10.6574507163074));
#60172=CARTESIAN_POINT('Ctrl Pts',(-1.67610001053631,-36.2742356128007,
10.707255314709));
#60173=CARTESIAN_POINT('Ctrl Pts',(-1.52463698246422,-36.2742356128005,
10.7505924289492));
#60174=CARTESIAN_POINT('Ctrl Pts',(-1.44518898427323,-36.2742356128004,
10.7733243590946));
#60175=CARTESIAN_POINT('Ctrl Pts',(-1.36523130057623,-36.2742356128003,
10.7942776299538));
#60176=CARTESIAN_POINT('Ctrl Pts',(-1.28484418209153,-36.2742356128002,
10.8134313424015));
#60177=CARTESIAN_POINT('Ctrl Pts',(-1.13262152986081,-36.2742356128,10.8497011946341));
#60178=CARTESIAN_POINT('Ctrl Pts',(-0.978861102002178,-36.2742356128,10.8795144100532));
#60179=CARTESIAN_POINT('Ctrl Pts',(-0.82411483131256,-36.2742356128,10.9027686625403));
#60180=CARTESIAN_POINT('Ctrl Pts',(-0.671184727618257,-36.2742356128,10.9257499933881));
#60181=CARTESIAN_POINT('Ctrl Pts',(-0.517291966768855,-36.2742356128,10.9423253362505));
#60182=CARTESIAN_POINT('Ctrl Pts',(-0.362980351578935,-36.2742356128,10.9524454430755));
#60183=CARTESIAN_POINT('Ctrl Pts',(-0.272471115856985,-36.2742356128,10.9583812446873));
#60184=CARTESIAN_POINT('Ctrl Pts',(-0.181817979358742,-36.2742356128,10.9620972299496));
#60185=CARTESIAN_POINT('Ctrl Pts',(-0.0911321048928935,-36.2742356128,10.9635917110187));
#60186=CARTESIAN_POINT('Ctrl Pts',(-0.0660653661594743,-36.2742356128,10.9640048047526));
#60187=CARTESIAN_POINT('Ctrl Pts',(-0.0409957765907243,-36.2742356128,10.9642482065052));
#60188=CARTESIAN_POINT('Ctrl Pts',(-0.0159262763392949,-36.2742356128,10.9643219569687));
#60189=CARTESIAN_POINT('Ctrl Pts',(-0.0106256139653286,-36.2742356128,10.9643375506703));
#60190=CARTESIAN_POINT('Ctrl Pts',(-0.00532495008970526,-36.2742356128,
10.9643455597667));
#60191=CARTESIAN_POINT('Ctrl Pts',(-2.46701990951337E-5,-36.2742356128,
10.9643459861));
#60192=CARTESIAN_POINT('',(-4.67790704727252,-36.2742356128007,1.76602464761587));
#60193=CARTESIAN_POINT('Ctrl Pts',(-4.67800175527594,-36.2742356128,1.76632657424107));
#60194=CARTESIAN_POINT('Ctrl Pts',(-4.69198401483433,-36.2742356128,1.81130696346438));
#60195=CARTESIAN_POINT('Ctrl Pts',(-4.705344244229,-36.2742356128112,1.85562502943862));
#60196=CARTESIAN_POINT('Ctrl Pts',(-4.71832385294181,-36.2742356128199,
1.89944120814255));
#60197=CARTESIAN_POINT('Ctrl Pts',(-4.73151535902486,-36.2742356128287,
1.94397270371365));
#60198=CARTESIAN_POINT('Ctrl Pts',(-4.74431347042368,-36.2742356128363,
1.98798562464597));
#60199=CARTESIAN_POINT('Ctrl Pts',(-4.75692050655433,-36.2742356128616,
2.03162435033008));
#60200=CARTESIAN_POINT('Ctrl Pts',(-4.77000908213447,-36.2742356128878,
2.07692990457919));
#60201=CARTESIAN_POINT('Ctrl Pts',(-4.78289163080876,-36.2742356129249,
2.12183203129925));
#60202=CARTESIAN_POINT('Ctrl Pts',(-4.79574215657131,-36.2742356130778,
2.16646854508074));
#60203=CARTESIAN_POINT('Ctrl Pts',(-4.80705064219312,-36.2742356132124,
2.20574875692834));
#60204=CARTESIAN_POINT('Ctrl Pts',(-4.81833339247835,-36.2742356134291,
2.24482282251678));
#60205=CARTESIAN_POINT('Ctrl Pts',(-4.82967844196943,-36.2742356139743,
2.28377145245306));
#60206=CARTESIAN_POINT('Ctrl Pts',(-4.84309399664076,-36.2742356146189,
2.32982832286991));
#60207=CARTESIAN_POINT('Ctrl Pts',(-4.85663254045109,-36.2742356167299,
2.3758619561797));
#60208=CARTESIAN_POINT('Ctrl Pts',(-4.87035410558333,-36.2742356218589,
2.42180875135198));
#60209=CARTESIAN_POINT('Ctrl Pts',(-4.88114209308927,-36.2742356258913,
2.45793243312445));
#60210=CARTESIAN_POINT('Ctrl Pts',(-4.8920422151928,-36.274235631805,2.4940022482321));
#60211=CARTESIAN_POINT('Ctrl Pts',(-4.90306179734455,-36.2742356374317,
2.52998105296957));
#60212=CARTESIAN_POINT('Ctrl Pts',(-4.91857234662679,-36.2742356453514,
2.58062281200475));
#60213=CARTESIAN_POINT('Ctrl Pts',(-4.93433974729081,-36.274235650124,2.63113356670393));
#60214=CARTESIAN_POINT('Ctrl Pts',(-4.95040944020017,-36.2742356495911,
2.68169254618777));
#60215=CARTESIAN_POINT('Ctrl Pts',(-4.96027798559937,-36.2742356492639,
2.71274127793313));
#60216=CARTESIAN_POINT('Ctrl Pts',(-4.97025944992807,-36.2742356470856,
2.74380776889054));
#60217=CARTESIAN_POINT('Ctrl Pts',(-4.98035527463554,-36.2742356436435,
2.77493058470113));
#60218=CARTESIAN_POINT('Ctrl Pts',(-4.99775694492439,-36.2742356377105,
2.82857543243661));
#60219=CARTESIAN_POINT('Ctrl Pts',(-5.01549138037413,-36.2742356323325,
2.88238703379159));
#60220=CARTESIAN_POINT('Ctrl Pts',(-5.03348596356622,-36.27423562799,2.9364371383734));
#60221=CARTESIAN_POINT('Ctrl Pts',(-5.05350905181838,-36.2742356231581,
2.9965802382456));
#60222=CARTESIAN_POINT('Ctrl Pts',(-5.07385411249554,-36.2742356196165,
3.05701811984453));
#60223=CARTESIAN_POINT('Ctrl Pts',(-5.09435518995256,-36.2742356172974,
3.11783961754101));
#60224=CARTESIAN_POINT('Ctrl Pts',(-5.11697946350513,-36.2742356147382,
3.18496009960577));
#60225=CARTESIAN_POINT('Ctrl Pts',(-5.13979261948919,-36.2742356136397,
3.25254656888927));
#60226=CARTESIAN_POINT('Ctrl Pts',(-5.16250518657835,-36.2742356131765,
3.32072084496247));
#60227=CARTESIAN_POINT('Ctrl Pts',(-5.18560887764447,-36.2742356127054,
3.39006912280654));
#60228=CARTESIAN_POINT('Ctrl Pts',(-5.20860586975898,-36.2742356128,3.46002414789234));
#60229=CARTESIAN_POINT('Ctrl Pts',(-5.23115686865635,-36.2742356128,3.53073768416982));
#60230=CARTESIAN_POINT('Ctrl Pts',(-5.25137840927041,-36.2742356128,3.59414669998799));
#60231=CARTESIAN_POINT('Ctrl Pts',(-5.27126682535185,-36.2742356128,3.65823688138688));
#60232=CARTESIAN_POINT('Ctrl Pts',(-5.29057772872032,-36.2742356128,3.72303682547084));
#60233=CARTESIAN_POINT('Ctrl Pts',(-5.31043088538772,-36.2742356128,3.78965636249563));
#60234=CARTESIAN_POINT('Ctrl Pts',(-5.32967208410964,-36.2742356128,3.85702515017592));
#60235=CARTESIAN_POINT('Ctrl Pts',(-5.34803592730172,-36.2742356128,3.92511801119792));
#60236=CARTESIAN_POINT('Ctrl Pts',(-5.3656885232509,-36.2742356128,3.99057357788252));
#60237=CARTESIAN_POINT('Ctrl Pts',(-5.38252963521041,-36.2742356128,4.05669852810358));
#60238=CARTESIAN_POINT('Ctrl Pts',(-5.39834060086143,-36.2742356128,4.12342537331533));
#60239=CARTESIAN_POINT('Ctrl Pts',(-5.4140940065713,-36.2742356128,4.18990929893772));
#60240=CARTESIAN_POINT('Ctrl Pts',(-5.42882371242491,-36.2742356128,4.25699046577942));
#60241=CARTESIAN_POINT('Ctrl Pts',(-5.44234517887241,-36.2742356128,4.32455897862455));
#60242=CARTESIAN_POINT('Ctrl Pts',(-5.45153207351824,-36.2742356128,4.37046707678046));
#60243=CARTESIAN_POINT('Ctrl Pts',(-5.46016234726271,-36.2742356128,4.41660102851775));
#60244=CARTESIAN_POINT('Ctrl Pts',(-5.46819181711895,-36.2742356128,4.46292801882197));
#60245=CARTESIAN_POINT('Ctrl Pts',(-5.47904486691391,-36.2742356128,4.52554599256428));
#60246=CARTESIAN_POINT('Ctrl Pts',(-5.48879737839669,-36.2742356128,4.58851297281068));
#60247=CARTESIAN_POINT('Ctrl Pts',(-5.49737103594156,-36.2742356128,4.65170380600931));
#60248=CARTESIAN_POINT('Ctrl Pts',(-5.50560634546158,-36.2742356128,4.71240089677772));
#60249=CARTESIAN_POINT('Ctrl Pts',(-5.5127537305799,-36.2742356128,4.77330424861653));
#60250=CARTESIAN_POINT('Ctrl Pts',(-5.51878676668022,-36.2742356128,4.83428226178526));
#60251=CARTESIAN_POINT('Ctrl Pts',(-5.52234392131188,-36.2742356128,4.87023567203606));
#60252=CARTESIAN_POINT('Ctrl Pts',(-5.52551451797872,-36.2742356128,4.90621466424306));
#60253=CARTESIAN_POINT('Ctrl Pts',(-5.52830117031403,-36.2742356128,4.94218922880154));
#60254=CARTESIAN_POINT('Ctrl Pts',(-5.53276441084929,-36.2742356128,4.99980787492446));
#60255=CARTESIAN_POINT('Ctrl Pts',(-5.536241669784,-36.2742356128,5.05743511975529));
#60256=CARTESIAN_POINT('Ctrl Pts',(-5.53877783630915,-36.2742356128,5.11493113448532));
#60257=CARTESIAN_POINT('Ctrl Pts',(-5.54126560210858,-36.2742356128,5.17132988339643));
#60258=CARTESIAN_POINT('Ctrl Pts',(-5.542847624125,-36.2742356128,5.22760222608721));
#60259=CARTESIAN_POINT('Ctrl Pts',(-5.5436136967884,-36.2742356128,5.28360428844439));
#60260=CARTESIAN_POINT('Ctrl Pts',(-5.54435882909874,-36.2742356128,5.338075552206));
#60261=CARTESIAN_POINT('Ctrl Pts',(-5.54433190551395,-36.2742356128,5.39229097618915));
#60262=CARTESIAN_POINT('Ctrl Pts',(-5.54366316138914,-36.2742356128,5.4461087902728));
#60263=CARTESIAN_POINT('Ctrl Pts',(-5.54301952581734,-36.2742356128,5.49790596987407));
#60264=CARTESIAN_POINT('Ctrl Pts',(-5.54178138873351,-36.2742356128,5.54933471403915));
#60265=CARTESIAN_POINT('Ctrl Pts',(-5.54010996325318,-36.2742356128,5.60026168051131));
#60266=CARTESIAN_POINT('Ctrl Pts',(-5.54003643972157,-36.2742356128,5.60250188234686));
#60267=CARTESIAN_POINT('Ctrl Pts',(-5.53996208891191,-36.2742356128,5.60474108660317));
#60268=CARTESIAN_POINT('Ctrl Pts',(-5.5398869008,-36.2742356128,5.60697988192));
#60269=CARTESIAN_POINT('',(-0.665818988042834,-36.2742356128,-2.24488955640065));
#60270=CARTESIAN_POINT('Ctrl Pts',(-0.665819092629,-36.2742356128,-2.2448895341));
#60271=CARTESIAN_POINT('Ctrl Pts',(-0.737228677932033,-36.2742356128,-2.23017916472095));
#60272=CARTESIAN_POINT('Ctrl Pts',(-0.808566626719662,-36.2742356127611,
-2.21435533917569));
#60273=CARTESIAN_POINT('Ctrl Pts',(-0.879795665857112,-36.2742356129554,
-2.19738461926913));
#60274=CARTESIAN_POINT('Ctrl Pts',(-0.954705463597933,-36.2742356131597,
-2.17953693788649));
#60275=CARTESIAN_POINT('Ctrl Pts',(-1.02949530188753,-36.2742356136668,
-2.16041996465169));
#60276=CARTESIAN_POINT('Ctrl Pts',(-1.10409917953572,-36.2742356148821,
-2.1399379701008));
#60277=CARTESIAN_POINT('Ctrl Pts',(-1.18453540429552,-36.2742356161925,
-2.11785474374367));
#60278=CARTESIAN_POINT('Ctrl Pts',(-1.26475633734396,-36.2742356183635,
-2.09418353794173));
#60279=CARTESIAN_POINT('Ctrl Pts',(-1.34464241851358,-36.2742356213129,
-2.06875540131051));
#60280=CARTESIAN_POINT('Ctrl Pts',(-1.38843799632301,-36.2742356229299,
-2.05481505125108));
#60281=CARTESIAN_POINT('Ctrl Pts',(-1.43213222438249,-36.2742356247662,
-2.0403459268008));
#60282=CARTESIAN_POINT('Ctrl Pts',(-1.47569974337329,-36.2742356267012,
-2.02531691033586));
#60283=CARTESIAN_POINT('Ctrl Pts',(-1.54285372709818,-36.2742356296839,
-2.0021515258828));
#60284=CARTESIAN_POINT('Ctrl Pts',(-1.60972379741354,-36.2742356283408,
-1.97766308160781));
#60285=CARTESIAN_POINT('Ctrl Pts',(-1.67619838733452,-36.2742356240296,
-1.95173199462251));
#60286=CARTESIAN_POINT('Ctrl Pts',(-1.742672977254,-36.2742356197183,-1.9258009076378));
#60287=CARTESIAN_POINT('Ctrl Pts',(-1.80876937761299,-36.2742356150089,
-1.89841859520787));
#60288=CARTESIAN_POINT('Ctrl Pts',(-1.87430531806608,-36.2742356139044,
-1.86946353977244));
#60289=CARTESIAN_POINT('Ctrl Pts',(-1.94075639204582,-36.2742356127845,
-1.84010416051391));
#60290=CARTESIAN_POINT('Ctrl Pts',(-2.00662329644622,-36.2742356128485,
-1.80914041603183));
#60291=CARTESIAN_POINT('Ctrl Pts',(-2.07172628696219,-36.2742356128159,
-1.77648961183462));
#60292=CARTESIAN_POINT('Ctrl Pts',(-2.13502947445721,-36.2742356127841,
-1.74474145459058));
#60293=CARTESIAN_POINT('Ctrl Pts',(-2.19761044716111,-36.2742356128,-1.7113975703382));
#60294=CARTESIAN_POINT('Ctrl Pts',(-2.25927107931469,-36.2742356128,-1.67641596621023));
#60295=CARTESIAN_POINT('Ctrl Pts',(-2.32014698221066,-36.2742356128,-1.64187955843005));
#60296=CARTESIAN_POINT('Ctrl Pts',(-2.3801290898588,-36.2742356128,-1.60574174956389));
#60297=CARTESIAN_POINT('Ctrl Pts',(-2.43909548117802,-36.2742356128,-1.56799290777033));
#60298=CARTESIAN_POINT('Ctrl Pts',(-2.49915480898836,-36.2742356128,-1.52954439476116));
#60299=CARTESIAN_POINT('Ctrl Pts',(-2.55816012613216,-36.2742356128,-1.48942481668619));
#60300=CARTESIAN_POINT('Ctrl Pts',(-2.6159991563388,-36.2742356128,-1.44767594041806));
#60301=CARTESIAN_POINT('Ctrl Pts',(-2.67546098795818,-36.2742356128,-1.40475570745278));
#60302=CARTESIAN_POINT('Ctrl Pts',(-2.73368979290356,-36.2742356128,-1.36011369078322));
#60303=CARTESIAN_POINT('Ctrl Pts',(-2.79058610628415,-36.2742356128,-1.31384619761134));
#60304=CARTESIAN_POINT('Ctrl Pts',(-2.83586651357112,-36.2742356128,-1.2770246390517));
#60305=CARTESIAN_POINT('Ctrl Pts',(-2.88030335942422,-36.2742356128,-1.23917465391729));
#60306=CARTESIAN_POINT('Ctrl Pts',(-2.92385864229918,-36.2742356128,-1.20036514515414));
#60307=CARTESIAN_POINT('Ctrl Pts',(-2.95967700329097,-36.2742356128,-1.16844954495513));
#60308=CARTESIAN_POINT('Ctrl Pts',(-2.99489972169506,-36.2742356128,-1.13588523359943));
#60309=CARTESIAN_POINT('Ctrl Pts',(-3.02951901097885,-36.2742356128,-1.10271102209015));
#60310=CARTESIAN_POINT('Ctrl Pts',(-3.08321457923609,-36.2742356128,-1.05125681331438));
#60311=CARTESIAN_POINT('Ctrl Pts',(-3.13545017609485,-36.2742356128,-0.998339298681614));
#60312=CARTESIAN_POINT('Ctrl Pts',(-3.1861888002707,-36.2742356128,-0.944168555886378));
#60313=CARTESIAN_POINT('Ctrl Pts',(-3.21255606226399,-36.2742356128,-0.916017730142606));
#60314=CARTESIAN_POINT('Ctrl Pts',(-3.23851969999428,-36.2742356128,-0.887529050260996));
#60315=CARTESIAN_POINT('Ctrl Pts',(-3.26407891862252,-36.2742356128,-0.858735372798419));
#60316=CARTESIAN_POINT('Ctrl Pts',(-3.30671952622392,-36.2742356128,-0.810698696875676));
#60317=CARTESIAN_POINT('Ctrl Pts',(-3.3482422594108,-36.2742356127889,-0.761808566534635));
#60318=CARTESIAN_POINT('Ctrl Pts',(-3.38869992815495,-36.2742356128111,
-0.712264459872021));
#60319=CARTESIAN_POINT('Ctrl Pts',(-3.39362145153746,-36.2742356128137,
-0.706237605459142));
#60320=CARTESIAN_POINT('Ctrl Pts',(-3.39852723137462,-36.2742356128172,
-0.700201012931191));
#60321=CARTESIAN_POINT('Ctrl Pts',(-3.40341737611036,-36.274235612822,-0.694154991753613));
#60322=CARTESIAN_POINT('Ctrl Pts',(-3.44454477977108,-36.2742356128622,
-0.643306363144609));
#60323=CARTESIAN_POINT('Ctrl Pts',(-3.48454420070821,-36.2742356122796,
-0.591773595290768));
#60324=CARTESIAN_POINT('Ctrl Pts',(-3.52350036363258,-36.2742356262016,
-0.539735571971687));
#60325=CARTESIAN_POINT('Ctrl Pts',(-3.52725363315677,-36.2742356275429,
-0.534721917844568));
#60326=CARTESIAN_POINT('Ctrl Pts',(-3.5309972277434,-36.2742356290141,-0.529703535081257));
#60327=CARTESIAN_POINT('Ctrl Pts',(-3.53473122853353,-36.2742356306207,
-0.524680559427204));
#60328=CARTESIAN_POINT('Ctrl Pts',(-3.57694501547953,-36.2742356487836,
-0.467894598198846));
#60329=CARTESIAN_POINT('Ctrl Pts',(-3.61794060915933,-36.2742356874614,
-0.410522390412449));
#60330=CARTESIAN_POINT('Ctrl Pts',(-3.65782801944055,-36.2742357136805,
-0.352746823971276));
#60331=CARTESIAN_POINT('Ctrl Pts',(-3.69771542972177,-36.2742357398996,
-0.294971257530103));
#60332=CARTESIAN_POINT('Ctrl Pts',(-3.73649023726764,-36.2742357474187,
-0.236799307450452));
#60333=CARTESIAN_POINT('Ctrl Pts',(-3.77426745301402,-36.274235735014,-0.178287757725677));
#60334=CARTESIAN_POINT('Ctrl Pts',(-3.81489213576152,-36.2742357216743,
-0.115365885436529));
#60335=CARTESIAN_POINT('Ctrl Pts',(-3.85436208782408,-36.2742356989606,
-0.0520319711964369));
#60336=CARTESIAN_POINT('Ctrl Pts',(-3.89277713141461,-36.2742356785138,
0.0116646972747143));
#60337=CARTESIAN_POINT('Ctrl Pts',(-3.93133559414501,-36.2742356579906,
0.0755991715779432));
#60338=CARTESIAN_POINT('Ctrl Pts',(-3.96883222655404,-36.2742356401906,
0.139900037745291));
#60339=CARTESIAN_POINT('Ctrl Pts',(-4.00533748203647,-36.2742356294551,
0.204560244972189));
#60340=CARTESIAN_POINT('Ctrl Pts',(-4.04068199553069,-36.2742356190609,
0.2671644792576));
#60341=CARTESIAN_POINT('Ctrl Pts',(-4.07509781584091,-36.274235614972,0.330106576768051));
#60342=CARTESIAN_POINT('Ctrl Pts',(-4.10860887549533,-36.2742356136137,
0.393405625592747));
#60343=CARTESIAN_POINT('Ctrl Pts',(-4.1336476948815,-36.2742356125987,0.440701457690656));
#60344=CARTESIAN_POINT('Ctrl Pts',(-4.15818066405112,-36.2742356128,0.488197154084093));
#60345=CARTESIAN_POINT('Ctrl Pts',(-4.18219924647829,-36.2742356128,0.535905566233154));
#60346=CARTESIAN_POINT('Ctrl Pts',(-4.21266801474939,-36.2742356128,0.596426063592234));
#60347=CARTESIAN_POINT('Ctrl Pts',(-4.24232577357362,-36.2742356128,0.657296560446234));
#60348=CARTESIAN_POINT('Ctrl Pts',(-4.27120625360895,-36.2742356128,0.718566923232716));
#60349=CARTESIAN_POINT('Ctrl Pts',(-4.30008673365087,-36.2742356128,0.779837286033185));
#60350=CARTESIAN_POINT('Ctrl Pts',(-4.32819338159656,-36.2742356128,0.841515222100351));
#60351=CARTESIAN_POINT('Ctrl Pts',(-4.35553865680325,-36.2742356128,0.903617154925355));
#60352=CARTESIAN_POINT('Ctrl Pts',(-4.38898012358046,-36.2742356128,0.979563720014614));
#60353=CARTESIAN_POINT('Ctrl Pts',(-4.42129069411876,-36.2742356128,1.05616247724551));
#60354=CARTESIAN_POINT('Ctrl Pts',(-4.45246773012636,-36.2742356128001,
1.13340427103704));
#60355=CARTESIAN_POINT('Ctrl Pts',(-4.48679159733215,-36.2742356128001,
1.21844240847226));
#60356=CARTESIAN_POINT('Ctrl Pts',(-4.51974041626447,-36.2742356128003,
1.30425926912065));
#60357=CARTESIAN_POINT('Ctrl Pts',(-4.5512834584953,-36.2742356128004,1.39077904393112));
#60358=CARTESIAN_POINT('Ctrl Pts',(-4.58913299486063,-36.2742356128005,
1.49459697433378));
#60359=CARTESIAN_POINT('Ctrl Pts',(-4.62495504282474,-36.2742356128003,
1.59942531003409));
#60360=CARTESIAN_POINT('Ctrl Pts',(-4.6586950898368,-36.2742356128001,1.70506228796727));
#60361=CARTESIAN_POINT('Ctrl Pts',(-4.664047403989,-36.2742356128,1.72181989034363));
#60362=CARTESIAN_POINT('Ctrl Pts',(-4.66934739557618,-36.2742356128,1.73859776216507));
#60363=CARTESIAN_POINT('Ctrl Pts',(-4.67459495121429,-36.2742356128,1.7553950339094));
#60364=CARTESIAN_POINT('Ctrl Pts',(-4.67570152189309,-36.2742356128,1.75893713420865));
#60365=CARTESIAN_POINT('Ctrl Pts',(-4.67680559494956,-36.2742356128,1.76247955985014));
#60366=CARTESIAN_POINT('Ctrl Pts',(-4.67790780735,-36.2742356128,1.7660244085));
#60367=CARTESIAN_POINT('',(0.665819005986112,-36.2742356128,-2.24488955701597));
#60368=CARTESIAN_POINT('Origin',(0.000212348057480882,-36.2742356128,0.227537950203741));
#60369=CARTESIAN_POINT('',(4.67794129913,-36.2742356128,1.76613211329));
#60370=CARTESIAN_POINT('Ctrl Pts',(4.67793839402,-36.2742356128,1.76612278889));
#60371=CARTESIAN_POINT('Ctrl Pts',(4.6548471491261,-36.2742356128,1.69186544974786));
#60372=CARTESIAN_POINT('Ctrl Pts',(4.6307323914171,-36.2742356128003,1.61797566847106));
#60373=CARTESIAN_POINT('Ctrl Pts',(4.6056194961289,-36.2742356128003,1.54456189260851));
#60374=CARTESIAN_POINT('Ctrl Pts',(4.57962597242507,-36.2742356128003,1.46857373189777));
#60375=CARTESIAN_POINT('Ctrl Pts',(4.55256322090791,-36.2742356128002,1.39309516362647));
#60376=CARTESIAN_POINT('Ctrl Pts',(4.52444922260764,-36.2742356128002,1.31818980649636));
#60377=CARTESIAN_POINT('Ctrl Pts',(4.49451631237348,-36.2742356128001,1.23843824262817));
#60378=CARTESIAN_POINT('Ctrl Pts',(4.46339198392542,-36.2742356128,1.15933612320618));
#60379=CARTESIAN_POINT('Ctrl Pts',(4.43108342262081,-36.2742356128,1.0809023888135));
#60380=CARTESIAN_POINT('Ctrl Pts',(4.41927317708614,-36.2742356128,1.05223129904735));
#60381=CARTESIAN_POINT('Ctrl Pts',(4.40730453730176,-36.2742356128,1.02364901856025));
#60382=CARTESIAN_POINT('Ctrl Pts',(4.39517730788851,-36.2742356128,0.995154883908435));
#60383=CARTESIAN_POINT('Ctrl Pts',(4.35794106844874,-36.2742356128,0.907664626705557));
#60384=CARTESIAN_POINT('Ctrl Pts',(4.31921781659372,-36.2742356128,0.821022734370667));
#60385=CARTESIAN_POINT('Ctrl Pts',(4.27898363757762,-36.2742356128,0.735169479465547));
#60386=CARTESIAN_POINT('Ctrl Pts',(4.2608748946734,-36.2742356128,0.696528340051589));
#60387=CARTESIAN_POINT('Ctrl Pts',(4.24246006787135,-36.2742356128,0.658047080571516));
#60388=CARTESIAN_POINT('Ctrl Pts',(4.22373377331199,-36.2742356128,0.619715222891086));
#60389=CARTESIAN_POINT('Ctrl Pts',(4.17632752669855,-36.2742356128,0.522676831628486));
#60390=CARTESIAN_POINT('Ctrl Pts',(4.12690751722882,-36.2742356128,0.426554009358753));
#60391=CARTESIAN_POINT('Ctrl Pts',(4.07538515541344,-36.2742356128,0.331241273540381));
#60392=CARTESIAN_POINT('Ctrl Pts',(4.06339888726419,-36.2742356128,0.309067522778492));
#60393=CARTESIAN_POINT('Ctrl Pts',(4.05129861740903,-36.2742356128,0.286937563794092));
#60394=CARTESIAN_POINT('Ctrl Pts',(4.03908282686399,-36.2742356128,0.264850055636609));
#60395=CARTESIAN_POINT('Ctrl Pts',(4.00554454927516,-36.2742356128,0.204209119047194));
#60396=CARTESIAN_POINT('Ctrl Pts',(3.97113537519678,-36.2742356126953,0.143887166400186));
#60397=CARTESIAN_POINT('Ctrl Pts',(3.93582787419494,-36.2742356130921,0.0838826972028474));
#60398=CARTESIAN_POINT('Ctrl Pts',(3.90185603841753,-36.2742356134739,0.0261481672689329));
#60399=CARTESIAN_POINT('Ctrl Pts',(3.86705131020918,-36.2742356143011,-0.0312931655954265));
#60400=CARTESIAN_POINT('Ctrl Pts',(3.83134932336719,-36.2742356174484,-0.0884208183885626));
#60401=CARTESIAN_POINT('Ctrl Pts',(3.79481499520452,-36.2742356206691,-0.146880321596174));
#60402=CARTESIAN_POINT('Ctrl Pts',(3.75734127373668,-36.2742356252224,-0.20502580031905));
#60403=CARTESIAN_POINT('Ctrl Pts',(3.71883255615869,-36.274235626969,-0.262808961349773));
#60404=CARTESIAN_POINT('Ctrl Pts',(3.68059893653406,-36.2742356287032,-0.320179331969947));
#60405=CARTESIAN_POINT('Ctrl Pts',(3.64134406340379,-36.2742356268112,-0.377193377062157));
#60406=CARTESIAN_POINT('Ctrl Pts',(3.60096083749056,-36.2742356218413,-0.433754819684179));
#60407=CARTESIAN_POINT('Ctrl Pts',(3.563485510393,-36.2742356172293,-0.486243409078299));
#60408=CARTESIAN_POINT('Ctrl Pts',(3.52503334401459,-36.2742356149048,-0.538321086354601));
#60409=CARTESIAN_POINT('Ctrl Pts',(3.48552085288005,-36.2742356138311,-0.589851613583241));
#60410=CARTESIAN_POINT('Ctrl Pts',(3.44795857840759,-36.2742356128104,-0.638838750356814));
#60411=CARTESIAN_POINT('Ctrl Pts',(3.40943757352298,-36.2742356128121,-0.687331515184078));
#60412=CARTESIAN_POINT('Ctrl Pts',(3.36989713281383,-36.2742356128019,-0.735166458595873));
#60413=CARTESIAN_POINT('Ctrl Pts',(3.36032902804291,-36.2742356127994,-0.746741689980915));
#60414=CARTESIAN_POINT('Ctrl Pts',(3.35070130074832,-36.2742356128,-0.75827817578659));
#60415=CARTESIAN_POINT('Ctrl Pts',(3.34101324167528,-36.2742356128,-0.769773154095528));
#60416=CARTESIAN_POINT('Ctrl Pts',(3.29526352088457,-36.2742356128,-0.824055652185619));
#60417=CARTESIAN_POINT('Ctrl Pts',(3.24815560232718,-36.2742356128,-0.877433457315812));
#60418=CARTESIAN_POINT('Ctrl Pts',(3.19967614454946,-36.2742356128,-0.929673275944785));
#60419=CARTESIAN_POINT('Ctrl Pts',(3.15240628788772,-36.2742356128,-0.980609669457032));
#60420=CARTESIAN_POINT('Ctrl Pts',(3.10383269162824,-36.2742356128,-1.03046421061228));
#60421=CARTESIAN_POINT('Ctrl Pts',(3.05397476891398,-36.2742356128,-1.07905634490027));
#60422=CARTESIAN_POINT('Ctrl Pts',(3.00183115446817,-36.2742356128,-1.12987614198513));
#60423=CARTESIAN_POINT('Ctrl Pts',(2.94827976440738,-36.2742356128,-1.17931792987394));
#60424=CARTESIAN_POINT('Ctrl Pts',(2.89336456309009,-36.2742356128,-1.22722756870653));
#60425=CARTESIAN_POINT('Ctrl Pts',(2.83863179705281,-36.2742356128,-1.27497804562829));
#60426=CARTESIAN_POINT('Ctrl Pts',(2.78254459846684,-36.2742356128,-1.32120629344724));
#60427=CARTESIAN_POINT('Ctrl Pts',(2.72517907321423,-36.2742356128,-1.36580058859031));
#60428=CARTESIAN_POINT('Ctrl Pts',(2.66752673177032,-36.2742356128,-1.4106178463199));
#60429=CARTESIAN_POINT('Ctrl Pts',(2.60858331698472,-36.2742356128,-1.45378468187809));
#60430=CARTESIAN_POINT('Ctrl Pts',(2.54845707550452,-36.2742356128,-1.49523068468984));
#60431=CARTESIAN_POINT('Ctrl Pts',(2.48833083402433,-36.2742356128,-1.5366766875016));
#60432=CARTESIAN_POINT('Ctrl Pts',(2.42702185855343,-36.2742356128,-1.57640180073771));
#60433=CARTESIAN_POINT('Ctrl Pts',(2.36466806519104,-36.2742356128,-1.61437955209257));
#60434=CARTESIAN_POINT('Ctrl Pts',(2.30285964294221,-36.2742356128,-1.65202513490675));
#60435=CARTESIAN_POINT('Ctrl Pts',(2.24001695357672,-36.2742356128,-1.68795837080037));
#60436=CARTESIAN_POINT('Ctrl Pts',(2.17630747177397,-36.2742356128,-1.72219266457153));
#60437=CARTESIAN_POINT('Ctrl Pts',(2.11259798997122,-36.2742356128,-1.75642695834268));
#60438=CARTESIAN_POINT('Ctrl Pts',(2.04802182342419,-36.2742356128,-1.78896225437204));
#60439=CARTESIAN_POINT('Ctrl Pts',(1.98277319980503,-36.2742356128,-1.81985743232702));
#60440=CARTESIAN_POINT('Ctrl Pts',(1.91752074047581,-36.2742356128,-1.85075442648805));
#60441=CARTESIAN_POINT('Ctrl Pts',(1.85157764819585,-36.2742356126615,-1.88002487306571));
#60442=CARTESIAN_POINT('Ctrl Pts',(1.78516561446401,-36.2742356129385,-1.90775210033866));
#60443=CARTESIAN_POINT('Ctrl Pts',(1.71875358073217,-36.2742356132154,-1.93547932761161));
#60444=CARTESIAN_POINT('Ctrl Pts',(1.6518693341746,-36.2742356144321,-1.96167041142089));
#60445=CARTESIAN_POINT('Ctrl Pts',(1.58464405915673,-36.2742356155218,-1.98645717948924));
#60446=CARTESIAN_POINT('Ctrl Pts',(1.50771176789187,-36.274235616769,-2.01482304128813));
#60447=CARTESIAN_POINT('Ctrl Pts',(1.43032073812522,-36.2742356171986,-2.04135449475494));
#60448=CARTESIAN_POINT('Ctrl Pts',(1.35262135824679,-36.2742356167949,-2.06621671682666));
#60449=CARTESIAN_POINT('Ctrl Pts',(1.27282710612553,-36.2742356163803,-2.09174925543107));
#60450=CARTESIAN_POINT('Ctrl Pts',(1.19270675788403,-36.2742356152832,-2.11552252631164));
#60451=CARTESIAN_POINT('Ctrl Pts',(1.11236951057882,-36.2742356144497,-2.13769695919322));
#60452=CARTESIAN_POINT('Ctrl Pts',(1.03319649335471,-36.2742356136283,-2.15955004497047));
#60453=CARTESIAN_POINT('Ctrl Pts',(0.953811601705358,-36.2742356131035,
-2.17985130581748));
#60454=CARTESIAN_POINT('Ctrl Pts',(0.874284313879753,-36.2742356129234,
-2.19872032066919));
#60455=CARTESIAN_POINT('Ctrl Pts',(0.809363582982145,-36.2742356127764,
-2.2141237157677));
#60456=CARTESIAN_POINT('Ctrl Pts',(0.74434705187334,-36.2742356128,-2.22857228708359));
#60457=CARTESIAN_POINT('Ctrl Pts',(0.679263141868309,-36.2742356128,-2.24210692825591));
#60458=CARTESIAN_POINT('Ctrl Pts',(0.674782103646385,-36.2742356128,-2.24303879059191));
#60459=CARTESIAN_POINT('Ctrl Pts',(0.670301885654333,-36.2742356128,-2.24396609231333));
#60460=CARTESIAN_POINT('Ctrl Pts',(0.665819006916,-36.2742356128,-2.24488956153));
#60461=CARTESIAN_POINT('',(5.53988691730504,-36.2742356128,5.60697933185575));
#60462=CARTESIAN_POINT('Ctrl Pts',(5.53988692237398,-36.2742356128,5.60697918091797));
#60463=CARTESIAN_POINT('Ctrl Pts',(5.54165830493023,-36.2742356128,5.55423263886826));
#60464=CARTESIAN_POINT('Ctrl Pts',(5.5429724375768,-36.2742356128,5.50093679546234));
#60465=CARTESIAN_POINT('Ctrl Pts',(5.54364945845749,-36.2742356128,5.44724531226854));
#60466=CARTESIAN_POINT('Ctrl Pts',(5.54433722472412,-36.2742356128,5.39270166081026));
#60467=CARTESIAN_POINT('Ctrl Pts',(5.54436767013136,-36.2742356128,5.337749782334));
#60468=CARTESIAN_POINT('Ctrl Pts',(5.54360552907939,-36.2742356128,5.282539087133));
#60469=CARTESIAN_POINT('Ctrl Pts',(5.54282290024159,-36.2742356128,5.22584422453863));
#60470=CARTESIAN_POINT('Ctrl Pts',(5.54120462781002,-36.2742356128,5.16887654624831));
#60471=CARTESIAN_POINT('Ctrl Pts',(5.53865781012939,-36.2742356128,5.11178424092544));
#60472=CARTESIAN_POINT('Ctrl Pts',(5.53745660746727,-36.2742356128,5.08485674247821));
#60473=CARTESIAN_POINT('Ctrl Pts',(5.53604959570276,-36.2742356128,5.05790131769372));
#60474=CARTESIAN_POINT('Ctrl Pts',(5.53443085180288,-36.2742356128,5.03093240776099));
#60475=CARTESIAN_POINT('Ctrl Pts',(5.5308382665806,-36.2742356128,4.97107852519674));
#60476=CARTESIAN_POINT('Ctrl Pts',(5.52619836949679,-36.2742356128,4.9111422095337));
#60477=CARTESIAN_POINT('Ctrl Pts',(5.52048353574769,-36.2742356128,4.85126756067043));
#60478=CARTESIAN_POINT('Ctrl Pts',(5.51460523213774,-36.2742356128,4.78968022847327));
#60479=CARTESIAN_POINT('Ctrl Pts',(5.50758989745033,-36.2742356128,4.72815829258806));
#60480=CARTESIAN_POINT('Ctrl Pts',(5.49946006720242,-36.2742356128,4.66683869085727));
#60481=CARTESIAN_POINT('Ctrl Pts',(5.49106651547459,-36.2742356128,4.60352995828077));
#60482=CARTESIAN_POINT('Ctrl Pts',(5.48148534744977,-36.2742356128,4.5404370884034));
#60483=CARTESIAN_POINT('Ctrl Pts',(5.47079175011765,-36.2742356128,4.47768722295259));
#60484=CARTESIAN_POINT('Ctrl Pts',(5.46138568923118,-36.2742356128,4.42249260165565));
#60485=CARTESIAN_POINT('Ctrl Pts',(5.45111955899517,-36.2742356128,4.36755995871729));
#60486=CARTESIAN_POINT('Ctrl Pts',(5.44006866845322,-36.2742356128,4.31295000014857));
#60487=CARTESIAN_POINT('Ctrl Pts',(5.42645679487174,-36.2742356128,4.245684484351));
#60488=CARTESIAN_POINT('Ctrl Pts',(5.41165453195185,-36.2742356128,4.17891441274785));
#60489=CARTESIAN_POINT('Ctrl Pts',(5.39584673414317,-36.2742356128,4.11274168517014));
#60490=CARTESIAN_POINT('Ctrl Pts',(5.37930929780952,-36.2742356128,4.04351463137146));
#60491=CARTESIAN_POINT('Ctrl Pts',(5.36167225848251,-36.2742356128,3.97494176650156));
#60492=CARTESIAN_POINT('Ctrl Pts',(5.34318328727252,-36.2742356128,3.907096637803));
#60493=CARTESIAN_POINT('Ctrl Pts',(5.34002882901784,-36.2742356128,3.89552137902669));
#60494=CARTESIAN_POINT('Ctrl Pts',(5.33684963359364,-36.2742356128,3.8839671975358));
#60495=CARTESIAN_POINT('Ctrl Pts',(5.33364699796188,-36.2742356128,3.87243432667238));
#60496=CARTESIAN_POINT('Ctrl Pts',(5.31440651792086,-36.2742356128,3.80314827693791));
#60497=CARTESIAN_POINT('Ctrl Pts',(5.29431680957279,-36.2742356128,3.73462645497715));
#60498=CARTESIAN_POINT('Ctrl Pts',(5.27366540454653,-36.2742356128,3.66689041569989));
#60499=CARTESIAN_POINT('Ctrl Pts',(5.26699976162205,-36.2742356128,3.64502729063082));
#60500=CARTESIAN_POINT('Ctrl Pts',(5.2602756459931,-36.2742356128,3.62324562548497));
#60501=CARTESIAN_POINT('Ctrl Pts',(5.25350273274586,-36.2742356128,3.60154498249611));
#60502=CARTESIAN_POINT('Ctrl Pts',(5.23084294007848,-36.2742356128,3.52894224082113));
#60503=CARTESIAN_POINT('Ctrl Pts',(5.20764098851541,-36.2742356128,3.45725487651199));
#60504=CARTESIAN_POINT('Ctrl Pts',(5.18422503958467,-36.2742356128,3.38623266017563));
#60505=CARTESIAN_POINT('Ctrl Pts',(5.17895808821716,-36.2742356128,3.37025762706625));
#60506=CARTESIAN_POINT('Ctrl Pts',(5.17368029169311,-36.2742356128,3.35431645791937));
#60507=CARTESIAN_POINT('Ctrl Pts',(5.16839529949842,-36.2742356128,3.33840663348512));
#60508=CARTESIAN_POINT('Ctrl Pts',(5.14673287022256,-36.2742356128,3.27319453214193));
#60509=CARTESIAN_POINT('Ctrl Pts',(5.12495264363142,-36.2742356125143,3.20855115611014));
#60510=CARTESIAN_POINT('Ctrl Pts',(5.10330747750946,-36.2742356145159,3.1443462134388));
#60511=CARTESIAN_POINT('Ctrl Pts',(5.08348665088416,-36.2742356163488,3.08555271515814));
#60512=CARTESIAN_POINT('Ctrl Pts',(5.06377991216152,-36.2742356205018,3.02712777923992));
#60513=CARTESIAN_POINT('Ctrl Pts',(5.04434337184934,-36.2742356265321,2.96897470189817));
#60514=CARTESIAN_POINT('Ctrl Pts',(5.02611549217322,-36.2742356321874,2.91443787180618));
#60515=CARTESIAN_POINT('Ctrl Pts',(5.0081257568683,-36.2742356393532,2.86014068095253));
#60516=CARTESIAN_POINT('Ctrl Pts',(4.99045886252433,-36.2742356442228,2.80599669724385));
#60517=CARTESIAN_POINT('Ctrl Pts',(4.97397667379101,-36.2742356487659,2.75548349775978));
#60518=CARTESIAN_POINT('Ctrl Pts',(4.95777566188676,-36.2742356509722,2.70510395407236));
#60519=CARTESIAN_POINT('Ctrl Pts',(4.94188051554086,-36.274235648232,2.65477619342767));
#60520=CARTESIAN_POINT('Ctrl Pts',(4.93489101734184,-36.274235647027,2.63264580313543));
#60521=CARTESIAN_POINT('Ctrl Pts',(4.92796004742607,-36.2742356449018,2.610525240921));
#60522=CARTESIAN_POINT('Ctrl Pts',(4.92108659841074,-36.2742356419742,2.58840653662621));
#60523=CARTESIAN_POINT('Ctrl Pts',(4.90838833654212,-36.2742356365656,2.54754363087059));
#60524=CARTESIAN_POINT('Ctrl Pts',(4.89587110254343,-36.2742356286996,2.50663414959663));
#60525=CARTESIAN_POINT('Ctrl Pts',(4.88349086308502,-36.2742356228979,2.46557954036258));
#60526=CARTESIAN_POINT('Ctrl Pts',(4.87111062362242,-36.2742356170962,2.42452493111463));
#60527=CARTESIAN_POINT('Ctrl Pts',(4.85888611536352,-36.2742356144804,2.38339106874945));
#60528=CARTESIAN_POINT('Ctrl Pts',(4.84678270416545,-36.2742356139505,2.34224859775519));
#60529=CARTESIAN_POINT('Ctrl Pts',(4.83364239888552,-36.2742356133753,2.29758146879557));
#60530=CARTESIAN_POINT('Ctrl Pts',(4.82064635349563,-36.2742356131413,2.25284307171249));
#60531=CARTESIAN_POINT('Ctrl Pts',(4.80767077257532,-36.2742356130048,2.20789713737373));
#60532=CARTESIAN_POINT('Ctrl Pts',(4.79507702413614,-36.2742356128723,2.16427382725746));
#60533=CARTESIAN_POINT('Ctrl Pts',(4.78250272372987,-36.2742356128384,2.1204551903821));
#60534=CARTESIAN_POINT('Ctrl Pts',(4.76979178214926,-36.2742356128196,2.07629693005267));
#60535=CARTESIAN_POINT('Ctrl Pts',(4.75743128237245,-36.2742356128014,2.03335611693627));
#60536=CARTESIAN_POINT('Ctrl Pts',(4.74494177342037,-36.2742356128013,1.99009431956366));
#60537=CARTESIAN_POINT('Ctrl Pts',(4.73213582539401,-36.2742356128005,1.94635742420483));
#60538=CARTESIAN_POINT('Ctrl Pts',(4.71981950552344,-36.2742356127997,1.90429278422065));
#60539=CARTESIAN_POINT('Ctrl Pts',(4.70721060716778,-36.2742356128,1.86178879696953));
#60540=CARTESIAN_POINT('Ctrl Pts',(4.69409898682122,-36.2742356128,1.81868627934494));
#60541=CARTESIAN_POINT('Ctrl Pts',(4.69152954119736,-36.2742356128,1.81023960590866));
#60542=CARTESIAN_POINT('Ctrl Pts',(4.68894064748119,-36.2742356128,1.80176987349512));
#60543=CARTESIAN_POINT('Ctrl Pts',(4.68633051117043,-36.2742356128,1.79327577326918));
#60544=CARTESIAN_POINT('Ctrl Pts',(4.68355698486512,-36.2742356128,1.78424995713865));
#60545=CARTESIAN_POINT('Ctrl Pts',(4.68076549196667,-36.2742356128,1.77521613159));
#60546=CARTESIAN_POINT('Ctrl Pts',(4.67794710935,-36.2742356128,1.76615076209));
#60547=CARTESIAN_POINT('Ctrl Pts',(2.32481332798E-5,-36.2742356128,10.9643459795));
#60548=CARTESIAN_POINT('Ctrl Pts',(0.012267597991931,-36.2742356128,10.9643448993192));
#60549=CARTESIAN_POINT('Ctrl Pts',(0.0244497673928545,-36.2742356128,10.9643037788664));
#60550=CARTESIAN_POINT('Ctrl Pts',(0.0366626829731096,-36.2742356128,10.9642222827207));
#60551=CARTESIAN_POINT('Ctrl Pts',(0.190945660670054,-36.2742356128,10.9631927604951));
#60552=CARTESIAN_POINT('Ctrl Pts',(0.345196887448164,-36.2742356128,10.955732938611));
#60553=CARTESIAN_POINT('Ctrl Pts',(0.498871345331836,-36.2742356128,10.9418556346228));
#60554=CARTESIAN_POINT('Ctrl Pts',(0.654951435072277,-36.2742356128,10.927761094244));
#60555=CARTESIAN_POINT('Ctrl Pts',(0.810436383027939,-36.2742356128,10.9070466255314));
#60556=CARTESIAN_POINT('Ctrl Pts',(0.964764670252676,-36.2742356128,10.8797788422672));
#60557=CARTESIAN_POINT('Ctrl Pts',(1.11914274361821,-36.2742356128,10.8525022624451));
#60558=CARTESIAN_POINT('Ctrl Pts',(1.27236128250835,-36.2742356128,10.8186685334414));
#60559=CARTESIAN_POINT('Ctrl Pts',(1.42386599695573,-36.2742356128,10.7783972802877));
#60560=CARTESIAN_POINT('Ctrl Pts',(1.57654467229091,-36.2742356128,10.7378139782563));
#60561=CARTESIAN_POINT('Ctrl Pts',(1.72748264701554,-36.2742356128,10.6906931305989));
#60562=CARTESIAN_POINT('Ctrl Pts',(1.87612834575455,-36.2742356128,10.6372081072336));
#60563=CARTESIAN_POINT('Ctrl Pts',(2.02581869224373,-36.2742356128,10.5833472034372));
#60564=CARTESIAN_POINT('Ctrl Pts',(2.17318420757732,-36.2742356128,10.5230325024168));
#60565=CARTESIAN_POINT('Ctrl Pts',(2.31768076387948,-36.2742356128,10.4564904323508));
#60566=CARTESIAN_POINT('Ctrl Pts',(2.46348798666278,-36.2742356128,10.389344787618));
#60567=CARTESIAN_POINT('Ctrl Pts',(2.60637372464546,-36.2742356128,10.3158584289551));
#60568=CARTESIAN_POINT('Ctrl Pts',(2.74580189015219,-36.2742356128,10.2363119782628));
#60569=CARTESIAN_POINT('Ctrl Pts',(2.88575737001097,-36.2742356128,10.1564646845884));
#60570=CARTESIAN_POINT('Ctrl Pts',(3.02222884358078,-36.2742356128,10.0705115620573));
#60571=CARTESIAN_POINT('Ctrl Pts',(3.1547007261638,-36.2742356128,9.97878201671825));
#60572=CARTESIAN_POINT('Ctrl Pts',(3.28770166123135,-36.2742356128,9.8866861314215));
#60573=CARTESIAN_POINT('Ctrl Pts',(3.41667075619548,-36.2742356128,9.78876778525046));
#60574=CARTESIAN_POINT('Ctrl Pts',(3.54111654199492,-36.2742356128,9.68540334602765));
#60575=CARTESIAN_POINT('Ctrl Pts',(3.64858270370976,-36.2742356128,9.59614215112479));
#60576=CARTESIAN_POINT('Ctrl Pts',(3.75267608382533,-36.2742356128,9.50282039201421));
#60577=CARTESIAN_POINT('Ctrl Pts',(3.85310031130201,-36.2742356128,9.40570437827657));
#60578=CARTESIAN_POINT('Ctrl Pts',(3.96951110904278,-36.2742356128,9.29312843005505));
#60579=CARTESIAN_POINT('Ctrl Pts',(4.080990284725,-36.2742356128,9.17545378429104));
#60580=CARTESIAN_POINT('Ctrl Pts',(4.18710961345993,-36.2742356128,9.05313210221856));
#60581=CARTESIAN_POINT('Ctrl Pts',(4.29281661966718,-36.2742356128,8.93128569628798));
#60582=CARTESIAN_POINT('Ctrl Pts',(4.39320516825513,-36.2742356128,8.80482851427014));
#60583=CARTESIAN_POINT('Ctrl Pts',(4.48789158020286,-36.2742356128,8.67424009053965));
#60584=CARTESIAN_POINT('Ctrl Pts',(4.58220205051933,-36.2742356128,8.54417015329556));
#60585=CARTESIAN_POINT('Ctrl Pts',(4.67085539903292,-36.2742356128,8.41000192729587));
#60586=CARTESIAN_POINT('Ctrl Pts',(4.75351448617961,-36.2742356128,8.27223895635978));
#60587=CARTESIAN_POINT('Ctrl Pts',(4.8357582380376,-36.2742356128,8.13516819997965));
#60588=CARTESIAN_POINT('Ctrl Pts',(4.91206765482947,-36.2742356128,7.99453894339549));
#60589=CARTESIAN_POINT('Ctrl Pts',(4.98215479283938,-36.2742356128,7.85087347247978));
#60590=CARTESIAN_POINT('Ctrl Pts',(5.05182619136561,-36.2742356128,7.70806018943188));
#60591=CARTESIAN_POINT('Ctrl Pts',(5.11534876334311,-36.2742356128,7.56224681130156));
#60592=CARTESIAN_POINT('Ctrl Pts',(5.1724856667926,-36.2742356128,7.41396932577449));
#60593=CARTESIAN_POINT('Ctrl Pts',(5.22901464574304,-36.2742356128,7.26726948115318));
#60594=CARTESIAN_POINT('Ctrl Pts',(5.27929301765054,-36.2742356128,7.11815789491069));
#60595=CARTESIAN_POINT('Ctrl Pts',(5.32313836217568,-36.2742356128,6.9671730420275));
#60596=CARTESIAN_POINT('Ctrl Pts',(5.36670086892032,-36.2742356128,6.8171621630323));
#60597=CARTESIAN_POINT('Ctrl Pts',(5.40391295200194,-36.2742356128,6.66530229338273));
#60598=CARTESIAN_POINT('Ctrl Pts',(5.43464400506635,-36.2742356128,6.51213790757587));
#60599=CARTESIAN_POINT('Ctrl Pts',(5.46503102108015,-36.2742356128,6.36068821157939));
#60600=CARTESIAN_POINT('Ctrl Pts',(5.48908122944364,-36.2742356128,6.20796322934857));
#60601=CARTESIAN_POINT('Ctrl Pts',(5.50671718129312,-36.2742356128,6.05450262692307));
#60602=CARTESIAN_POINT('Ctrl Pts',(5.52334991985196,-36.2742356128,5.90977156273051));
#60603=CARTESIAN_POINT('Ctrl Pts',(5.53427767276785,-36.2742356128,5.7643864062297));
#60604=CARTESIAN_POINT('Ctrl Pts',(5.53947703985376,-36.2742356128,5.61880872757919));
#60605=CARTESIAN_POINT('Ctrl Pts',(5.53961786526957,-36.2742356128,5.61486574052124));
#60606=CARTESIAN_POINT('Ctrl Pts',(5.53975449137418,-36.2742356128,5.61092259462969));
#60607=CARTESIAN_POINT('Ctrl Pts',(5.53988691225,-36.2742356128,5.60697948238));
#60608=CARTESIAN_POINT('Origin',(-3.35265884719E-30,-38.2742356128,3.15283103411E-22));
#60609=CARTESIAN_POINT('',(10.0697226343,-38.2742356128,2.85693747561));
#60610=CARTESIAN_POINT('',(10.7486858853,-38.2742356128,0.75419629452));
#60611=CARTESIAN_POINT('Ctrl Pts',(10.0697226344311,-38.2742356128,2.85693747569001));
#60612=CARTESIAN_POINT('Ctrl Pts',(10.0776188393002,-38.2742356128,2.84400003564299));
#60613=CARTESIAN_POINT('Ctrl Pts',(10.0855029430265,-38.2742356128062,2.8309683272098));
#60614=CARTESIAN_POINT('Ctrl Pts',(10.0933605009977,-38.2742356127531,2.81785320039552));
#60615=CARTESIAN_POINT('Ctrl Pts',(10.1109731368737,-38.2742356126341,2.78845577769836));
#60616=CARTESIAN_POINT('Ctrl Pts',(10.1284465935078,-38.2742356123565,2.75863590433942));
#60617=CARTESIAN_POINT('Ctrl Pts',(10.1456594638731,-38.2742356122038,2.72850124510115));
#60618=CARTESIAN_POINT('Ctrl Pts',(10.1640041649347,-38.2742356120411,2.69638508413648));
#60619=CARTESIAN_POINT('Ctrl Pts',(10.1820528841507,-38.2742356120154,2.66391120473192));
#60620=CARTESIAN_POINT('Ctrl Pts',(10.1997035416477,-38.2742356121317,2.63116652928536));
#60621=CARTESIAN_POINT('Ctrl Pts',(10.2172099443932,-38.274235612247,2.59868946851639));
#60622=CARTESIAN_POINT('Ctrl Pts',(10.2343253141801,-38.2742356124941,2.56594530790568));
#60623=CARTESIAN_POINT('Ctrl Pts',(10.250987782861,-38.2742356126595,2.53298508626117));
#60624=CARTESIAN_POINT('Ctrl Pts',(10.2704216371138,-38.2742356128525,2.49454275482485));
#60625=CARTESIAN_POINT('Ctrl Pts',(10.2892457459371,-38.2742356127993,2.45580776597392));
#60626=CARTESIAN_POINT('Ctrl Pts',(10.3074100253296,-38.2742356127999,2.41681942324682));
#60627=CARTESIAN_POINT('Ctrl Pts',(10.3156933625564,-38.2742356128001,2.39903982496235));
#60628=CARTESIAN_POINT('Ctrl Pts',(10.3238401489906,-38.2742356128,2.3812070736748));
#60629=CARTESIAN_POINT('Ctrl Pts',(10.3318485530151,-38.2742356128,2.3633231281257));
#60630=CARTESIAN_POINT('Ctrl Pts',(10.3539275416858,-38.2742356128,2.31401749494804));
#60631=CARTESIAN_POINT('Ctrl Pts',(10.3749527959892,-38.2742356128,2.26431782944173));
#60632=CARTESIAN_POINT('Ctrl Pts',(10.394940586342,-38.2742356128,2.21425144102859));
#60633=CARTESIAN_POINT('Ctrl Pts',(10.3981007591477,-38.2742356128,2.20633568664295));
#60634=CARTESIAN_POINT('Ctrl Pts',(10.4012351022165,-38.2742356128,2.19841078058856));
#60635=CARTESIAN_POINT('Ctrl Pts',(10.4043437787341,-38.2742356128,2.19047687263431));
#60636=CARTESIAN_POINT('Ctrl Pts',(10.4217205779389,-38.2742356128,2.1461281201514));
#60637=CARTESIAN_POINT('Ctrl Pts',(10.438297812734,-38.2742356128,2.10148777201649));
#60638=CARTESIAN_POINT('Ctrl Pts',(10.4541056780973,-38.2742356128,2.05660920251616));
#60639=CARTESIAN_POINT('Ctrl Pts',(10.4675450264758,-38.2742356128,2.01845485868911));
#60640=CARTESIAN_POINT('Ctrl Pts',(10.4804291335677,-38.2742356128,1.98012800337298));
#60641=CARTESIAN_POINT('Ctrl Pts',(10.4927701214951,-38.2742356128,1.94169718949288));
#60642=CARTESIAN_POINT('Ctrl Pts',(10.5039195447129,-38.2742356128,1.90697700249726));
#60643=CARTESIAN_POINT('Ctrl Pts',(10.514626001726,-38.2742356128,1.87217183244256));
#60644=CARTESIAN_POINT('Ctrl Pts',(10.5248856152871,-38.2742356128,1.83736677743975));
#60645=CARTESIAN_POINT('Ctrl Pts',(10.5346062277631,-38.2742356128,1.80439024768327));
#60646=CARTESIAN_POINT('Ctrl Pts',(10.5439352285554,-38.2742356127913,1.77139355586021));
#60647=CARTESIAN_POINT('Ctrl Pts',(10.5528945995153,-38.2742356127464,1.73842376238139));
#60648=CARTESIAN_POINT('Ctrl Pts',(10.560024647317,-38.2742356127106,1.71218573690282));
#60649=CARTESIAN_POINT('Ctrl Pts',(10.5669209610923,-38.2742356126719,1.6859628905476));
#60650=CARTESIAN_POINT('Ctrl Pts',(10.57359934485,-38.2742356127066,1.659756377355));
#60651=CARTESIAN_POINT('Ctrl Pts',(10.5886695541833,-38.2742356127848,1.60061966793));
#60652=CARTESIAN_POINT('Ctrl Pts',(10.6026459235773,-38.2742356128,1.54154272041369));
#60653=CARTESIAN_POINT('Ctrl Pts',(10.6157344632958,-38.2742356128,1.48260713307673));
#60654=CARTESIAN_POINT('Ctrl Pts',(10.6229873571614,-38.2742356128,1.44994851958333));
#60655=CARTESIAN_POINT('Ctrl Pts',(10.6299550378573,-38.2742356128,1.4173888281794));
#60656=CARTESIAN_POINT('Ctrl Pts',(10.6366903508906,-38.2742356128,1.38487935873198));
#60657=CARTESIAN_POINT('Ctrl Pts',(10.6428618776733,-38.2742356128,1.35509112759876));
#60658=CARTESIAN_POINT('Ctrl Pts',(10.648838346926,-38.2742356128,1.32534429110625));
#60659=CARTESIAN_POINT('Ctrl Pts',(10.6546508806194,-38.2742356128,1.2956426679367));
#60660=CARTESIAN_POINT('Ctrl Pts',(10.6599433244144,-38.2742356128,1.26859866620975));
#60661=CARTESIAN_POINT('Ctrl Pts',(10.6650998558584,-38.2742356128,1.24159183508873));
#60662=CARTESIAN_POINT('Ctrl Pts',(10.6701355237829,-38.2742356128,1.21466761412695));
#60663=CARTESIAN_POINT('Ctrl Pts',(10.6725084893088,-38.2742356128,1.20198007215385));
#60664=CARTESIAN_POINT('Ctrl Pts',(10.6748544884253,-38.2742356128,1.18931154490809));
#60665=CARTESIAN_POINT('Ctrl Pts',(10.6771743463304,-38.2742356128,1.17667085189563));
#60666=CARTESIAN_POINT('Ctrl Pts',(10.6794225509139,-38.2742356128,1.16442059126226));
#60667=CARTESIAN_POINT('Ctrl Pts',(10.681645032157,-38.2742356128,1.15220289282337));
#60668=CARTESIAN_POINT('Ctrl Pts',(10.68385417031,-38.2742356127999,1.1399539012589));
#60669=CARTESIAN_POINT('Ctrl Pts',(10.684249048922,-38.2742356127998,1.13776442081368));
#60670=CARTESIAN_POINT('Ctrl Pts',(10.6846434790834,-38.2742356127998,1.13557407331553));
#60671=CARTESIAN_POINT('Ctrl Pts',(10.6850375033588,-38.2742356127997,1.13338266268583));
#60672=CARTESIAN_POINT('Ctrl Pts',(10.6874088318044,-38.2742356127994,1.12019425098996));
#60673=CARTESIAN_POINT('Ctrl Pts',(10.6897723350178,-38.2742356127989,1.10692783802663));
#60674=CARTESIAN_POINT('Ctrl Pts',(10.6921362766321,-38.2742356127984,1.093545659875));
#60675=CARTESIAN_POINT('Ctrl Pts',(10.6948056682513,-38.2742356127979,1.078434341563));
#60676=CARTESIAN_POINT('Ctrl Pts',(10.6974756107928,-38.2742356127975,1.06317553188));
#60677=CARTESIAN_POINT('Ctrl Pts',(10.7001461013002,-38.2742356127972,1.04778309134131));
#60678=CARTESIAN_POINT('Ctrl Pts',(10.7032679269097,-38.274235612797,1.0297892003566));
#60679=CARTESIAN_POINT('Ctrl Pts',(10.7063903477994,-38.274235612797,1.0116137923099));
#60680=CARTESIAN_POINT('Ctrl Pts',(10.7094989857158,-38.2742356127972,0.993358985853085));
#60681=CARTESIAN_POINT('Ctrl Pts',(10.7131804317752,-38.2742356127974,0.97174048697887));
#60682=CARTESIAN_POINT('Ctrl Pts',(10.7168416621835,-38.2742356127979,0.950016346973492));
#60683=CARTESIAN_POINT('Ctrl Pts',(10.7204480893748,-38.2742356127984,0.928407232902512));
#60684=CARTESIAN_POINT('Ctrl Pts',(10.7231942485053,-38.2742356127987,0.911952702487821));
#60685=CARTESIAN_POINT('Ctrl Pts',(10.7259082038139,-38.2742356127991,0.89556715018462));
#60686=CARTESIAN_POINT('Ctrl Pts',(10.7285778286188,-38.2742356127993,0.879323202461527));
#60687=CARTESIAN_POINT('Ctrl Pts',(10.730988497373,-38.2742356127995,0.864654932542631));
#60688=CARTESIAN_POINT('Ctrl Pts',(10.7333628612606,-38.2742356127997,0.850103016441976));
#60689=CARTESIAN_POINT('Ctrl Pts',(10.7356981739405,-38.2742356127998,0.835680045130879));
#60690=CARTESIAN_POINT('Ctrl Pts',(10.7378330625263,-38.2742356127999,0.822494899908279));
#60691=CARTESIAN_POINT('Ctrl Pts',(10.7399352552987,-38.2742356128,0.809417839967112));
#60692=CARTESIAN_POINT('Ctrl Pts',(10.7420094653683,-38.2742356128,0.796414883560318));
#60693=CARTESIAN_POINT('Ctrl Pts',(10.7429375365281,-38.2742356128,0.790596924709413));
#60694=CARTESIAN_POINT('Ctrl Pts',(10.7438601064876,-38.2742356128,0.784793160677161));
#60695=CARTESIAN_POINT('Ctrl Pts',(10.7447781403271,-38.2742356128,0.778997116234539));
#60696=CARTESIAN_POINT('Ctrl Pts',(10.7460880302118,-38.2742356128,0.770727072518073));
#60697=CARTESIAN_POINT('Ctrl Pts',(10.7473907134667,-38.2742356128,0.762459686238333));
#60698=CARTESIAN_POINT('Ctrl Pts',(10.7486858853,-38.2742356128,0.75419629452));
#60699=CARTESIAN_POINT('',(6.79137814506709,-38.2742356128,3.87179982043696));
#60700=CARTESIAN_POINT('Ctrl Pts',(6.79137821743737,-38.2742356128,3.87179986876002));
#60701=CARTESIAN_POINT('Ctrl Pts',(6.80226365184488,-38.2742356128,3.87906825465593));
#60702=CARTESIAN_POINT('Ctrl Pts',(6.81320993266797,-38.2742356128,3.88625408753819));
#60703=CARTESIAN_POINT('Ctrl Pts',(6.82421601895544,-38.2742356128,3.89335477754412));
#60704=CARTESIAN_POINT('Ctrl Pts',(6.87563019015907,-38.2742356128,3.9265251600119));
#60705=CARTESIAN_POINT('Ctrl Pts',(6.92832455620214,-38.2742356128001,3.95781726483387));
#60706=CARTESIAN_POINT('Ctrl Pts',(6.98218879584778,-38.2742356127999,3.98701052943907));
#60707=CARTESIAN_POINT('Ctrl Pts',(7.03678152742978,-38.2742356127997,4.01659862107609));
#60708=CARTESIAN_POINT('Ctrl Pts',(7.09257560090438,-38.2742356128,4.04403030945431));
#60709=CARTESIAN_POINT('Ctrl Pts',(7.14940901416357,-38.2742356127945,4.06910193455759));
#60710=CARTESIAN_POINT('Ctrl Pts',(7.20715367516088,-38.2742356127889,4.09457554962341));
#60711=CARTESIAN_POINT('Ctrl Pts',(7.26597081847314,-38.2742356127788,4.11761237182838));
#60712=CARTESIAN_POINT('Ctrl Pts',(7.32564859213579,-38.2742356127345,4.13803193031878));
#60713=CARTESIAN_POINT('Ctrl Pts',(7.33536951733907,-38.2742356127273,4.14135807653012));
#60714=CARTESIAN_POINT('Ctrl Pts',(7.34511319782085,-38.2742356127191,4.14461485693852));
#60715=CARTESIAN_POINT('Ctrl Pts',(7.3548786281491,-38.2742356127097,4.14780158544441));
#60716=CARTESIAN_POINT('Ctrl Pts',(7.40494059735844,-38.2742356126613,4.16413818290895));
#60717=CARTESIAN_POINT('Ctrl Pts',(7.45560498502167,-38.2742356122277,4.17865129560831));
#60718=CARTESIAN_POINT('Ctrl Pts',(7.50678821535502,-38.2742356117529,4.19125010342492));
#60719=CARTESIAN_POINT('Ctrl Pts',(7.55797144568837,-38.2742356112782,4.20384891124152));
#60720=CARTESIAN_POINT('Ctrl Pts',(7.60968799204104,-38.2742356112205,4.21453391209546));
#60721=CARTESIAN_POINT('Ctrl Pts',(7.66177351399378,-38.2742356112926,4.2232251536338));
#60722=CARTESIAN_POINT('Ctrl Pts',(7.71385951973192,-38.2742356113647,4.23191647589892));
#60723=CARTESIAN_POINT('Ctrl Pts',(7.76630497190309,-38.2742356112526,4.23861290835011));
#60724=CARTESIAN_POINT('Ctrl Pts',(7.81885823355599,-38.2742356112199,4.24325350235059));
#60725=CARTESIAN_POINT('Ctrl Pts',(7.87141149519477,-38.2742356111873,4.24789409634982));
#60726=CARTESIAN_POINT('Ctrl Pts',(7.92410320133167,-38.2742356114824,4.25048261299401));
#60727=CARTESIAN_POINT('Ctrl Pts',(7.97680547469087,-38.2742356117947,4.25099795223007));
#60728=CARTESIAN_POINT('Ctrl Pts',(8.04056423400334,-38.2742356121725,4.25162140522785));
#60729=CARTESIAN_POINT('Ctrl Pts',(8.10433843773227,-38.2742356123995,4.24920992909844));
#60730=CARTESIAN_POINT('Ctrl Pts',(8.16783744970057,-38.2742356125418,4.2437573156433));
#60731=CARTESIAN_POINT('Ctrl Pts',(8.23026340554995,-38.2742356126817,4.23839684472787));
#60732=CARTESIAN_POINT('Ctrl Pts',(8.29242292091689,-38.2742356127405,4.23009699484735));
#60733=CARTESIAN_POINT('Ctrl Pts',(8.35403932933331,-38.2742356127697,4.21890169877675));
#60734=CARTESIAN_POINT('Ctrl Pts',(8.4140575137154,-38.2742356127981,4.2079967894994));
#60735=CARTESIAN_POINT('Ctrl Pts',(8.47356000826017,-38.2742356127991,4.19434463963401));
#60736=CARTESIAN_POINT('Ctrl Pts',(8.53229689916312,-38.2742356127998,4.17803492716954));
#60737=CARTESIAN_POINT('Ctrl Pts',(8.55498221166293,-38.2742356128001,4.17173580376769));
#60738=CARTESIAN_POINT('Ctrl Pts',(8.57755341554526,-38.2742356128,4.16504079768994));
#60739=CARTESIAN_POINT('Ctrl Pts',(8.59999653905443,-38.2742356128,4.15795713803855));
#60740=CARTESIAN_POINT('Ctrl Pts',(8.65275187384972,-38.2742356128,4.1413061207979));
#60741=CARTESIAN_POINT('Ctrl Pts',(8.70480164426777,-38.2742356128066,4.12250510557686));
#60742=CARTESIAN_POINT('Ctrl Pts',(8.75602778748263,-38.2742356127783,4.10163626378869));
#60743=CARTESIAN_POINT('Ctrl Pts',(8.80228054147308,-38.2742356127528,4.08279351388176));
#60744=CARTESIAN_POINT('Ctrl Pts',(8.84786037356255,-38.2742356126966,4.06226581784222));
#60745=CARTESIAN_POINT('Ctrl Pts',(8.8926632647348,-38.2742356125373,4.04014566152166));
#60746=CARTESIAN_POINT('Ctrl Pts',(8.94857266920348,-38.2742356123387,4.01254197938691));
#60747=CARTESIAN_POINT('Ctrl Pts',(9.00330501446036,-38.2742356122495,3.98243553233308));
#60748=CARTESIAN_POINT('Ctrl Pts',(9.05668746409715,-38.2742356123646,3.95003024395078));
#60749=CARTESIAN_POINT('Ctrl Pts',(9.09347531147182,-38.274235612444,3.92769854483896));
#60750=CARTESIAN_POINT('Ctrl Pts',(9.12962185589216,-38.2742356126008,3.90427618224411));
#60751=CARTESIAN_POINT('Ctrl Pts',(9.16507828894361,-38.2742356127068,3.87984233486085));
#60752=CARTESIAN_POINT('Ctrl Pts',(9.20849780261757,-38.2742356128365,3.8499209446007));
#60753=CARTESIAN_POINT('Ctrl Pts',(9.25088407878093,-38.2742356128,3.81848432781475));
#60754=CARTESIAN_POINT('Ctrl Pts',(9.29213478581693,-38.2742356128,3.7857321116292));
#60755=CARTESIAN_POINT('Ctrl Pts',(9.31268689240908,-38.2742356128,3.76941416009476));
#60756=CARTESIAN_POINT('Ctrl Pts',(9.33295849535396,-38.2742356128,3.75276882613797));
#60757=CARTESIAN_POINT('Ctrl Pts',(9.35293864601996,-38.2742356128,3.73582645507306));
#60758=CARTESIAN_POINT('Ctrl Pts',(9.36914328585316,-38.2742356128,3.72208556664751));
#60759=CARTESIAN_POINT('Ctrl Pts',(9.38514901708334,-38.2742356128,3.70815579621019));
#60760=CARTESIAN_POINT('Ctrl Pts',(9.40097242007251,-38.2742356128,3.69403625763351));
#60761=CARTESIAN_POINT('Ctrl Pts',(9.40479906360245,-38.2742356128,3.69062166717043));
#60762=CARTESIAN_POINT('Ctrl Pts',(9.40861504872694,-38.2742356128,3.68719596937193));
#60763=CARTESIAN_POINT('Ctrl Pts',(9.41242061503587,-38.2742356128,3.68375913884913));
#60764=CARTESIAN_POINT('Ctrl Pts',(9.44710216596526,-38.2742356128,3.65243801522751));
#60765=CARTESIAN_POINT('Ctrl Pts',(9.48095984392308,-38.2742356128367,3.62015512214142));
#60766=CARTESIAN_POINT('Ctrl Pts',(9.51391146087876,-38.2742356126435,3.58711756919405));
#60767=CARTESIAN_POINT('Ctrl Pts',(9.54924040229739,-38.2742356124364,3.55169649185321));
#60768=CARTESIAN_POINT('Ctrl Pts',(9.58352812796506,-38.2742356119099,3.51540827645441));
#60769=CARTESIAN_POINT('Ctrl Pts',(9.61673281222635,-38.2742356107591,3.47851494924075));
#60770=CARTESIAN_POINT('Ctrl Pts',(9.62208609212353,-38.2742356105735,3.47256698402722));
#60771=CARTESIAN_POINT('Ctrl Pts',(9.62741133109786,-38.2742356103727,3.4666032974567));
#60772=CARTESIAN_POINT('Ctrl Pts',(9.63270847298428,-38.2742356101568,3.46062499292125));
#60773=CARTESIAN_POINT('Ctrl Pts',(9.64981262109995,-38.2742356094594,3.4413214121512));
#60774=CARTESIAN_POINT('Ctrl Pts',(9.6666629516528,-38.2742356085896,3.42182106045621));
#60775=CARTESIAN_POINT('Ctrl Pts',(9.6832637335943,-38.2742356078081,3.40214758502691));
#60776=CARTESIAN_POINT('Ctrl Pts',(9.6998645155358,-38.2742356070266,3.38247410959761));
#60777=CARTESIAN_POINT('Ctrl Pts',(9.71621862624953,-38.274235606372,3.3626240804197));
#60778=CARTESIAN_POINT('Ctrl Pts',(9.73233640212346,-38.2742356060233,3.34261606036647));
#60779=CARTESIAN_POINT('Ctrl Pts',(9.78137505758533,-38.2742356049622,3.28174125918181));
#60780=CARTESIAN_POINT('Ctrl Pts',(9.82817652284925,-38.2742356070341,3.219469380873));
#60781=CARTESIAN_POINT('Ctrl Pts',(9.87305796788631,-38.2742356090049,3.15633700294021));
#60782=CARTESIAN_POINT('Ctrl Pts',(9.90790930677723,-38.2742356105353,3.10731344996618));
#60783=CARTESIAN_POINT('Ctrl Pts',(9.94160538607107,-38.2742356118045,3.05776986132032));
#60784=CARTESIAN_POINT('Ctrl Pts',(9.97426184086033,-38.274235612334,3.00794438327731));
#60785=CARTESIAN_POINT('Ctrl Pts',(10.0025204308224,-38.2742356127921,2.96482893296992));
#60786=CARTESIAN_POINT('Ctrl Pts',(10.0300010756658,-38.2742356127974,2.92150209599565));
#60787=CARTESIAN_POINT('Ctrl Pts',(10.0567356987662,-38.2742356127997,2.87811469479087));
#60788=CARTESIAN_POINT('Ctrl Pts',(10.0608963896839,-38.2742356128001,2.87136234352503));
#60789=CARTESIAN_POINT('Ctrl Pts',(10.065038908559,-38.2742356128,2.86460852225224));
#60790=CARTESIAN_POINT('Ctrl Pts',(10.0691632550904,-38.2742356128,2.85785379691802));
#60791=CARTESIAN_POINT('Ctrl Pts',(10.069349746965,-38.2742356128,2.85754836637758));
#60792=CARTESIAN_POINT('Ctrl Pts',(10.0695362045312,-38.2742356128,2.8572429295994));
#60793=CARTESIAN_POINT('Ctrl Pts',(10.0697226343,-38.2742356128,2.85693747561));
#60794=CARTESIAN_POINT('',(5.86597170597801,-38.2742356128,4.46707956737663));
#60795=CARTESIAN_POINT('Ctrl Pts',(5.86597168188,-38.2742356128,4.46707937639));
#60796=CARTESIAN_POINT('Ctrl Pts',(5.86521847952036,-38.2742356128,4.46244689300994));
#60797=CARTESIAN_POINT('Ctrl Pts',(5.86451251383266,-38.2742356128,4.45775891558074));
#60798=CARTESIAN_POINT('Ctrl Pts',(5.86386803963271,-38.2742356127999,4.45310957470034));
#60799=CARTESIAN_POINT('Ctrl Pts',(5.86322141073989,-38.2742356127999,4.4484446895179));
#60800=CARTESIAN_POINT('Ctrl Pts',(5.86262940399853,-38.2742356127997,4.44377160748202));
#60801=CARTESIAN_POINT('Ctrl Pts',(5.8620923017773,-38.2742356127993,4.43909214018255));
#60802=CARTESIAN_POINT('Ctrl Pts',(5.85880657218188,-38.2742356127967,4.41046544010783));
#60803=CARTESIAN_POINT('Ctrl Pts',(5.85757720777026,-38.2742356127862,4.38158802376726));
#60804=CARTESIAN_POINT('Ctrl Pts',(5.8584296426603,-38.2742356127781,4.35276644081144));
#60805=CARTESIAN_POINT('Ctrl Pts',(5.85930076534106,-38.2742356127698,4.32331300700491));
#60806=CARTESIAN_POINT('Ctrl Pts',(5.86234582254843,-38.2742356127665,4.29391819633034));
#60807=CARTESIAN_POINT('Ctrl Pts',(5.8675381376056,-38.2742356127753,4.26490239478237));
#60808=CARTESIAN_POINT('Ctrl Pts',(5.86889338350707,-38.2742356127776,4.25732898182635));
#60809=CARTESIAN_POINT('Ctrl Pts',(5.87039464119523,-38.2742356127806,4.24978133983799));
#60810=CARTESIAN_POINT('Ctrl Pts',(5.87204087021659,-38.2742356127838,4.24226504999152));
#60811=CARTESIAN_POINT('Ctrl Pts',(5.87836316827691,-38.2742356127961,4.21339894199529));
#60812=CARTESIAN_POINT('Ctrl Pts',(5.88682789242818,-38.2742356127977,4.18500208544504));
#60813=CARTESIAN_POINT('Ctrl Pts',(5.89734093285122,-38.2742356127986,4.15738756121468));
#60814=CARTESIAN_POINT('Ctrl Pts',(5.90798936103777,-38.2742356127994,4.12941741496392));
#60815=CARTESIAN_POINT('Ctrl Pts',(5.92073893937052,-38.2742356127996,4.10225034381996));
#60816=CARTESIAN_POINT('Ctrl Pts',(5.93544258166133,-38.2742356127962,4.07619079382842));
#60817=CARTESIAN_POINT('Ctrl Pts',(5.94424329501613,-38.2742356127942,4.06059311910984));
#60818=CARTESIAN_POINT('Ctrl Pts',(5.9537431263084,-38.2742356127907,4.04539178133931));
#60819=CARTESIAN_POINT('Ctrl Pts',(5.96390288113939,-38.2742356127826,4.03064749997891));
#60820=CARTESIAN_POINT('Ctrl Pts',(5.9810490467527,-38.2742356127691,4.00576423318162));
#60821=CARTESIAN_POINT('Ctrl Pts',(6.00007557603257,-38.2742356127705,3.98218298150727));
#60822=CARTESIAN_POINT('Ctrl Pts',(6.0207634836268,-38.2742356127792,3.96016862488714));
#60823=CARTESIAN_POINT('Ctrl Pts',(6.04132264280314,-38.2742356127878,3.93829127166248));
#60824=CARTESIAN_POINT('Ctrl Pts',(6.06352216120708,-38.274235612797,3.91796176161847));
#60825=CARTESIAN_POINT('Ctrl Pts',(6.08711174806247,-38.274235612799,3.89940302051962));
#60826=CARTESIAN_POINT('Ctrl Pts',(6.10047468249298,-38.2742356128002,3.88888993939034));
#60827=CARTESIAN_POINT('Ctrl Pts',(6.11428307295518,-38.2742356128,3.87894438340428));
#60828=CARTESIAN_POINT('Ctrl Pts',(6.12848708214859,-38.2742356128,3.86960082529007));
#60829=CARTESIAN_POINT('Ctrl Pts',(6.15338993303026,-38.2742356128,3.85321944794413));
#60830=CARTESIAN_POINT('Ctrl Pts',(6.17951083601368,-38.2742356128,3.8386899453089));
#60831=CARTESIAN_POINT('Ctrl Pts',(6.20656832160519,-38.2742356127994,3.82617616464038));
#60832=CARTESIAN_POINT('Ctrl Pts',(6.23388644440146,-38.2742356127989,3.81354184221628));
#60833=CARTESIAN_POINT('Ctrl Pts',(6.26215874205547,-38.2742356127977,3.80296251155965));
#60834=CARTESIAN_POINT('Ctrl Pts',(6.29106888820992,-38.2742356127976,3.79456090317743));
#60835=CARTESIAN_POINT('Ctrl Pts',(6.3074976151048,-38.2742356127975,3.78978653334714));
#60836=CARTESIAN_POINT('Ctrl Pts',(6.32413188205186,-38.2742356127978,3.78571455856394));
#60837=CARTESIAN_POINT('Ctrl Pts',(6.34091089081714,-38.2742356127985,3.78236053332006));
#60838=CARTESIAN_POINT('Ctrl Pts',(6.37044752808834,-38.2742356127997,3.77645633311296));
#60839=CARTESIAN_POINT('Ctrl Pts',(6.40043493735285,-38.2742356127998,3.77278002228652));
#60840=CARTESIAN_POINT('Ctrl Pts',(6.43053277796928,-38.2742356127999,3.77137787478142));
#60841=CARTESIAN_POINT('Ctrl Pts',(6.46027533040864,-38.2742356128,3.76999227884349));
#60842=CARTESIAN_POINT('Ctrl Pts',(6.49012515981829,-38.2742356128,3.77082754411741));
#60843=CARTESIAN_POINT('Ctrl Pts',(6.5197493946603,-38.2742356127999,3.7738779521685));
#60844=CARTESIAN_POINT('Ctrl Pts',(6.53700806446756,-38.2742356127999,3.77565507774194));
#60845=CARTESIAN_POINT('Ctrl Pts',(6.55419012590196,-38.2742356127999,3.77818308879307));
#60846=CARTESIAN_POINT('Ctrl Pts',(6.57123018973728,-38.2742356127998,3.78145267165003));
#60847=CARTESIAN_POINT('Ctrl Pts',(6.59976050908503,-38.2742356127997,3.78692696117996));
#60848=CARTESIAN_POINT('Ctrl Pts',(6.62788960711445,-38.2742356127906,3.79448443707445));
#60849=CARTESIAN_POINT('Ctrl Pts',(6.65531799034395,-38.2742356127749,3.80403807813415));
#60850=CARTESIAN_POINT('Ctrl Pts',(6.66446340893655,-38.2742356127697,3.80722353918898));
#60851=CARTESIAN_POINT('Ctrl Pts',(6.67353103771832,-38.2742356127651,3.81063051321018));
#60852=CARTESIAN_POINT('Ctrl Pts',(6.68251015765301,-38.2742356127641,3.81425453223265));
#60853=CARTESIAN_POINT('Ctrl Pts',(6.70935764852629,-38.2742356127609,3.82509031773702));
#60854=CARTESIAN_POINT('Ctrl Pts',(6.73541115755773,-38.2742356127925,3.83786890772086));
#60855=CARTESIAN_POINT('Ctrl Pts',(6.76040182236934,-38.2742356127979,3.85244737074258));
#60856=CARTESIAN_POINT('Ctrl Pts',(6.76883599265748,-38.2742356127998,3.85736749754158));
#60857=CARTESIAN_POINT('Ctrl Pts',(6.77714924361623,-38.2742356128,3.86249222401201));
#60858=CARTESIAN_POINT('Ctrl Pts',(6.78533170849366,-38.2742356128,3.86781477988002));
#60859=CARTESIAN_POINT('Ctrl Pts',(6.78735517139677,-38.2742356128,3.86913100848716));
#60860=CARTESIAN_POINT('Ctrl Pts',(6.7893712469383,-38.2742356128,3.87045977491255));
#60861=CARTESIAN_POINT('Ctrl Pts',(6.79137807329,-38.2742356128,3.87179977251));
#60862=CARTESIAN_POINT('',(1.96099433484507E-5,-38.2742356128,11.3643459819103));
#60863=CARTESIAN_POINT('Ctrl Pts',(1.96099437674846E-5,-38.2742356128,11.3643459876291));
#60864=CARTESIAN_POINT('Ctrl Pts',(0.0472697587385178,-38.2742356128,11.3643425323295));
#60865=CARTESIAN_POINT('Ctrl Pts',(0.0945221110592471,-38.2742356128,11.363777913887));
#60866=CARTESIAN_POINT('Ctrl Pts',(0.141759781888426,-38.2742356128,11.3626518420063));
#60867=CARTESIAN_POINT('Ctrl Pts',(0.245241952691282,-38.2742356128,11.3601849895844));
#60868=CARTESIAN_POINT('Ctrl Pts',(0.348663149583877,-38.2742356128,11.3550229294214));
#60869=CARTESIAN_POINT('Ctrl Pts',(0.451876489369207,-38.2742356128,11.3471684549389));
#60870=CARTESIAN_POINT('Ctrl Pts',(0.614063148796439,-38.2742356128,11.3348261454999));
#60871=CARTESIAN_POINT('Ctrl Pts',(0.775739638000677,-38.2742356128,11.315833030005));
#60872=CARTESIAN_POINT('Ctrl Pts',(0.93635482831518,-38.2742356128,11.290242195175));
#60873=CARTESIAN_POINT('Ctrl Pts',(1.09834028128939,-38.2742356128,11.2644330362542));
#60874=CARTESIAN_POINT('Ctrl Pts',(1.25924606969199,-38.2742356128,11.2319132010809));
#60875=CARTESIAN_POINT('Ctrl Pts',(1.41851896539168,-38.2742356128,11.1927887894903));
#60876=CARTESIAN_POINT('Ctrl Pts',(1.57908539079494,-38.2742356128,11.1533466302484));
#60877=CARTESIAN_POINT('Ctrl Pts',(1.73799210302976,-38.2742356128,11.1071922912551));
#60878=CARTESIAN_POINT('Ctrl Pts',(1.8946873563024,-38.2742356128,11.0544851600217));
#60879=CARTESIAN_POINT('Ctrl Pts',(2.05312041979911,-38.2742356128,11.0011934865662));
#60880=CARTESIAN_POINT('Ctrl Pts',(2.20929248845345,-38.2742356128,10.9412029647644));
#60881=CARTESIAN_POINT('Ctrl Pts',(2.36265166093631,-38.2742356128,10.8747284217424));
#60882=CARTESIAN_POINT('Ctrl Pts',(2.51692692416807,-38.2742356128,10.8078567931537));
#60883=CARTESIAN_POINT('Ctrl Pts',(2.66835537858543,-38.2742356128,10.7344235939096));
#60884=CARTESIAN_POINT('Ctrl Pts',(2.81639684408017,-38.2742356128,10.6546960255344));
#60885=CARTESIAN_POINT('Ctrl Pts',(2.9651921921399,-38.2742356128,10.5745624545331));
#60886=CARTESIAN_POINT('Ctrl Pts',(3.11056575655573,-38.2742356128,10.4880704051236));
#60887=CARTESIAN_POINT('Ctrl Pts',(3.25199403978543,-38.2742356128,10.3955377043536));
#60888=CARTESIAN_POINT('Ctrl Pts',(3.39399708912114,-38.2742356128,10.302628949665));
#60889=CARTESIAN_POINT('Ctrl Pts',(3.53202251132963,-38.2742356128,10.2036305196863));
#60890=CARTESIAN_POINT('Ctrl Pts',(3.66556871335094,-38.2742356128,10.0989083774764));
#60891=CARTESIAN_POINT('Ctrl Pts',(3.79963116547533,-38.2742356128,9.99378141045011));
#60892=CARTESIAN_POINT('Ctrl Pts',(3.9291794812562,-38.2742356128,9.88288657476412));
#60893=CARTESIAN_POINT('Ctrl Pts',(4.05373795681475,-38.2742356128,9.76663590776425));
#60894=CARTESIAN_POINT('Ctrl Pts',(4.17841478767598,-38.2742356128,9.65027477953067));
#60895=CARTESIAN_POINT('Ctrl Pts',(4.2980920856376,-38.2742356128,9.52854784101018));
#60896=CARTESIAN_POINT('Ctrl Pts',(4.41232768238676,-38.2742356128,9.40190718867832));
#60897=CARTESIAN_POINT('Ctrl Pts',(4.52652134987461,-38.2742356128,9.27531301878411));
#60898=CARTESIAN_POINT('Ctrl Pts',(4.63527711242045,-38.2742356128,9.14380895394925));
#60899=CARTESIAN_POINT('Ctrl Pts',(4.73819115171614,-38.2742356128,9.00788229232382));
#60900=CARTESIAN_POINT('Ctrl Pts',(4.77683663195496,-38.2742356128,8.95684016870565));
#60901=CARTESIAN_POINT('Ctrl Pts',(4.81465877164806,-38.2742356128,8.90517476127336));
#60902=CARTESIAN_POINT('Ctrl Pts',(4.85163765566323,-38.2742356128,8.85291307936199));
#60903=CARTESIAN_POINT('Ctrl Pts',(4.94954299698168,-38.2742356128,8.71454498249593));
#60904=CARTESIAN_POINT('Ctrl Pts',(5.04153458224144,-38.2742356128,8.57199450810618));
#60905=CARTESIAN_POINT('Ctrl Pts',(5.12727126160882,-38.2742356128,8.42578326478887));
#60906=CARTESIAN_POINT('Ctrl Pts',(5.21317959608459,-38.2742356128,8.27927928903775));
#60907=CARTESIAN_POINT('Ctrl Pts',(5.29280778803326,-38.2742356128,8.12910009662651));
#60908=CARTESIAN_POINT('Ctrl Pts',(5.3658589507314,-38.2742356128,7.97579537182009));
#60909=CARTESIAN_POINT('Ctrl Pts',(5.438330036196,-38.2742356128,7.82370799356053));
#60910=CARTESIAN_POINT('Ctrl Pts',(5.50432804704475,-38.2742356128,7.66854477968326));
#60911=CARTESIAN_POINT('Ctrl Pts',(5.56361038688553,-38.2742356128,7.51086328617028));
#60912=CARTESIAN_POINT('Ctrl Pts',(5.62264547171644,-38.2742356128,7.35383945123388));
#60913=CARTESIAN_POINT('Ctrl Pts',(5.67502067999286,-38.2742356128,7.19431853361871));
#60914=CARTESIAN_POINT('Ctrl Pts',(5.72054497528076,-38.2742356128,7.03286828206397));
#60915=CARTESIAN_POINT('Ctrl Pts',(5.76583911502499,-38.2742356128,6.87223426874395));
#60916=CARTESIAN_POINT('Ctrl Pts',(5.80435134203715,-38.2742356128,6.70969060885712));
#60917=CARTESIAN_POINT('Ctrl Pts',(5.83594316574969,-38.2742356128,6.545810032148));
#60918=CARTESIAN_POINT('Ctrl Pts',(5.86838176458437,-38.2742356128,6.37753686333587));
#60919=CARTESIAN_POINT('Ctrl Pts',(5.89352360761337,-38.2742356128,6.20785433630628));
#60920=CARTESIAN_POINT('Ctrl Pts',(5.91127539609655,-38.2742356128,6.03739372678238));
#60921=CARTESIAN_POINT('Ctrl Pts',(5.92829692245465,-38.2742356128,5.87394542067063));
#60922=CARTESIAN_POINT('Ctrl Pts',(5.9385241365587,-38.2742356128,5.70978199238531));
#60923=CARTESIAN_POINT('Ctrl Pts',(5.94192631696286,-38.2742356128,5.54546668994573));
#60924=CARTESIAN_POINT('Ctrl Pts',(5.94530777257515,-38.2742356128,5.38215233397002));
#60925=CARTESIAN_POINT('Ctrl Pts',(5.94194702074655,-38.2742356128,5.2186881472073));
#60926=CARTESIAN_POINT('Ctrl Pts',(5.93186515922344,-38.2742356128,5.05563062583815));
#60927=CARTESIAN_POINT('Ctrl Pts',(5.92187214024643,-38.2742356128,4.89400998647002));
#60928=CARTESIAN_POINT('Ctrl Pts',(5.90527590134661,-38.2742356128,4.73278906515281));
#60929=CARTESIAN_POINT('Ctrl Pts',(5.88214831546199,-38.2742356128,4.57251032877608));
#60930=CARTESIAN_POINT('Ctrl Pts',(5.87863513626286,-38.2742356128,4.54816330330133));
#60931=CARTESIAN_POINT('Ctrl Pts',(5.87497134477382,-38.2742356128,4.52383801660917));
#60932=CARTESIAN_POINT('Ctrl Pts',(5.87115729873963,-38.2742356128,4.49953636706381));
#60933=CARTESIAN_POINT('Ctrl Pts',(5.86945856588079,-38.2742356128,4.48871268789568));
#60934=CARTESIAN_POINT('Ctrl Pts',(5.86773011656,-38.2742356128,4.47789435759));
#60935=CARTESIAN_POINT('Ctrl Pts',(5.86597173001,-38.2742356128,4.46707975784));
#60936=CARTESIAN_POINT('',(-5.86597169341063,-38.2742356128,4.46707928635527));
#60937=CARTESIAN_POINT('Ctrl Pts',(-5.86597170737572,-38.2742356128,4.46707937224455));
#60938=CARTESIAN_POINT('Ctrl Pts',(-5.87355683913933,-38.2742356128,4.51373024197535));
#60939=CARTESIAN_POINT('Ctrl Pts',(-5.88058812630781,-38.2742356128,4.56047314614868));
#60940=CARTESIAN_POINT('Ctrl Pts',(-5.88706259142912,-38.2742356128,4.6072918885805));
#60941=CARTESIAN_POINT('Ctrl Pts',(-5.90124205880004,-38.2742356128,4.70982774570868));
#60942=CARTESIAN_POINT('Ctrl Pts',(-5.91275148943592,-38.2742356128,4.81273614246136));
#60943=CARTESIAN_POINT('Ctrl Pts',(-5.92157005802919,-38.2742356128,4.91587165229804));
#60944=CARTESIAN_POINT('Ctrl Pts',(-5.93542730978309,-38.2742356128,5.07793590450159));
#60945=CARTESIAN_POINT('Ctrl Pts',(-5.94263812513509,-38.2742356128,5.24056440725797));
#60946=CARTESIAN_POINT('Ctrl Pts',(-5.94316641713255,-38.2742356128,5.40320465831166));
#60947=CARTESIAN_POINT('Ctrl Pts',(-5.9436992161682,-38.2742356128,5.56723244850165));
#60948=CARTESIAN_POINT('Ctrl Pts',(-5.93743505163129,-38.2742356128,5.7312719950569));
#60949=CARTESIAN_POINT('Ctrl Pts',(-5.92438982488806,-38.2742356128,5.89476021211246));
#60950=CARTESIAN_POINT('Ctrl Pts',(-5.91123865175597,-38.2742356128,6.05957619345761));
#60951=CARTESIAN_POINT('Ctrl Pts',(-5.89119590289791,-38.2742356128,6.22383164873817));
#60952=CARTESIAN_POINT('Ctrl Pts',(-5.86433031406539,-38.2742356128,6.38695639973516));
#60953=CARTESIAN_POINT('Ctrl Pts',(-5.83716677560075,-38.2742356128,6.5518902664695));
#60954=CARTESIAN_POINT('Ctrl Pts',(-5.803028282697,-38.2742356128,6.71566798530386));
#60955=CARTESIAN_POINT('Ctrl Pts',(-5.76203826654907,-38.2742356128,6.87771032354166));
#60956=CARTESIAN_POINT('Ctrl Pts',(-5.72080339661986,-38.2742356128,7.04072062137001));
#60957=CARTESIAN_POINT('Ctrl Pts',(-5.67263501528278,-38.2742356128,7.20197451664067));
#60958=CARTESIAN_POINT('Ctrl Pts',(-5.6177101305643,-38.2742356128,7.36089593699001));
#60959=CARTESIAN_POINT('Ctrl Pts',(-5.56250554778591,-38.2742356128,7.52062664466291));
#60960=CARTESIAN_POINT('Ctrl Pts',(-5.50047559764723,-38.2742356128,7.67800082696959));
#60961=CARTESIAN_POINT('Ctrl Pts',(-5.43184993537474,-38.2742356128,7.8324507496487));
#60962=CARTESIAN_POINT('Ctrl Pts',(-5.36294537767596,-38.2742356128,7.98752835846738));
#60963=CARTESIAN_POINT('Ctrl Pts',(-5.28739152667286,-38.2742356128,8.13965765223937));
#60964=CARTESIAN_POINT('Ctrl Pts',(-5.20546906596608,-38.2742356128,8.288284788677));
#60965=CARTESIAN_POINT('Ctrl Pts',(-5.12322991732637,-38.2742356128,8.43748647353773));
#60966=CARTESIAN_POINT('Ctrl Pts',(-5.03457296952003,-38.2742356128,8.58315862728677));
#60967=CARTESIAN_POINT('Ctrl Pts',(-4.939828539296,-38.2742356128,8.72476556363208));
#60968=CARTESIAN_POINT('Ctrl Pts',(-4.84499408306954,-38.2742356128,8.86650705465637));
#60969=CARTESIAN_POINT('Ctrl Pts',(-4.74406073872847,-38.2742356128,9.00417536348988));
#60970=CARTESIAN_POINT('Ctrl Pts',(-4.63740374669067,-38.2742356128,9.13726147277406));
#60971=CARTESIAN_POINT('Ctrl Pts',(-4.53078590229245,-38.2742356128,9.27029873381173));
#60972=CARTESIAN_POINT('Ctrl Pts',(-4.41844878903217,-38.2742356128,9.39875692919792));
#60973=CARTESIAN_POINT('Ctrl Pts',(-4.30080854952501,-38.2742356128,9.52215924236615));
#60974=CARTESIAN_POINT('Ctrl Pts',(-4.25663325102553,-38.2742356128,9.56849826753789));
#60975=CARTESIAN_POINT('Ctrl Pts',(-4.21171056680681,-38.2742356128,9.61412470438002));
#60976=CARTESIAN_POINT('Ctrl Pts',(-4.16606395831939,-38.2742356128,9.65901455978178));
#60977=CARTESIAN_POINT('Ctrl Pts',(-4.04520980158801,-38.2742356128,9.77786513379252));
#60978=CARTESIAN_POINT('Ctrl Pts',(-3.91927805635973,-38.2742356128,9.8915501596496));
#60979=CARTESIAN_POINT('Ctrl Pts',(-3.78872879215426,-38.2742356128,9.99964916764474));
#60980=CARTESIAN_POINT('Ctrl Pts',(-3.65791815280783,-38.2742356128,10.1079646027));
#60981=CARTESIAN_POINT('Ctrl Pts',(-3.52247168238513,-38.2742356128,10.2106714302746));
#60982=CARTESIAN_POINT('Ctrl Pts',(-3.38288426840432,-38.2742356128,10.3073883619451));
#60983=CARTESIAN_POINT('Ctrl Pts',(-3.24440527586281,-38.2742356128,10.403337293711));
#60984=CARTESIAN_POINT('Ctrl Pts',(-3.10185108199932,-38.2742356128,10.4933909566946));
#60985=CARTESIAN_POINT('Ctrl Pts',(-2.95573306037451,-38.2742356128,10.5772203846891));
#60986=CARTESIAN_POINT('Ctrl Pts',(-2.81022446838551,-38.2742356128,10.6607001765661));
#60987=CARTESIAN_POINT('Ctrl Pts',(-2.66118192854463,-38.2742356128,10.7380074008848));
#60988=CARTESIAN_POINT('Ctrl Pts',(-2.50913515301595,-38.2742356128,10.8088623460546));
#60989=CARTESIAN_POINT('Ctrl Pts',(-2.35785707494213,-38.2742356128,10.8793590724076));
#60990=CARTESIAN_POINT('Ctrl Pts',(-2.20360527131204,-38.2742356128,10.9434684638986));
#60991=CARTESIAN_POINT('Ctrl Pts',(-2.04692280704148,-38.2742356128,11.0009618734306));
#60992=CARTESIAN_POINT('Ctrl Pts',(-1.8860406861784,-38.2742356128,11.0599963142292));
#60993=CARTESIAN_POINT('Ctrl Pts',(-1.72259597875071,-38.2742356128,11.1120549335068));
#60994=CARTESIAN_POINT('Ctrl Pts',(-1.55719679180931,-38.2742356128,11.156944290039));
#60995=CARTESIAN_POINT('Ctrl Pts',(-1.3986016946317,-38.2742356128,11.1999870159019));
#60996=CARTESIAN_POINT('Ctrl Pts',(-1.23820990933965,-38.2742356128,11.236438384511));
#60997=CARTESIAN_POINT('Ctrl Pts',(-1.07657244471484,-38.2742356128,11.266177642151));
#60998=CARTESIAN_POINT('Ctrl Pts',(-0.915919614215123,-38.2742356128,11.2957357395136));
#60999=CARTESIAN_POINT('Ctrl Pts',(-0.754036419195308,-38.2742356128,11.3186631496228));
#61000=CARTESIAN_POINT('Ctrl Pts',(-0.591475523881897,-38.2742356128,11.3348913497454));
#61001=CARTESIAN_POINT('Ctrl Pts',(-0.430347134286956,-38.2742356128,11.3509765450609));
#61002=CARTESIAN_POINT('Ctrl Pts',(-0.268553114665031,-38.2742356128,11.3604800062314));
#61003=CARTESIAN_POINT('Ctrl Pts',(-0.106640434026326,-38.2742356128,11.3633855794612));
#61004=CARTESIAN_POINT('Ctrl Pts',(-0.0820452052041727,-38.2742356128,11.3638269484643));
#61005=CARTESIAN_POINT('Ctrl Pts',(-0.0574472519929075,-38.2742356128,11.3641161688066));
#61006=CARTESIAN_POINT('Ctrl Pts',(-0.0328485055666778,-38.2742356128,11.364253288805));
#61007=CARTESIAN_POINT('Ctrl Pts',(-0.0218925028918889,-38.2742356128,11.3643143604971));
#61008=CARTESIAN_POINT('Ctrl Pts',(-0.0109370086389902,-38.2742356128,11.3643452424498));
#61009=CARTESIAN_POINT('Ctrl Pts',(1.96099429597E-5,-38.2742356128,11.3643459766));
#61010=CARTESIAN_POINT('',(-6.79137866102648,-38.2742356128,3.871800145837));
#61011=CARTESIAN_POINT('Ctrl Pts',(-6.79137822626605,-38.2742356128,3.87179985553789));
#61012=CARTESIAN_POINT('Ctrl Pts',(-6.7874746870692,-38.2742356128,3.86919337612066));
#61013=CARTESIAN_POINT('Ctrl Pts',(-6.78350177861248,-38.2742356128,3.86660738669588));
#61014=CARTESIAN_POINT('Ctrl Pts',(-6.77953817139297,-38.2742356127999,
3.86409312034724));
#61015=CARTESIAN_POINT('Ctrl Pts',(-6.77556131249333,-38.2742356127999,
3.86157044795541));
#61016=CARTESIAN_POINT('Ctrl Pts',(-6.77155434602956,-38.2742356127997,
3.85909408218151));
#61017=CARTESIAN_POINT('Ctrl Pts',(-6.76751880344076,-38.2742356127993,
3.8566650311283));
#61018=CARTESIAN_POINT('Ctrl Pts',(-6.74283132067483,-38.2742356127967,
3.84180528062534));
#61019=CARTESIAN_POINT('Ctrl Pts',(-6.71706303780477,-38.2742356127862,
3.82871283533343));
#61020=CARTESIAN_POINT('Ctrl Pts',(-6.69048236453115,-38.2742356127781,
3.81753794777997));
#61021=CARTESIAN_POINT('Ctrl Pts',(-6.66331896745911,-38.2742356127698,
3.8061180749752));
#61022=CARTESIAN_POINT('Ctrl Pts',(-6.63530751562895,-38.2742356127665,
3.79670075836635));
#61023=CARTESIAN_POINT('Ctrl Pts',(-6.60675061684617,-38.2742356127753,
3.78939456752495));
#61024=CARTESIAN_POINT('Ctrl Pts',(-6.59929698268323,-38.2742356127776,
3.78748757916214));
#61025=CARTESIAN_POINT('Ctrl Pts',(-6.59180625735376,-38.2742356127806,
3.78572414505303));
#61026=CARTESIAN_POINT('Ctrl Pts',(-6.58428395105746,-38.2742356127838,
3.78410563257977));
#61027=CARTESIAN_POINT('Ctrl Pts',(-6.55539473516567,-38.2742356127961,
3.77788977876823));
#61028=CARTESIAN_POINT('Ctrl Pts',(-6.52604419496571,-38.2742356127977,
3.773818071927));
#61029=CARTESIAN_POINT('Ctrl Pts',(-6.49655625119644,-38.2742356127986,
3.77193468945706));
#61030=CARTESIAN_POINT('Ctrl Pts',(-6.46668855933259,-38.2742356127994,
3.77002705263727));
#61031=CARTESIAN_POINT('Ctrl Pts',(-6.43668043247659,-38.2742356127996,
3.770364419042));
#61032=CARTESIAN_POINT('Ctrl Pts',(-6.40686989994023,-38.2742356127962,
3.77293917800287));
#61033=CARTESIAN_POINT('Ctrl Pts',(-6.38902711292706,-38.2742356127942,
3.77448027344265));
#61034=CARTESIAN_POINT('Ctrl Pts',(-6.37125510424854,-38.2742356127907,
3.7768218932986));
#61035=CARTESIAN_POINT('Ctrl Pts',(-6.35362537931003,-38.2742356127826,
3.77995354797865));
#61036=CARTESIAN_POINT('Ctrl Pts',(-6.32387247818031,-38.2742356127691,
3.78523870202347));
#61037=CARTESIAN_POINT('Ctrl Pts',(-6.29452471716957,-38.2742356127705,
3.79277482754427));
#61038=CARTESIAN_POINT('Ctrl Pts',(-6.26591393330974,-38.2742356127792,
3.80247248097018));
#61039=CARTESIAN_POINT('Ctrl Pts',(-6.23748120457973,-38.2742356127878,
3.8121097824341));
#61040=CARTESIAN_POINT('Ctrl Pts',(-6.20977683144767,-38.274235612797,3.82388158510264));
#61041=CARTESIAN_POINT('Ctrl Pts',(-6.1831074537671,-38.274235612799,3.83765256203365));
#61042=CARTESIAN_POINT('Ctrl Pts',(-6.1679998927991,-38.2742356128002,3.84545348922686));
#61043=CARTESIAN_POINT('Ctrl Pts',(-6.15322406734753,-38.2742356128,3.85389509364796));
#61044=CARTESIAN_POINT('Ctrl Pts',(-6.13883201163921,-38.2742356128,3.86294631787056));
#61045=CARTESIAN_POINT('Ctrl Pts',(-6.11359947122505,-38.2742356128,3.87881516841026));
#61046=CARTESIAN_POINT('Ctrl Pts',(-6.08954705620527,-38.2742356128,3.8965602905199));
#61047=CARTESIAN_POINT('Ctrl Pts',(-6.0669405737948,-38.2742356127994,3.91599348875386));
#61048=CARTESIAN_POINT('Ctrl Pts',(-6.0441163294935,-38.2742356127989,3.93561388152413));
#61049=CARTESIAN_POINT('Ctrl Pts',(-6.02276645828458,-38.2742356127977,
3.95695464194579));
#61050=CARTESIAN_POINT('Ctrl Pts',(-6.00313380480363,-38.2742356127976,
3.97977880667488));
#61051=CARTESIAN_POINT('Ctrl Pts',(-5.99197718539001,-38.2742356127975,
3.99274906153947));
#61052=CARTESIAN_POINT('Ctrl Pts',(-5.98137450999299,-38.2742356127978,
4.00619759615233));
#61053=CARTESIAN_POINT('Ctrl Pts',(-5.97136514237198,-38.2742356127985,
4.02007553453086));
#61054=CARTESIAN_POINT('Ctrl Pts',(-5.95374532527902,-38.2742356127997,
4.04450532321639));
#61055=CARTESIAN_POINT('Ctrl Pts',(-5.93796594671887,-38.2742356127998,
4.07026908063358));
#61056=CARTESIAN_POINT('Ctrl Pts',(-5.92421023426017,-38.2742356127999,
4.09707628881351));
#61057=CARTESIAN_POINT('Ctrl Pts',(-5.91061690032008,-38.2742356128,4.1235670528423));
#61058=CARTESIAN_POINT('Ctrl Pts',(-5.89900003626705,-38.2742356128,4.15107629598417));
#61059=CARTESIAN_POINT('Ctrl Pts',(-5.88949246037583,-38.2742356127999,
4.17929873891104));
#61060=CARTESIAN_POINT('Ctrl Pts',(-5.88395347814263,-38.2742356127999,
4.19574074386982));
#61061=CARTESIAN_POINT('Ctrl Pts',(-5.87912955562004,-38.2742356127999,
4.21242438372798));
#61062=CARTESIAN_POINT('Ctrl Pts',(-5.87503933051281,-38.2742356127998,
4.22928629342425));
#61063=CARTESIAN_POINT('Ctrl Pts',(-5.8681910328462,-38.2742356127997,4.25751832804343));
#61064=CARTESIAN_POINT('Ctrl Pts',(-5.86340476684082,-38.2742356127906,
4.28624903021261));
#61065=CARTESIAN_POINT('Ctrl Pts',(-5.86072552655069,-38.2742356127749,
4.31516978274542));
#61066=CARTESIAN_POINT('Ctrl Pts',(-5.85983219010252,-38.2742356127697,
4.32481280074619));
#61067=CARTESIAN_POINT('Ctrl Pts',(-5.85917268201552,-38.2742356127651,
4.33447687936722));
#61068=CARTESIAN_POINT('Ctrl Pts',(-5.8587473810514,-38.2742356127641,4.3441504118431));
#61069=CARTESIAN_POINT('Ctrl Pts',(-5.85747573494016,-38.2742356127609,
4.37307418816316));
#61070=CARTESIAN_POINT('Ctrl Pts',(-5.85830122916367,-38.2742356127925,
4.40208101771261));
#61071=CARTESIAN_POINT('Ctrl Pts',(-5.86120527939883,-38.2742356127979,
4.43086697454951));
#61072=CARTESIAN_POINT('Ctrl Pts',(-5.86218537575815,-38.2742356127998,
4.44058203083669));
#61073=CARTESIAN_POINT('Ctrl Pts',(-5.86340179293723,-38.2742356128,4.45027188757047));
#61074=CARTESIAN_POINT('Ctrl Pts',(-5.8648524612382,-38.2742356128,4.45992475891561));
#61075=CARTESIAN_POINT('Ctrl Pts',(-5.86521120069541,-38.2742356128,4.4623118420445));
#61076=CARTESIAN_POINT('Ctrl Pts',(-5.86558441248322,-38.2742356128,4.46469740146893));
#61077=CARTESIAN_POINT('Ctrl Pts',(-5.86597167956,-38.2742356128,4.46707920117));
#61078=CARTESIAN_POINT('',(-10.0697223221,-38.2742356128,2.85693798735));
#61079=CARTESIAN_POINT('Ctrl Pts',(-10.0697223221334,-38.2742356128,2.85693798737036));
#61080=CARTESIAN_POINT('Ctrl Pts',(-10.0633104414333,-38.2742356128,2.8674434550834));
#61081=CARTESIAN_POINT('Ctrl Pts',(-10.0568574951365,-38.2742356128007,
2.87794244256903));
#61082=CARTESIAN_POINT('Ctrl Pts',(-10.0503628618,-38.2742356127971,2.88843372499632));
#61083=CARTESIAN_POINT('Ctrl Pts',(-10.0215331036382,-38.2742356127809,
2.93500465818227));
#61084=CARTESIAN_POINT('Ctrl Pts',(-9.99182828957869,-38.2742356126542,
2.9815154431619));
#61085=CARTESIAN_POINT('Ctrl Pts',(-9.96120627016625,-38.274235611881,3.02776802419006));
#61086=CARTESIAN_POINT('Ctrl Pts',(-9.92616571750551,-38.2742356109961,
3.0806945140921));
#61087=CARTESIAN_POINT('Ctrl Pts',(-9.88992281642545,-38.2742356091384,
3.13328334536304));
#61088=CARTESIAN_POINT('Ctrl Pts',(-9.85233972844716,-38.2742356074002,
3.18522873807128));
#61089=CARTESIAN_POINT('Ctrl Pts',(-9.81179508152477,-38.2742356055251,
3.24126744377361));
#61090=CARTESIAN_POINT('Ctrl Pts',(-9.76968638910866,-38.2742356041571,
3.29655790872663));
#61091=CARTESIAN_POINT('Ctrl Pts',(-9.72580603199727,-38.274235605455,3.35069795220807));
#61092=CARTESIAN_POINT('Ctrl Pts',(-9.70965791715154,-38.2742356059326,
3.37062166517313));
#61093=CARTESIAN_POINT('Ctrl Pts',(-9.69327312413074,-38.2742356067395,
3.39038536076922));
#61094=CARTESIAN_POINT('Ctrl Pts',(-9.67664111106427,-38.274235607639,3.40997117451938));
#61095=CARTESIAN_POINT('Ctrl Pts',(-9.6600090979978,-38.2742356085385,3.42955698826954));
#61096=CARTESIAN_POINT('Ctrl Pts',(-9.64312794404234,-38.2742356094539,
3.44896763473112));
#61097=CARTESIAN_POINT('Ctrl Pts',(-9.62599170539255,-38.2742356102203,
3.46818060849546));
#61098=CARTESIAN_POINT('Ctrl Pts',(-9.59172981984717,-38.2742356117526,
3.50659468065872));
#61099=CARTESIAN_POINT('Ctrl Pts',(-9.55628350961246,-38.2742356123503,
3.54440198554242));
#61100=CARTESIAN_POINT('Ctrl Pts',(-9.51970351119237,-38.2742356126017,
3.58129418363479));
#61101=CARTESIAN_POINT('Ctrl Pts',(-9.4871353878986,-38.2742356128255,3.61414026641076));
#61102=CARTESIAN_POINT('Ctrl Pts',(-9.4536687089984,-38.2742356127996,3.64626067650308));
#61103=CARTESIAN_POINT('Ctrl Pts',(-9.41938694957581,-38.2742356128,3.67744527399227));
#61104=CARTESIAN_POINT('Ctrl Pts',(-9.41516398171632,-38.2742356128,3.68128672073031));
#61105=CARTESIAN_POINT('Ctrl Pts',(-9.41092870958514,-38.2742356128,3.68511398034174));
#61106=CARTESIAN_POINT('Ctrl Pts',(-9.40668134445996,-38.2742356128,3.68892667205413));
#61107=CARTESIAN_POINT('Ctrl Pts',(-9.38731105321667,-38.2742356128,3.70631461651221));
#61108=CARTESIAN_POINT('Ctrl Pts',(-9.3676655441854,-38.2742356128,3.72341953810915));
#61109=CARTESIAN_POINT('Ctrl Pts',(-9.34772272761063,-38.2742356128,3.74023552570305));
#61110=CARTESIAN_POINT('Ctrl Pts',(-9.32777991104666,-38.2742356128,3.75705151328784));
#61111=CARTESIAN_POINT('Ctrl Pts',(-9.30754898442837,-38.2742356128008,
3.77357031050439));
#61112=CARTESIAN_POINT('Ctrl Pts',(-9.2870412695087,-38.2742356127992,3.78976284024232));
#61113=CARTESIAN_POINT('Ctrl Pts',(-9.24453342509635,-38.2742356127959,
3.82332628392381));
#61114=CARTESIAN_POINT('Ctrl Pts',(-9.20083288838149,-38.2742356127424,
3.85548921994169));
#61115=CARTESIAN_POINT('Ctrl Pts',(-9.15603215791692,-38.2742356124498,
3.88604394693062));
#61116=CARTESIAN_POINT('Ctrl Pts',(-9.11383041795814,-38.2742356121741,
3.9148261259158));
#61117=CARTESIAN_POINT('Ctrl Pts',(-9.07065408929891,-38.2742356117035,
3.94218116564615));
#61118=CARTESIAN_POINT('Ctrl Pts',(-9.02661495058258,-38.2742356116231,
3.96795976616807));
#61119=CARTESIAN_POINT('Ctrl Pts',(-8.97306006550268,-38.2742356115254,
3.99930847163129));
#61120=CARTESIAN_POINT('Ctrl Pts',(-8.91820571108124,-38.2742356120678,
4.02834059887391));
#61121=CARTESIAN_POINT('Ctrl Pts',(-8.86221555378884,-38.2742356123975,
4.05487553259682));
#61122=CARTESIAN_POINT('Ctrl Pts',(-8.82327077478763,-38.2742356126268,
4.07333229677867));
#61123=CARTESIAN_POINT('Ctrl Pts',(-8.7837768881238,-38.2742356127455,4.09058175925433));
#61124=CARTESIAN_POINT('Ctrl Pts',(-8.74378271581823,-38.2742356127794,
4.10657708416326));
#61125=CARTESIAN_POINT('Ctrl Pts',(-8.69495943512302,-38.2742356128206,
4.12610353496397));
#61126=CARTESIAN_POINT('Ctrl Pts',(-8.64537775540928,-38.2742356128,4.14376462596244));
#61127=CARTESIAN_POINT('Ctrl Pts',(-8.5951696327512,-38.2742356128,4.1594740219235));
#61128=CARTESIAN_POINT('Ctrl Pts',(-8.54496151009177,-38.2742356128,4.17518341788498));
#61129=CARTESIAN_POINT('Ctrl Pts',(-8.4941169724322,-38.2742356128,4.18894526362599));
#61130=CARTESIAN_POINT('Ctrl Pts',(-8.44279988453127,-38.2742356128,4.2006885559872));
#61131=CARTESIAN_POINT('Ctrl Pts',(-8.38210007741659,-38.2742356128,4.21457896969487));
#61132=CARTESIAN_POINT('Ctrl Pts',(-8.32072862449063,-38.2742356128,4.22564662450852));
#61133=CARTESIAN_POINT('Ctrl Pts',(-8.25895938697734,-38.2742356128,4.23382180321406));
#61134=CARTESIAN_POINT('Ctrl Pts',(-8.19517547597314,-38.2742356128,4.24226362461239));
#61135=CARTESIAN_POINT('Ctrl Pts',(-8.13096964626072,-38.2742356128,4.24762123684602));
#61136=CARTESIAN_POINT('Ctrl Pts',(-8.06663542917861,-38.2742356128,4.24987419949773));
#61137=CARTESIAN_POINT('Ctrl Pts',(-8.0228271688435,-38.2742356128,4.25140835004541));
#61138=CARTESIAN_POINT('Ctrl Pts',(-7.97896315899794,-38.2742356128,4.25150389571578));
#61139=CARTESIAN_POINT('Ctrl Pts',(-7.93513432458635,-38.2742356128,4.25016834652164));
#61140=CARTESIAN_POINT('Ctrl Pts',(-7.8842940518043,-38.2742356128,4.24861914526508));
#61141=CARTESIAN_POINT('Ctrl Pts',(-7.83349885095115,-38.2742356128,4.24514493423103));
#61142=CARTESIAN_POINT('Ctrl Pts',(-7.78284834806656,-38.2742356128,4.23976656890104));
#61143=CARTESIAN_POINT('Ctrl Pts',(-7.73716457234106,-38.2742356128,4.23491559958164));
#61144=CARTESIAN_POINT('Ctrl Pts',(-7.69160498203115,-38.2742356128,4.22851414021581));
#61145=CARTESIAN_POINT('Ctrl Pts',(-7.64633824031241,-38.2742356128,4.22060655270573));
#61146=CARTESIAN_POINT('Ctrl Pts',(-7.5986399936733,-38.2742356128,4.21227420880257));
#61147=CARTESIAN_POINT('Ctrl Pts',(-7.55126746264243,-38.2742356128,4.20227103909697));
#61148=CARTESIAN_POINT('Ctrl Pts',(-7.50434329892817,-38.2742356128,4.19066324261345));
#61149=CARTESIAN_POINT('Ctrl Pts',(-7.48263553697715,-38.2742356128,4.18529331669693));
#61150=CARTESIAN_POINT('Ctrl Pts',(-7.46101470252345,-38.2742356128,4.17957805554725));
#61151=CARTESIAN_POINT('Ctrl Pts',(-7.43948853881381,-38.2742356128,4.17352310085893));
#61152=CARTESIAN_POINT('Ctrl Pts',(-7.37616575706325,-38.2742356128,4.15571144712398));
#61153=CARTESIAN_POINT('Ctrl Pts',(-7.31367164510924,-38.2742356128,4.13495923978566));
#61154=CARTESIAN_POINT('Ctrl Pts',(-7.2522425471246,-38.2742356128,4.11145109233569));
#61155=CARTESIAN_POINT('Ctrl Pts',(-7.19141311353757,-38.2742356128,4.08817242895015));
#61156=CARTESIAN_POINT('Ctrl Pts',(-7.13162842509448,-38.2742356128,4.06219174970784));
#61157=CARTESIAN_POINT('Ctrl Pts',(-7.07307992195391,-38.2742356128,4.03372160610396));
#61158=CARTESIAN_POINT('Ctrl Pts',(-7.02430271531214,-38.2742356128,4.01000291129202));
#61159=CARTESIAN_POINT('Ctrl Pts',(-6.9763829736138,-38.2742356128,3.98455703310644));
#61160=CARTESIAN_POINT('Ctrl Pts',(-6.9294076769401,-38.2742356128,3.95752201570169));
#61161=CARTESIAN_POINT('Ctrl Pts',(-6.90592002860325,-38.2742356128,3.94400450699932));
#61162=CARTESIAN_POINT('Ctrl Pts',(-6.88266813368041,-38.2742356128,3.93008991477376));
#61163=CARTESIAN_POINT('Ctrl Pts',(-6.85966059236408,-38.2742356128,3.91579662211982));
#61164=CARTESIAN_POINT('Ctrl Pts',(-6.84686917138494,-38.2742356128,3.90785003099994));
#61165=CARTESIAN_POINT('Ctrl Pts',(-6.83415325180026,-38.2742356128,3.89978639679546));
#61166=CARTESIAN_POINT('Ctrl Pts',(-6.82151409446459,-38.2742356128,3.89160896986944));
#61167=CARTESIAN_POINT('Ctrl Pts',(-6.81272250047702,-38.2742356128,3.88592088359223));
#61168=CARTESIAN_POINT('Ctrl Pts',(-6.80396727363108,-38.2742356128,3.8801772286737));
#61169=CARTESIAN_POINT('Ctrl Pts',(-6.79525123070431,-38.2742356128,3.87438074050389));
#61170=CARTESIAN_POINT('Ctrl Pts',(-6.79395950941247,-38.2742356128,3.87352169847648));
#61171=CARTESIAN_POINT('Ctrl Pts',(-6.79266874994473,-38.2742356128,3.87266156363026));
#61172=CARTESIAN_POINT('Ctrl Pts',(-6.79137909539,-38.2742356128,3.87180043587));
#61173=CARTESIAN_POINT('',(-10.7486857339,-38.2742356128,0.754197251045));
#61174=CARTESIAN_POINT('Ctrl Pts',(-10.748685733951,-38.2742356128,0.754197251052992));
#61175=CARTESIAN_POINT('Ctrl Pts',(-10.7467233592932,-38.2742356128,0.76671756222468));
#61176=CARTESIAN_POINT('Ctrl Pts',(-10.7447502486204,-38.2742356128,0.779205465261789));
#61177=CARTESIAN_POINT('Ctrl Pts',(-10.742753142554,-38.2742356128,0.791748410472544));
#61178=CARTESIAN_POINT('Ctrl Pts',(-10.7424571718059,-38.2742356128,0.793607272623299));
#61179=CARTESIAN_POINT('Ctrl Pts',(-10.7421606885948,-38.2742356128,0.795467251786625));
#61180=CARTESIAN_POINT('Ctrl Pts',(-10.7418636644767,-38.2742356128,0.797328539574165));
#61181=CARTESIAN_POINT('Ctrl Pts',(-10.7397289995216,-38.2742356128,0.810705317986936));
#61182=CARTESIAN_POINT('Ctrl Pts',(-10.7375655067097,-38.2742356128,0.824156020876981));
#61183=CARTESIAN_POINT('Ctrl Pts',(-10.7353677682444,-38.2742356127999,
0.83771928337193));
#61184=CARTESIAN_POINT('Ctrl Pts',(-10.7328906315049,-38.2742356127998,
0.85300684208891));
#61185=CARTESIAN_POINT('Ctrl Pts',(-10.7303700221984,-38.2742356127996,
0.868437268995491));
#61186=CARTESIAN_POINT('Ctrl Pts',(-10.7278087378651,-38.2742356127991,
0.883997963310959));
#61187=CARTESIAN_POINT('Ctrl Pts',(-10.7248377347222,-38.2742356127985,
0.90204784208249));
#61188=CARTESIAN_POINT('Ctrl Pts',(-10.72181220956,-38.2742356127974,0.920271904703645));
#61189=CARTESIAN_POINT('Ctrl Pts',(-10.7187482319499,-38.2742356127961,
0.938572490763118));
#61190=CARTESIAN_POINT('Ctrl Pts',(-10.7149229765464,-38.2742356127944,
0.961420051880341));
#61191=CARTESIAN_POINT('Ctrl Pts',(-10.7110388540621,-38.2742356127923,
0.984380955081967));
#61192=CARTESIAN_POINT('Ctrl Pts',(-10.7071345609069,-38.2742356127909,
1.00720366640169));
#61193=CARTESIAN_POINT('Ctrl Pts',(-10.7042498808607,-38.27423561279,1.02406618602461));
#61194=CARTESIAN_POINT('Ctrl Pts',(-10.7013545207682,-38.2742356127895,
1.0408508782088));
#61195=CARTESIAN_POINT('Ctrl Pts',(-10.6984588552136,-38.27423561279,1.05748168729192));
#61196=CARTESIAN_POINT('Ctrl Pts',(-10.6958462069106,-38.2742356127904,
1.07248703038407));
#61197=CARTESIAN_POINT('Ctrl Pts',(-10.6932334434059,-38.2742356127916,
1.08736621956575));
#61198=CARTESIAN_POINT('Ctrl Pts',(-10.6906206945055,-38.2742356127934,
1.10210512196072));
#61199=CARTESIAN_POINT('Ctrl Pts',(-10.6882215637706,-38.274235612795,1.11563897273773));
#61200=CARTESIAN_POINT('Ctrl Pts',(-10.6858224949344,-38.2742356127971,
1.12905419587582));
#61201=CARTESIAN_POINT('Ctrl Pts',(-10.6834157727329,-38.2742356127986,
1.1423847022234));
#61202=CARTESIAN_POINT('Ctrl Pts',(-10.6828674279457,-38.2742356127989,
1.14542190928546));
#61203=CARTESIAN_POINT('Ctrl Pts',(-10.6823186498546,-38.2742356127992,
1.14845492720555));
#61204=CARTESIAN_POINT('Ctrl Pts',(-10.6817692804452,-38.2742356127994,
1.15148454459705));
#61205=CARTESIAN_POINT('Ctrl Pts',(-10.6795353563807,-38.2742356128004,
1.16380400593097));
#61206=CARTESIAN_POINT('Ctrl Pts',(-10.6772801001843,-38.2742356128,1.17613331617475));
#61207=CARTESIAN_POINT('Ctrl Pts',(-10.6750013200392,-38.2742356128,1.18847758722424));
#61208=CARTESIAN_POINT('Ctrl Pts',(-10.6746215084719,-38.2742356128,1.19053504631933));
#61209=CARTESIAN_POINT('Ctrl Pts',(-10.6742410257375,-38.2742356128,1.19259303749411));
#61210=CARTESIAN_POINT('Ctrl Pts',(-10.6738598407567,-38.2742356128,1.19465172326413));
#61211=CARTESIAN_POINT('Ctrl Pts',(-10.6710364362196,-38.2742356128,1.20990023261282));
#61212=CARTESIAN_POINT('Ctrl Pts',(-10.6681670600522,-38.2742356128,1.22522670900423));
#61213=CARTESIAN_POINT('Ctrl Pts',(-10.6652585665919,-38.2742356128,1.24056634443058));
#61214=CARTESIAN_POINT('Ctrl Pts',(-10.6620395305332,-38.2742356128,1.25754380724367));
#61215=CARTESIAN_POINT('Ctrl Pts',(-10.6587724492008,-38.2742356128,1.27453816301365));
#61216=CARTESIAN_POINT('Ctrl Pts',(-10.6554555858017,-38.2742356128,1.29152616786436));
#61217=CARTESIAN_POINT('Ctrl Pts',(-10.6511604363153,-38.2742356128,1.31352466811263));
#61218=CARTESIAN_POINT('Ctrl Pts',(-10.646781470819,-38.2742356128,1.33551458505531));
#61219=CARTESIAN_POINT('Ctrl Pts',(-10.6423001074962,-38.2742356128,1.3575313458063));
#61220=CARTESIAN_POINT('Ctrl Pts',(-10.6384602262308,-38.2742356128,1.37639653058204));
#61221=CARTESIAN_POINT('Ctrl Pts',(-10.6345444130273,-38.2742356128,1.39528583945895));
#61222=CARTESIAN_POINT('Ctrl Pts',(-10.6305412850362,-38.2742356128,1.41421856465516));
#61223=CARTESIAN_POINT('Ctrl Pts',(-10.6276006111313,-38.2742356128,1.42812643146691));
#61224=CARTESIAN_POINT('Ctrl Pts',(-10.6246127952894,-38.2742356128,1.44205784892357));
#61225=CARTESIAN_POINT('Ctrl Pts',(-10.6215764121983,-38.2742356128,1.45600181465977));
#61226=CARTESIAN_POINT('Ctrl Pts',(-10.6122522885066,-38.2742356128,1.49882093773288));
#61227=CARTESIAN_POINT('Ctrl Pts',(-10.6024753861189,-38.2742356127986,
1.54173415070471));
#61228=CARTESIAN_POINT('Ctrl Pts',(-10.5921655850875,-38.2742356127461,
1.58468657520376));
#61229=CARTESIAN_POINT('Ctrl Pts',(-10.588366873773,-38.2742356127268,1.60051266733034));
#61230=CARTESIAN_POINT('Ctrl Pts',(-10.5844959048361,-38.2742356127021,
1.61634467614605));
#61231=CARTESIAN_POINT('Ctrl Pts',(-10.5805488316998,-38.2742356126787,
1.63218139868328));
#61232=CARTESIAN_POINT('Ctrl Pts',(-10.5673420237974,-38.2742356126001,
1.68517067583315));
#61233=CARTESIAN_POINT('Ctrl Pts',(-10.5532662440154,-38.2742356127979,
1.73824876968933));
#61234=CARTESIAN_POINT('Ctrl Pts',(-10.5381979081127,-38.2742356127998,
1.79134448248764));
#61235=CARTESIAN_POINT('Ctrl Pts',(-10.5365404194269,-38.2742356128,1.79718491130464));
#61236=CARTESIAN_POINT('Ctrl Pts',(-10.534870891996,-38.2742356128,1.80302550347159));
#61237=CARTESIAN_POINT('Ctrl Pts',(-10.5331891355497,-38.2742356128,1.8088661121043));
#61238=CARTESIAN_POINT('Ctrl Pts',(-10.5223070013948,-38.2742356128,1.84665891309219));
#61239=CARTESIAN_POINT('Ctrl Pts',(-10.5109029235634,-38.2742356128,1.88447164217536));
#61240=CARTESIAN_POINT('Ctrl Pts',(-10.4989800247135,-38.2742356128,1.9221950930079));
#61241=CARTESIAN_POINT('Ctrl Pts',(-10.4853933388155,-38.2742356128,1.96518268217577));
#61242=CARTESIAN_POINT('Ctrl Pts',(-10.4711323192743,-38.2742356128,2.00805437618363));
#61243=CARTESIAN_POINT('Ctrl Pts',(-10.456177188935,-38.2742356128,2.05071523903541));
#61244=CARTESIAN_POINT('Ctrl Pts',(-10.4401159541856,-38.2742356128,2.09653136482825));
#61245=CARTESIAN_POINT('Ctrl Pts',(-10.4232523167762,-38.2742356128,2.142106292031));
#61246=CARTESIAN_POINT('Ctrl Pts',(-10.405554623622,-38.2742356128,2.18737956628733));
#61247=CARTESIAN_POINT('Ctrl Pts',(-10.386182665736,-38.2742356128,2.23693585334798));
#61248=CARTESIAN_POINT('Ctrl Pts',(-10.3658081590339,-38.2742356128,2.2861351960916));
#61249=CARTESIAN_POINT('Ctrl Pts',(-10.3444057568216,-38.2742356128,2.33495675618703));
#61250=CARTESIAN_POINT('Ctrl Pts',(-10.3267437697895,-38.2742356128,2.37524596076966));
#61251=CARTESIAN_POINT('Ctrl Pts',(-10.308380690975,-38.2742356128292,2.4152812514512));
#61252=CARTESIAN_POINT('Ctrl Pts',(-10.2893404343762,-38.2742356127708,
2.45504116755052));
#61253=CARTESIAN_POINT('Ctrl Pts',(-10.281341785723,-38.2742356127462,2.47174396762627));
#61254=CARTESIAN_POINT('Ctrl Pts',(-10.2732241195849,-38.2742356127022,
2.48839790173856));
#61255=CARTESIAN_POINT('Ctrl Pts',(-10.2649916475408,-38.2742356125604,
2.50499979826043));
#61256=CARTESIAN_POINT('Ctrl Pts',(-10.2479974939845,-38.2742356122679,
2.53927081397805));
#61257=CARTESIAN_POINT('Ctrl Pts',(-10.2305030891973,-38.2742356119712,
2.5733197530435));
#61258=CARTESIAN_POINT('Ctrl Pts',(-10.2125691285345,-38.274235611949,2.60709854992017));
#61259=CARTESIAN_POINT('Ctrl Pts',(-10.1954390335978,-38.2742356119277,
2.63936325754504));
#61260=CARTESIAN_POINT('Ctrl Pts',(-10.1779076823657,-38.2742356121028,
2.67138189744662));
#61261=CARTESIAN_POINT('Ctrl Pts',(-10.1600624624965,-38.27423561229,2.703082197551));
#61262=CARTESIAN_POINT('Ctrl Pts',(-10.1431808811642,-38.2742356124672,
2.73307068737573));
#61263=CARTESIAN_POINT('Ctrl Pts',(-10.1260183450808,-38.2742356126392,
2.7627744857011));
#61264=CARTESIAN_POINT('Ctrl Pts',(-10.1086823197939,-38.2742356127228,
2.79210055954277));
#61265=CARTESIAN_POINT('Ctrl Pts',(-10.0979357011284,-38.2742356127746,
2.8102798207816));
#61266=CARTESIAN_POINT('Ctrl Pts',(-10.0871230781097,-38.2742356127961,
2.82831329245778));
#61267=CARTESIAN_POINT('Ctrl Pts',(-10.0762772719591,-38.2742356127995,
2.846171629031));
#61268=CARTESIAN_POINT('Ctrl Pts',(-10.0740935067996,-38.2742356128001,
2.84976734268047));
#61269=CARTESIAN_POINT('Ctrl Pts',(-10.0719070834333,-38.2742356128,2.85335838651667));
#61270=CARTESIAN_POINT('Ctrl Pts',(-10.0697223221,-38.2742356128,2.85693798735));
#61271=CARTESIAN_POINT('',(-1.34538288120071,-38.2742356128,-9.83573535821205));
#61272=CARTESIAN_POINT('Ctrl Pts',(-1.34538313247,-38.2742356128,-9.83573533307));
#61273=CARTESIAN_POINT('Ctrl Pts',(-1.36959257784029,-38.2742356128,-9.83234472937659));
#61274=CARTESIAN_POINT('Ctrl Pts',(-1.39358213876267,-38.2742356128,-9.82897090867581));
#61275=CARTESIAN_POINT('Ctrl Pts',(-1.41743559841733,-38.2742356128,-9.82559963885233));
#61276=CARTESIAN_POINT('Ctrl Pts',(-1.44325409530112,-38.2742356128,-9.82195064534396));
#61277=CARTESIAN_POINT('Ctrl Pts',(-1.46891304898785,-38.2742356128,-9.81830465474449));
#61278=CARTESIAN_POINT('Ctrl Pts',(-1.49445697405912,-38.2742356128,-9.81465207203634));
#61279=CARTESIAN_POINT('Ctrl Pts',(-1.52191069053112,-38.2742356128,-9.81072640400451));
#61280=CARTESIAN_POINT('Ctrl Pts',(-1.54923100158245,-38.2742356128,-9.80679319694156));
#61281=CARTESIAN_POINT('Ctrl Pts',(-1.57640956213349,-38.2742356128,-9.80284921566262));
#61282=CARTESIAN_POINT('Ctrl Pts',(-1.6070765377458,-38.2742356128,-9.79839901759309));
#61283=CARTESIAN_POINT('Ctrl Pts',(-1.63756215570723,-38.2742356128,-9.79393522891224));
#61284=CARTESIAN_POINT('Ctrl Pts',(-1.6677866639062,-38.2742356128,-9.78946237139186));
#61285=CARTESIAN_POINT('Ctrl Pts',(-1.71351404398834,-38.2742356128,-9.78269527845716));
#61286=CARTESIAN_POINT('Ctrl Pts',(-1.75863901101848,-38.2742356128,-9.77590814500956));
#61287=CARTESIAN_POINT('Ctrl Pts',(-1.8027616949637,-38.2742356128,-9.76913273533593));
#61288=CARTESIAN_POINT('Ctrl Pts',(-1.83164853545357,-38.2742356128,-9.76469691772478));
#61289=CARTESIAN_POINT('Ctrl Pts',(-1.86010274514465,-38.2742356128,-9.76026651943909));
#61290=CARTESIAN_POINT('Ctrl Pts',(-1.88803424909477,-38.2742356128,-9.75584709271156));
#61291=CARTESIAN_POINT('Ctrl Pts',(-1.90276621750807,-38.2742356128,-9.75351614572527));
#61292=CARTESIAN_POINT('Ctrl Pts',(-1.91735339380267,-38.2742356128,-9.75118816150423));
#61293=CARTESIAN_POINT('Ctrl Pts',(-1.93178873575302,-38.2742356128,-9.74886307273491));
#61294=CARTESIAN_POINT('Ctrl Pts',(-1.9542416630588,-38.2742356128,-9.74524659802329));
#61295=CARTESIAN_POINT('Ctrl Pts',(-1.97633365589926,-38.2742356128,-9.74163600882343));
#61296=CARTESIAN_POINT('Ctrl Pts',(-1.99822346015992,-38.2742356128,-9.73800258624781));
#61297=CARTESIAN_POINT('Ctrl Pts',(-2.02071725826659,-38.2742356128,-9.73426890855571));
#61298=CARTESIAN_POINT('Ctrl Pts',(-2.04299696927202,-38.2742356128,-9.73051122797212));
#61299=CARTESIAN_POINT('Ctrl Pts',(-2.06517301875635,-38.2742356128,-9.72670961912013));
#61300=CARTESIAN_POINT('Ctrl Pts',(-2.08884787124812,-38.2742356128,-9.72265107258477));
#61301=CARTESIAN_POINT('Ctrl Pts',(-2.1124040946237,-38.2742356128,-9.71854254870478));
#61302=CARTESIAN_POINT('Ctrl Pts',(-2.13591439660367,-38.2742356128,-9.71437098329188));
#61303=CARTESIAN_POINT('Ctrl Pts',(-2.1619581216413,-38.2742356128,-9.70974989834442));
#61304=CARTESIAN_POINT('Ctrl Pts',(-2.1879447425657,-38.2742356128,-9.70505159407837));
#61305=CARTESIAN_POINT('Ctrl Pts',(-2.21390903684172,-38.2742356128,-9.70026987667837));
#61306=CARTESIAN_POINT('Ctrl Pts',(-2.25014620370348,-38.2742356128,-9.69359625445443));
#61307=CARTESIAN_POINT('Ctrl Pts',(-2.28633804663903,-38.2742356128,-9.68676051999743));
#61308=CARTESIAN_POINT('Ctrl Pts',(-2.32247055514705,-38.2742356128,-9.67976513651878));
#61309=CARTESIAN_POINT('Ctrl Pts',(-2.35165394779118,-38.2742356128,-9.67411512684098));
#61310=CARTESIAN_POINT('Ctrl Pts',(-2.38079361486408,-38.2742356128,-9.66836187808848));
#61311=CARTESIAN_POINT('Ctrl Pts',(-2.40988939653965,-38.2742356128,-9.66250503837571));
#61312=CARTESIAN_POINT('Ctrl Pts',(-2.4225086275498,-38.2742356128,-9.65996484838703));
#61313=CARTESIAN_POINT('Ctrl Pts',(-2.43512007479769,-38.2742356128,-9.65740508209448));
#61314=CARTESIAN_POINT('Ctrl Pts',(-2.44772709713684,-38.2742356128,-9.65482507591868));
#61315=CARTESIAN_POINT('Ctrl Pts',(-2.56020547209503,-38.2742356128,-9.63180656336037));
#61316=CARTESIAN_POINT('Ctrl Pts',(-2.67234639159194,-38.2742356128,-9.6071728357461));
#61317=CARTESIAN_POINT('Ctrl Pts',(-2.78403077108086,-38.2742356128,-9.58090883358199));
#61318=CARTESIAN_POINT('Ctrl Pts',(-2.9120337603626,-38.2742356128,-9.55080730279592));
#61319=CARTESIAN_POINT('Ctrl Pts',(-3.03943743362999,-38.2742356128,-9.51856418783258));
#61320=CARTESIAN_POINT('Ctrl Pts',(-3.16613185998554,-38.2742356128,-9.48416597085791));
#61321=CARTESIAN_POINT('Ctrl Pts',(-3.33071450491481,-38.2742356128,-9.43948089911959));
#61322=CARTESIAN_POINT('Ctrl Pts',(-3.49410236255372,-38.2742356128,-9.39115857075402));
#61323=CARTESIAN_POINT('Ctrl Pts',(-3.65615113873269,-38.2742356128,-9.33918912043045));
#61324=CARTESIAN_POINT('Ctrl Pts',(-3.7213143204076,-38.2742356128,-9.31829112408125));
#61325=CARTESIAN_POINT('Ctrl Pts',(-3.78626160561947,-38.2742356128,-9.29680360387223));
#61326=CARTESIAN_POINT('Ctrl Pts',(-3.85098428964021,-38.2742356128,-9.27472670369517));
#61327=CARTESIAN_POINT('Ctrl Pts',(-3.95865102485678,-38.2742356128,-9.23800159252698));
#61328=CARTESIAN_POINT('Ctrl Pts',(-4.06569998469652,-38.2742356128,-9.1996429145904));
#61329=CARTESIAN_POINT('Ctrl Pts',(-4.17210492639527,-38.2742356128,-9.15965461239092));
#61330=CARTESIAN_POINT('Ctrl Pts',(-4.31210622633393,-38.2742356128,-9.10704038037415));
#61331=CARTESIAN_POINT('Ctrl Pts',(-4.45098794296568,-38.2742356128,-9.05160623665064));
#61332=CARTESIAN_POINT('Ctrl Pts',(-4.58863476770087,-38.2742356128,-8.99341240511538));
#61333=CARTESIAN_POINT('Ctrl Pts',(-4.6795968534866,-38.2742356128,-8.95495578029679));
#61334=CARTESIAN_POINT('Ctrl Pts',(-4.77001840222156,-38.2742356128,-8.91529515967408));
#61335=CARTESIAN_POINT('Ctrl Pts',(-4.85988107462834,-38.2742356128,-8.87444749686709));
#61336=CARTESIAN_POINT('Ctrl Pts',(-5.02694237423458,-38.2742356128,-8.79850869545327));
#61337=CARTESIAN_POINT('Ctrl Pts',(-5.19207696240372,-38.2742356128,-8.71846212306564));
#61338=CARTESIAN_POINT('Ctrl Pts',(-5.35517439119676,-38.2742356128,-8.6344774086833));
#61339=CARTESIAN_POINT('Ctrl Pts',(-5.49157233846693,-38.2742356128,-8.56424121471878));
#61340=CARTESIAN_POINT('Ctrl Pts',(-5.62654463760369,-38.2742356128,-8.49125208831812));
#61341=CARTESIAN_POINT('Ctrl Pts',(-5.76006044505498,-38.2742356128,-8.41562097191507));
#61342=CARTESIAN_POINT('Ctrl Pts',(-5.88434039844082,-38.2742356128,-8.34522158025862));
#61343=CARTESIAN_POINT('Ctrl Pts',(-6.00735775169599,-38.2742356128,-8.27253364803918));
#61344=CARTESIAN_POINT('Ctrl Pts',(-6.12912965309513,-38.2742356128,-8.19764585212784));
#61345=CARTESIAN_POINT('Ctrl Pts',(-6.24138886497924,-38.2742356128,-8.12860821001047));
#61346=CARTESIAN_POINT('Ctrl Pts',(-6.35258942208878,-38.2742356128,-8.05770128566654));
#61347=CARTESIAN_POINT('Ctrl Pts',(-6.46278702258669,-38.2742356128,-7.98498804904817));
#61348=CARTESIAN_POINT('Ctrl Pts',(-6.56530437260463,-38.2742356128,-7.91734258040219));
#61349=CARTESIAN_POINT('Ctrl Pts',(-6.66695365169245,-38.2742356128,-7.84813396875634));
#61350=CARTESIAN_POINT('Ctrl Pts',(-6.76781933890444,-38.2742356128,-7.7774039677487));
#61351=CARTESIAN_POINT('Ctrl Pts',(-6.85248887582691,-38.2742356128,-7.71803118600919));
#61352=CARTESIAN_POINT('Ctrl Pts',(-6.93661315853148,-38.2742356128,-7.65758405631927));
#61353=CARTESIAN_POINT('Ctrl Pts',(-7.02025404496547,-38.2742356128,-7.59605079899767));
#61354=CARTESIAN_POINT('Ctrl Pts',(-7.10707098904692,-38.2742356128,-7.53218096705544));
#61355=CARTESIAN_POINT('Ctrl Pts',(-7.19336693513277,-38.2742356128,-7.46714123578346));
#61356=CARTESIAN_POINT('Ctrl Pts',(-7.2791559123188,-38.2742356128,-7.40093769788929));
#61357=CARTESIAN_POINT('Ctrl Pts',(-7.36884947222418,-38.2742356128,-7.33172098512697));
#61358=CARTESIAN_POINT('Ctrl Pts',(-7.45798861557288,-38.2742356128,-7.26123249546362));
#61359=CARTESIAN_POINT('Ctrl Pts',(-7.5465335522818,-38.2742356128,-7.18949473649223));
#61360=CARTESIAN_POINT('Ctrl Pts',(-7.64317344207319,-38.2742356128,-7.11119856983884));
#61361=CARTESIAN_POINT('Ctrl Pts',(-7.73910544090864,-38.2742356128,-7.03141483703542));
#61362=CARTESIAN_POINT('Ctrl Pts',(-7.83421469437285,-38.2742356128,-6.95018353462036));
#61363=CARTESIAN_POINT('Ctrl Pts',(-7.93533493965101,-38.2742356128,-6.86381833959162));
#61364=CARTESIAN_POINT('Ctrl Pts',(-8.03552442437534,-38.2742356128,-6.77581783862214));
#61365=CARTESIAN_POINT('Ctrl Pts',(-8.13458343720895,-38.2742356128,-6.68622895146722));
#61366=CARTESIAN_POINT('Ctrl Pts',(-8.24082633690025,-38.2742356128,-6.59014296313374));
#61367=CARTESIAN_POINT('Ctrl Pts',(-8.34576756691707,-38.2742356128,-6.4922315231506));
#61368=CARTESIAN_POINT('Ctrl Pts',(-8.44910778731491,-38.2742356128,-6.39252971936197));
#61369=CARTESIAN_POINT('Ctrl Pts',(-8.47511576604178,-38.2742356128,-6.36743743310612));
#61370=CARTESIAN_POINT('Ctrl Pts',(-8.50102215119995,-38.2742356128,-6.34223156598619));
#61371=CARTESIAN_POINT('Ctrl Pts',(-8.52682186017411,-38.2742356128,-6.31691226462336));
#61372=CARTESIAN_POINT('Ctrl Pts',(-8.60961626803044,-38.2742356128,-6.23565954329336));
#61373=CARTESIAN_POINT('Ctrl Pts',(-8.69131691175532,-38.2742356128,-6.15323856599964));
#61374=CARTESIAN_POINT('Ctrl Pts',(-8.77180401686034,-38.2742356128,-6.06959560014329));
#61375=CARTESIAN_POINT('Ctrl Pts',(-8.85668253824117,-38.2742356128,-5.98138903268718));
#61376=CARTESIAN_POINT('Ctrl Pts',(-8.94021107931082,-38.2742356128,-5.89182312662737));
#61377=CARTESIAN_POINT('Ctrl Pts',(-9.02218699302706,-38.2742356128,-5.80083647024894));
#61378=CARTESIAN_POINT('Ctrl Pts',(-9.10978693087572,-38.2742356128,-5.70360760042021));
#61379=CARTESIAN_POINT('Ctrl Pts',(-9.19561326069119,-38.2742356128,-5.60475576571228));
#61380=CARTESIAN_POINT('Ctrl Pts',(-9.27935754613207,-38.2742356128,-5.50421539201818));
#61381=CARTESIAN_POINT('Ctrl Pts',(-9.37333346090317,-38.2742356128,-5.39139129256366));
#61382=CARTESIAN_POINT('Ctrl Pts',(-9.46468648696409,-38.2742356128,-5.27643956006855));
#61383=CARTESIAN_POINT('Ctrl Pts',(-9.55291854354469,-38.2742356128,-5.15929424499621));
#61384=CARTESIAN_POINT('Ctrl Pts',(-9.64137851939688,-38.2742356128,-5.04184632250526));
#61385=CARTESIAN_POINT('Ctrl Pts',(-9.72669884147059,-38.2742356128,-4.92219249370742));
#61386=CARTESIAN_POINT('Ctrl Pts',(-9.80834822171838,-38.2742356128,-4.80030871896846));
#61387=CARTESIAN_POINT('Ctrl Pts',(-9.88177596113607,-38.2742356128,-4.69069796597051));
#61388=CARTESIAN_POINT('Ctrl Pts',(-9.95223315159215,-38.2742356128,-4.57928380474877));
#61389=CARTESIAN_POINT('Ctrl Pts',(-10.0193388107923,-38.2742356128,-4.4660877450883));
#61390=CARTESIAN_POINT('Ctrl Pts',(-10.0741971857383,-38.2742356128,-4.37355081217879));
#61391=CARTESIAN_POINT('Ctrl Pts',(-10.1268155003064,-38.2742356128,-4.27982359904656));
#61392=CARTESIAN_POINT('Ctrl Pts',(-10.1769991523961,-38.2742356128,-4.18494031390587));
#61393=CARTESIAN_POINT('Ctrl Pts',(-10.2227626539552,-38.2742356128,-4.0984143002212));
#61394=CARTESIAN_POINT('Ctrl Pts',(-10.2665046430741,-38.2742356128,-4.01092417744194));
#61395=CARTESIAN_POINT('Ctrl Pts',(-10.30814198582,-38.2742356128,-3.92251508690199));
#61396=CARTESIAN_POINT('Ctrl Pts',(-10.35470936117,-38.2742356128,-3.82363799648239));
#61397=CARTESIAN_POINT('Ctrl Pts',(-10.3986412352236,-38.2742356128,-3.72361213751219));
#61398=CARTESIAN_POINT('Ctrl Pts',(-10.4398160136821,-38.2742356128,-3.62255987753841));
#61399=CARTESIAN_POINT('Ctrl Pts',(-10.477385766401,-38.2742356128,-3.53035516968021));
#61400=CARTESIAN_POINT('Ctrl Pts',(-10.5126579933682,-38.2742356128,-3.43729780988155));
#61401=CARTESIAN_POINT('Ctrl Pts',(-10.5455730499076,-38.2742356128,-3.34350507155265));
#61402=CARTESIAN_POINT('Ctrl Pts',(-10.5745613901557,-38.2742356128,-3.26090166456049));
#61403=CARTESIAN_POINT('Ctrl Pts',(-10.6017209066368,-38.2742356128,-3.17772876645298));
#61404=CARTESIAN_POINT('Ctrl Pts',(-10.6270526045767,-38.2742356128,-3.09406894779799));
#61405=CARTESIAN_POINT('Ctrl Pts',(-10.6356138257324,-38.2742356128,-3.06579487745959));
#61406=CARTESIAN_POINT('Ctrl Pts',(-10.6439666896209,-38.2742356128,-3.03746516058653));
#61407=CARTESIAN_POINT('Ctrl Pts',(-10.652112636549,-38.2742356128,-3.00908281936168));
#61408=CARTESIAN_POINT('Ctrl Pts',(-10.6798118244882,-38.2742356128,-2.91257251666922));
#61409=CARTESIAN_POINT('Ctrl Pts',(-10.7051257417243,-38.2742356131574,
-2.81545484897836));
#61410=CARTESIAN_POINT('Ctrl Pts',(-10.7280634120543,-38.2742356113512,
-2.71781791747719));
#61411=CARTESIAN_POINT('Ctrl Pts',(-10.7519843914305,-38.2742356094676,
-2.61599541365775));
#61412=CARTESIAN_POINT('Ctrl Pts',(-10.7733212964808,-38.2742356048073,
-2.51360839689941));
#61413=CARTESIAN_POINT('Ctrl Pts',(-10.7921397632951,-38.2742355939441,
-2.41077097878834));
#61414=CARTESIAN_POINT('Ctrl Pts',(-10.8125905501039,-38.2742355821387,
-2.29901340924145));
#61415=CARTESIAN_POINT('Ctrl Pts',(-10.8300671649845,-38.2742355626624,
-2.18672421827063));
#61416=CARTESIAN_POINT('Ctrl Pts',(-10.8447154334301,-38.2742355369699,
-2.07406220155496));
#61417=CARTESIAN_POINT('Ctrl Pts',(-10.860404624582,-38.2742355094516,-1.95339429310082));
#61418=CARTESIAN_POINT('Ctrl Pts',(-10.8728498863203,-38.2742354748395,
-1.83229930406024));
#61419=CARTESIAN_POINT('Ctrl Pts',(-10.8822918719481,-38.2742354444275,
-1.71097854711714));
#61420=CARTESIAN_POINT('Ctrl Pts',(-10.8925246339109,-38.2742354114683,
-1.57949704779296));
#61421=CARTESIAN_POINT('Ctrl Pts',(-10.8992312908214,-38.2742353844433,
-1.4477514764851));
#61422=CARTESIAN_POINT('Ctrl Pts',(-10.902772559254,-38.2742353812247,-1.31599141604773));
#61423=CARTESIAN_POINT('Ctrl Pts',(-10.9065651862778,-38.2742353777777,
-1.1748790504173));
#61424=CARTESIAN_POINT('Ctrl Pts',(-10.9066994914357,-38.2742354430818,
-1.03372140575963));
#61425=CARTESIAN_POINT('Ctrl Pts',(-10.9036908051778,-38.2742354987534,
-0.892752944805049));
#61426=CARTESIAN_POINT('Ctrl Pts',(-10.9010418512978,-38.2742355477687,
-0.76863932192075));
#61427=CARTESIAN_POINT('Ctrl Pts',(-10.8959582328936,-38.274235585137,-0.644672308720675));
#61428=CARTESIAN_POINT('Ctrl Pts',(-10.8887788880352,-38.2742355999926,
-0.520973121180266));
#61429=CARTESIAN_POINT('Ctrl Pts',(-10.8866544720092,-38.2742356043884,
-0.484369706578729));
#61430=CARTESIAN_POINT('Ctrl Pts',(-10.8843463777221,-38.2742356072249,
-0.447789460145407));
#61431=CARTESIAN_POINT('Ctrl Pts',(-10.8818628486602,-38.2742356090502,
-0.411234766122649));
#61432=CARTESIAN_POINT('Ctrl Pts',(-10.874153398296,-38.2742356147162,-0.297760515520062));
#61433=CARTESIAN_POINT('Ctrl Pts',(-10.8647666322912,-38.2742356127942,
-0.184597665520344));
#61434=CARTESIAN_POINT('Ctrl Pts',(-10.8539025069105,-38.2742356127992,
-0.0718960390738849));
#61435=CARTESIAN_POINT('Ctrl Pts',(-10.8503866394393,-38.2742356128008,
-0.0354233393866784));
#61436=CARTESIAN_POINT('Ctrl Pts',(-10.8467158042603,-38.2742356128,0.00100136055282495));
#61437=CARTESIAN_POINT('Ctrl Pts',(-10.8428959742023,-38.2742356128,0.0373739107865892));
#61438=CARTESIAN_POINT('Ctrl Pts',(-10.8325161134709,-38.2742356128,0.136211293637533));
#61439=CARTESIAN_POINT('Ctrl Pts',(-10.8210390244351,-38.2742356127994,
0.23467135316527));
#61440=CARTESIAN_POINT('Ctrl Pts',(-10.8085583220161,-38.2742356127967,
0.332816547392836));
#61441=CARTESIAN_POINT('Ctrl Pts',(-10.8022537424958,-38.2742356127953,
0.38239422024847));
#61442=CARTESIAN_POINT('Ctrl Pts',(-10.7956924176571,-38.2742356127937,
0.431891974651008));
#61443=CARTESIAN_POINT('Ctrl Pts',(-10.7888821093176,-38.2742356127936,
0.481320658221345));
#61444=CARTESIAN_POINT('Ctrl Pts',(-10.776316920979,-38.2742356127932,0.572517809279948));
#61445=CARTESIAN_POINT('Ctrl Pts',(-10.7629084439009,-38.2742356128,0.663453825543477));
#61446=CARTESIAN_POINT('Ctrl Pts',(-10.7486857339,-38.2742356128,0.754197251045));
#61447=CARTESIAN_POINT('',(1.34539004473266,-38.2742356128,-9.83573437512944));
#61448=CARTESIAN_POINT('Origin',(-0.000586909216232778,-38.2742356128,-2.71382866332907));
#61449=CARTESIAN_POINT('Ctrl Pts',(10.7486858853,-38.2742356128,0.754196294519999));
#61450=CARTESIAN_POINT('Ctrl Pts',(10.7487507681651,-38.2742356128,0.75378232052338));
#61451=CARTESIAN_POINT('Ctrl Pts',(10.7488160123459,-38.2742356128,0.753365938766182));
#61452=CARTESIAN_POINT('Ctrl Pts',(10.7488811261052,-38.2742356128,0.752950275000361));
#61453=CARTESIAN_POINT('Ctrl Pts',(10.7635805210417,-38.2742356128,0.659114411071533));
#61454=CARTESIAN_POINT('Ctrl Pts',(10.7774074937196,-38.2742356128009,0.565058978147053));
#61455=CARTESIAN_POINT('Ctrl Pts',(10.7903335869119,-38.2742356127991,0.47072184452806));
#61456=CARTESIAN_POINT('Ctrl Pts',(10.8036736449597,-38.2742356127974,0.373363515154428));
#61457=CARTESIAN_POINT('Ctrl Pts',(10.816053894268,-38.2742356128009,0.275705290202299));
#61458=CARTESIAN_POINT('Ctrl Pts',(10.8273976278922,-38.2742356127401,0.177714287921341));
#61459=CARTESIAN_POINT('Ctrl Pts',(10.839417545248,-38.2742356126756,0.0738821821922056));
#61460=CARTESIAN_POINT('Ctrl Pts',(10.8502734645611,-38.2742356125617,-0.0303235245117267));
#61461=CARTESIAN_POINT('Ctrl Pts',(10.8598278196961,-38.2742356120064,-0.134903919694318));
#61462=CARTESIAN_POINT('Ctrl Pts',(10.865531383808,-38.274235611675,-0.197334191580115));
#61463=CARTESIAN_POINT('Ctrl Pts',(10.8707702592039,-38.2742356111793,-0.2598972685949));
#61464=CARTESIAN_POINT('Ctrl Pts',(10.8755086549781,-38.2742356103235,-0.322587644605349));
#61465=CARTESIAN_POINT('Ctrl Pts',(10.8846876179272,-38.2742356086658,-0.444028036264462));
#61466=CARTESIAN_POINT('Ctrl Pts',(10.8920102665268,-38.2742356018392,-0.565865217904973));
#61467=CARTESIAN_POINT('Ctrl Pts',(10.8971588132929,-38.2742355766501,-0.687882711279094));
#61468=CARTESIAN_POINT('Ctrl Pts',(10.8984152249802,-38.2742355705032,-0.717658920314688));
#61469=CARTESIAN_POINT('Ctrl Pts',(10.8995420735683,-38.2742355633587,-0.74744563510997));
#61470=CARTESIAN_POINT('Ctrl Pts',(10.9005346180392,-38.2742355553307,-0.777239287853531));
#61471=CARTESIAN_POINT('Ctrl Pts',(10.9050918295056,-38.2742355184706,-0.914035149284712));
#61472=CARTESIAN_POINT('Ctrl Pts',(10.9068104832314,-38.2742354680899,-1.05102520549406));
#61473=CARTESIAN_POINT('Ctrl Pts',(10.9052251807396,-38.2742354568179,-1.18807097906776));
#61474=CARTESIAN_POINT('Ctrl Pts',(10.9050503429394,-38.2742354555748,-1.20318530690122));
#61475=CARTESIAN_POINT('Ctrl Pts',(10.9048352995357,-38.2742354548037,-1.21830026518269));
#61476=CARTESIAN_POINT('Ctrl Pts',(10.9045794158392,-38.2742354545548,-1.23341563491137));
#61477=CARTESIAN_POINT('Ctrl Pts',(10.902164660392,-38.2742354522063,-1.37605825686335));
#61478=CARTESIAN_POINT('Ctrl Pts',(10.8961336835133,-38.2742354717451,-1.51874802165549));
#61479=CARTESIAN_POINT('Ctrl Pts',(10.8860165731785,-38.2742354967745,-1.66116169724552));
#61480=CARTESIAN_POINT('Ctrl Pts',(10.8777741390387,-38.274235517166,-1.77718646151313));
#61481=CARTESIAN_POINT('Ctrl Pts',(10.8668192226381,-38.2742355405236,-1.89302685111375));
#61482=CARTESIAN_POINT('Ctrl Pts',(10.8529343365985,-38.2742355593193,-2.00850492848472));
#61483=CARTESIAN_POINT('Ctrl Pts',(10.8399197629638,-38.2742355769368,-2.11674477552758));
#61484=CARTESIAN_POINT('Ctrl Pts',(10.8243304799624,-38.2742355905135,-2.22466580464906));
#61485=CARTESIAN_POINT('Ctrl Pts',(10.8060293952058,-38.274235598896,-2.33212834528309));
#61486=CARTESIAN_POINT('Ctrl Pts',(10.7889938389441,-38.2742356066989,-2.43215980141552));
#61487=CARTESIAN_POINT('Ctrl Pts',(10.7696083786317,-38.2742356101862,-2.53179372082084));
#61488=CARTESIAN_POINT('Ctrl Pts',(10.7478046429435,-38.2742356116343,-2.63092871096361));
#61489=CARTESIAN_POINT('Ctrl Pts',(10.7260009072553,-38.2742356130824,-2.73006370110638));
#61490=CARTESIAN_POINT('Ctrl Pts',(10.701778271492,-38.2742356128,-2.82869940493948));
#61491=CARTESIAN_POINT('Ctrl Pts',(10.6751186719673,-38.2742356128,-2.92675080812293));
#61492=CARTESIAN_POINT('Ctrl Pts',(10.649771284584,-38.2742356128,-3.01997602321491));
#61493=CARTESIAN_POINT('Ctrl Pts',(10.6222091430034,-38.2742356128002,-3.11268297971948));
#61494=CARTESIAN_POINT('Ctrl Pts',(10.5924125813341,-38.2742356127998,-3.20473440645213));
#61495=CARTESIAN_POINT('Ctrl Pts',(10.5615425589387,-38.2742356127993,-3.30010210814564));
#61496=CARTESIAN_POINT('Ctrl Pts',(10.5282742733662,-38.2742356128003,-3.394766254745));
#61497=CARTESIAN_POINT('Ctrl Pts',(10.492632290442,-38.2742356127837,-3.48860580498373));
#61498=CARTESIAN_POINT('Ctrl Pts',(10.4561089049894,-38.2742356127667,-3.58476594487729));
#61499=CARTESIAN_POINT('Ctrl Pts',(10.4170931618951,-38.2742356127363,-3.68006035850158));
#61500=CARTESIAN_POINT('Ctrl Pts',(10.3756573972349,-38.2742356125976,-3.77438966006884));
#61501=CARTESIAN_POINT('Ctrl Pts',(10.3325447200932,-38.2742356124533,-3.87253648460131));
#61502=CARTESIAN_POINT('Ctrl Pts',(10.2868123323073,-38.2742356122017,-3.96963864096929));
#61503=CARTESIAN_POINT('Ctrl Pts',(10.2385883089484,-38.2742356115385,-4.06561497714332));
#61504=CARTESIAN_POINT('Ctrl Pts',(10.2340891761824,-38.2742356114766,-4.07456923373088));
#61505=CARTESIAN_POINT('Ctrl Pts',(10.229568386755,-38.2742356114109,-4.08351371121035));
#61506=CARTESIAN_POINT('Ctrl Pts',(10.225026063464,-38.2742356113411,-4.09244835589245));
#61507=CARTESIAN_POINT('Ctrl Pts',(10.1732446638246,-38.2742356105449,-4.19430116937208));
#61508=CARTESIAN_POINT('Ctrl Pts',(10.1186492306826,-38.2742356100661,-4.29488069311728));
#61509=CARTESIAN_POINT('Ctrl Pts',(10.0614431398963,-38.2742356101221,-4.39413041658256));
#61510=CARTESIAN_POINT('Ctrl Pts',(9.99888850242757,-38.2742356101833,-4.50265960263433));
#61511=CARTESIAN_POINT('Ctrl Pts',(9.93321232209925,-38.2742356107809,-4.60959891059151));
#61512=CARTESIAN_POINT('Ctrl Pts',(9.86473431993858,-38.2742356113417,-4.71490795461342));
#61513=CARTESIAN_POINT('Ctrl Pts',(9.79013485868931,-38.2742356119526,-4.82963089776058));
#61514=CARTESIAN_POINT('Ctrl Pts',(9.71221083835581,-38.2742356124542,-4.94241971263403));
#61515=CARTESIAN_POINT('Ctrl Pts',(9.63143135527856,-38.2742356126467,-5.05325356687146));
#61516=CARTESIAN_POINT('Ctrl Pts',(9.5572130696955,-38.2742356128236,-5.15508510048252));
#61517=CARTESIAN_POINT('Ctrl Pts',(9.48058587434832,-38.2742356128,-5.25526742056234));
#61518=CARTESIAN_POINT('Ctrl Pts',(9.40194072919181,-38.2742356128,-5.35379594985318));
#61519=CARTESIAN_POINT('Ctrl Pts',(9.32883368845949,-38.2742356128,-5.44538620872836));
#61520=CARTESIAN_POINT('Ctrl Pts',(9.25398927525911,-38.2742356128027,-5.53553487524453));
#61521=CARTESIAN_POINT('Ctrl Pts',(9.17757104467065,-38.2742356127973,-5.62435381279997));
#61522=CARTESIAN_POINT('Ctrl Pts',(9.0897197837434,-38.274235612791,-5.72646106650603));
#61523=CARTESIAN_POINT('Ctrl Pts',(8.99979124685434,-38.2742356128188,-5.82681131345604));
#61524=CARTESIAN_POINT('Ctrl Pts',(8.90806463915596,-38.2742356125302,-5.92551716111057));
#61525=CARTESIAN_POINT('Ctrl Pts',(8.82230671692448,-38.2742356122604,-6.0178001814833));
#61526=CARTESIAN_POINT('Ctrl Pts',(8.7349530547604,-38.2742356124164,-6.10865432231495));
#61527=CARTESIAN_POINT('Ctrl Pts',(8.64624659176705,-38.2742356125934,-6.19810755671757));
#61528=CARTESIAN_POINT('Ctrl Pts',(8.56780722406295,-38.27423561275,-6.27720726274637));
#61529=CARTESIAN_POINT('Ctrl Pts',(8.48831121256558,-38.2742356127989,-6.355210827178));
#61530=CARTESIAN_POINT('Ctrl Pts',(8.40788750264759,-38.2742356127999,-6.43212465908309));
#61531=CARTESIAN_POINT('Ctrl Pts',(8.39736067259514,-38.2742356128,-6.44219207375438));
#61532=CARTESIAN_POINT('Ctrl Pts',(8.38681787544318,-38.2742356128,-6.45224080652579));
#61533=CARTESIAN_POINT('Ctrl Pts',(8.37625932979455,-38.2742356128,-6.46227086223487));
#61534=CARTESIAN_POINT('Ctrl Pts',(8.29902949041214,-38.2742356128,-6.5356350941269));
#61535=CARTESIAN_POINT('Ctrl Pts',(8.22093580705538,-38.2742356128,-6.60801769618829));
#61536=CARTESIAN_POINT('Ctrl Pts',(8.14213077435888,-38.2742356128,-6.67939428797839));
#61537=CARTESIAN_POINT('Ctrl Pts',(8.06062371227756,-38.2742356128,-6.75321820631358));
#61538=CARTESIAN_POINT('Ctrl Pts',(7.97835543517539,-38.2742356128,-6.8259660231991));
#61539=CARTESIAN_POINT('Ctrl Pts',(7.89543908612086,-38.2742356128,-6.89761648202541));
#61540=CARTESIAN_POINT('Ctrl Pts',(7.80430769103316,-38.2742356128,-6.97636580403453));
#61541=CARTESIAN_POINT('Ctrl Pts',(7.71239362383212,-38.2742356128,-7.05378962970782));
#61542=CARTESIAN_POINT('Ctrl Pts',(7.61978080920412,-38.2742356128,-7.12986536475923));
#61543=CARTESIAN_POINT('Ctrl Pts',(7.53858314384994,-38.2742356128,-7.19656425627969));
#61544=CARTESIAN_POINT('Ctrl Pts',(7.45683925660418,-38.2742356128,-7.26223284344318));
#61545=CARTESIAN_POINT('Ctrl Pts',(7.37461477413073,-38.2742356128,-7.32682367825847));
#61546=CARTESIAN_POINT('Ctrl Pts',(7.26936526560721,-38.2742356128,-7.40950165220167));
#61547=CARTESIAN_POINT('Ctrl Pts',(7.16332488578667,-38.2742356128,-7.49041743571964));
#61548=CARTESIAN_POINT('Ctrl Pts',(7.05653747020417,-38.2742356128,-7.5695101875824));
#61549=CARTESIAN_POINT('Ctrl Pts',(6.93682525271323,-38.2742356128,-7.65817577295409));
#61550=CARTESIAN_POINT('Ctrl Pts',(6.8161179135486,-38.274235612803,-7.7445940920218));
#61551=CARTESIAN_POINT('Ctrl Pts',(6.69424703684613,-38.274235612797,-7.82878929709039));
#61552=CARTESIAN_POINT('Ctrl Pts',(6.66149200838404,-38.2742356127954,-7.85141829930169));
#61553=CARTESIAN_POINT('Ctrl Pts',(6.62865265483242,-38.2742356127928,-7.87388658008447));
#61554=CARTESIAN_POINT('Ctrl Pts',(6.59572521641468,-38.2742356127876,-7.89619429227605));
#61555=CARTESIAN_POINT('Ctrl Pts',(6.45082872454463,-38.2742356127644,-7.99435890493734));
#61556=CARTESIAN_POINT('Ctrl Pts',(6.30423053627507,-38.2742356127633,-8.08940636380272));
#61557=CARTESIAN_POINT('Ctrl Pts',(6.15579746382474,-38.2742356127777,-8.18120196847487));
#61558=CARTESIAN_POINT('Ctrl Pts',(6.04282160604217,-38.2742356127887,-8.25106973451452));
#61559=CARTESIAN_POINT('Ctrl Pts',(5.92878159477683,-38.2742356127977,-8.31905327369613));
#61560=CARTESIAN_POINT('Ctrl Pts',(5.81364866406122,-38.2742356127993,-8.38507547572244));
#61561=CARTESIAN_POINT('Ctrl Pts',(5.75685723795896,-38.2742356128001,-8.41764213570564));
#61562=CARTESIAN_POINT('Ctrl Pts',(5.69980049290472,-38.2742356128,-8.44973130130719));
#61563=CARTESIAN_POINT('Ctrl Pts',(5.64247954756403,-38.2742356128,-8.48133191784778));
#61564=CARTESIAN_POINT('Ctrl Pts',(5.47394056080791,-38.2742356128,-8.57424622449373));
#61565=CARTESIAN_POINT('Ctrl Pts',(5.30310577360258,-38.2742356127314,-8.66295141982281));
#61566=CARTESIAN_POINT('Ctrl Pts',(5.13008046296484,-38.2742356120248,-8.74723786088109));
#61567=CARTESIAN_POINT('Ctrl Pts',(4.96821764570703,-38.2742356113638,-8.82608667644479));
#61568=CARTESIAN_POINT('Ctrl Pts',(4.80443919432874,-38.2742356104042,-8.90106705839819));
#61569=CARTESIAN_POINT('Ctrl Pts',(4.63886472540473,-38.2742356109888,-8.9720316944694));
#61570=CARTESIAN_POINT('Ctrl Pts',(4.48111130549067,-38.2742356115458,-9.0396442563936));
#61571=CARTESIAN_POINT('Ctrl Pts',(4.32172857521236,-38.2742356121698,-9.10362042101943));
#61572=CARTESIAN_POINT('Ctrl Pts',(4.16084936519698,-38.2742356124732,-9.16388103868563));
#61573=CARTESIAN_POINT('Ctrl Pts',(4.01162006782644,-38.2742356127547,-9.21977794191249));
#61574=CARTESIAN_POINT('Ctrl Pts',(3.86110376548713,-38.2742356127939,-9.27247759567066));
#61575=CARTESIAN_POINT('Ctrl Pts',(3.70940907605795,-38.274235612799,-9.32196250357574));
#61576=CARTESIAN_POINT('Ctrl Pts',(3.66957825401608,-38.2742356128003,-9.33495586918361));
#61577=CARTESIAN_POINT('Ctrl Pts',(3.62966617913399,-38.2742356128,-9.34772787071446));
#61578=CARTESIAN_POINT('Ctrl Pts',(3.5896747782925,-38.2742356128,-9.3602788074025));
#61579=CARTESIAN_POINT('Ctrl Pts',(3.52881041758992,-38.2742356128,-9.37938053231491));
#61580=CARTESIAN_POINT('Ctrl Pts',(3.46776633660297,-38.2742356128,-9.39796892242277));
#61581=CARTESIAN_POINT('Ctrl Pts',(3.4065727323248,-38.2742356128,-9.41604021540843));
#61582=CARTESIAN_POINT('Ctrl Pts',(3.32968048064773,-38.2742356128,-9.43874752975565));
#61583=CARTESIAN_POINT('Ctrl Pts',(3.25255020799119,-38.2742356128,-9.4606387062831));
#61584=CARTESIAN_POINT('Ctrl Pts',(3.17515279442903,-38.2742356128,-9.48172455098315));
#61585=CARTESIAN_POINT('Ctrl Pts',(3.10379770456818,-38.2742356128,-9.50116424895388));
#61586=CARTESIAN_POINT('Ctrl Pts',(3.0322103272402,-38.2742356128,-9.51992044345575));
#61587=CARTESIAN_POINT('Ctrl Pts',(2.96036414388182,-38.2742356128,-9.53800370488677));
#61588=CARTESIAN_POINT('Ctrl Pts',(2.89997433382167,-38.2742356128,-9.55320346459621));
#61589=CARTESIAN_POINT('Ctrl Pts',(2.83940025379948,-38.2742356128,-9.56792807659975));
#61590=CARTESIAN_POINT('Ctrl Pts',(2.77866084909843,-38.2742356128,-9.5821780964647));
#61591=CARTESIAN_POINT('Ctrl Pts',(2.7249273018283,-38.2742356128,-9.59478447810084));
#61592=CARTESIAN_POINT('Ctrl Pts',(2.67106397863643,-38.2742356128,-9.60701951748907));
#61593=CARTESIAN_POINT('Ctrl Pts',(2.61712385866369,-38.2742356128,-9.6188766151844));
#61594=CARTESIAN_POINT('Ctrl Pts',(2.5791100250399,-38.2742356128,-9.62723280236529));
#61595=CARTESIAN_POINT('Ctrl Pts',(2.54105881814865,-38.2742356128,-9.63540114632831));
#61596=CARTESIAN_POINT('Ctrl Pts',(2.50300436723069,-38.2742356128,-9.64337655749628));
#61597=CARTESIAN_POINT('Ctrl Pts',(2.47884007178717,-38.2742356128,-9.64844088471945));
#61598=CARTESIAN_POINT('Ctrl Pts',(2.45468813957632,-38.2742356128003,-9.65342485999044));
#61599=CARTESIAN_POINT('Ctrl Pts',(2.4304966052416,-38.2742356127983,-9.65833864391884));
#61600=CARTESIAN_POINT('Ctrl Pts',(2.40173189730255,-38.2742356127959,-9.66418133077037));
#61601=CARTESIAN_POINT('Ctrl Pts',(2.37291265402142,-38.2742356127891,-9.66992453918787));
#61602=CARTESIAN_POINT('Ctrl Pts',(2.34403422863427,-38.2742356127787,-9.67556977277591));
#61603=CARTESIAN_POINT('Ctrl Pts',(2.31516852578334,-38.2742356127683,-9.68121251932776));
#61604=CARTESIAN_POINT('Ctrl Pts',(2.28624826799992,-38.274235612755,-9.68675655791408));
#61605=CARTESIAN_POINT('Ctrl Pts',(2.25729271764595,-38.2742356127499,-9.69219828457188));
#61606=CARTESIAN_POINT('Ctrl Pts',(2.23247417729856,-38.2742356127456,-9.69686252721156));
#61607=CARTESIAN_POINT('Ctrl Pts',(2.20763015646299,-38.2742356127488,-9.70145144234736));
#61608=CARTESIAN_POINT('Ctrl Pts',(2.18277308169882,-38.2742356127574,-9.70596255728258));
#61609=CARTESIAN_POINT('Ctrl Pts',(2.16642284667288,-38.2742356127631,-9.70892983280151));
#61610=CARTESIAN_POINT('Ctrl Pts',(2.15006640220555,-38.2742356127709,-9.71186355167236));
#61611=CARTESIAN_POINT('Ctrl Pts',(2.133694660445,-38.2742356127786,-9.714765315785));
#61612=CARTESIAN_POINT('Ctrl Pts',(2.11282185420172,-38.2742356127884,-9.71846485862978));
#61613=CARTESIAN_POINT('Ctrl Pts',(2.09193075869325,-38.2742356127951,-9.7221114546842));
#61614=CARTESIAN_POINT('Ctrl Pts',(2.07096182677399,-38.2742356127978,-9.72571609201187));
#61615=CARTESIAN_POINT('Ctrl Pts',(2.05047922380141,-38.2742356128004,-9.72923712758617));
#61616=CARTESIAN_POINT('Ctrl Pts',(2.02992295383359,-38.2742356128,-9.73271802045324));
#61617=CARTESIAN_POINT('Ctrl Pts',(2.00919017821102,-38.2742356128,-9.73617746265811));
#61618=CARTESIAN_POINT('Ctrl Pts',(1.99020952480306,-38.2742356128,-9.73934454817869));
#61619=CARTESIAN_POINT('Ctrl Pts',(1.97105595139246,-38.2742356128,-9.74249735848642));
#61620=CARTESIAN_POINT('Ctrl Pts',(1.95166188100995,-38.2742356128,-9.74564856373225));
#61621=CARTESIAN_POINT('Ctrl Pts',(1.93060030650991,-38.2742356128,-9.74907070992131));
#61622=CARTESIAN_POINT('Ctrl Pts',(1.90925526880756,-38.2742356128,-9.75249094179596));
#61623=CARTESIAN_POINT('Ctrl Pts',(1.88760220884021,-38.2742356128,-9.75591654570863));
#61624=CARTESIAN_POINT('Ctrl Pts',(1.86420953953537,-38.2742356128,-9.75961736303512));
#61625=CARTESIAN_POINT('Ctrl Pts',(1.84045811266083,-38.2742356128,-9.76332434748164));
#61626=CARTESIAN_POINT('Ctrl Pts',(1.81637926323375,-38.2742356128,-9.76703763917552));
#61627=CARTESIAN_POINT('Ctrl Pts',(1.79251866984357,-38.2742356128,-9.77071727276912));
#61628=CARTESIAN_POINT('Ctrl Pts',(1.76833830132548,-38.2742356128,-9.77440285307543));
#61629=CARTESIAN_POINT('Ctrl Pts',(1.74390696076956,-38.2742356128,-9.77808886554085));
#61630=CARTESIAN_POINT('Ctrl Pts',(1.7075926768814,-38.2742356128,-9.78356768496044));
#61631=CARTESIAN_POINT('Ctrl Pts',(1.67072328673315,-38.2742356128,-9.78904774830279));
#61632=CARTESIAN_POINT('Ctrl Pts',(1.63351884074209,-38.2742356128,-9.79451085705819));
#61633=CARTESIAN_POINT('Ctrl Pts',(1.60635470047306,-38.2742356128,-9.79849964518776));
#61634=CARTESIAN_POINT('Ctrl Pts',(1.57901385029371,-38.2742356127999,-9.80247908710984));
#61635=CARTESIAN_POINT('Ctrl Pts',(1.5515482103417,-38.2742356127999,-9.80644638056753));
#61636=CARTESIAN_POINT('Ctrl Pts',(1.52760933636065,-38.2742356127999,-9.80990424786265));
#61637=CARTESIAN_POINT('Ctrl Pts',(1.50357615349941,-38.2742356127999,-9.81335280883629));
#61638=CARTESIAN_POINT('Ctrl Pts',(1.47944139357322,-38.2742356127999,-9.81679588996537));
#61639=CARTESIAN_POINT('Ctrl Pts',(1.47214765940106,-38.2742356127999,-9.81783641900173));
#61640=CARTESIAN_POINT('Ctrl Pts',(1.46484430455737,-38.2742356127999,-9.81887649496593));
#61641=CARTESIAN_POINT('Ctrl Pts',(1.45753015363098,-38.2742356127999,-9.81991635837771));
#61642=CARTESIAN_POINT('Ctrl Pts',(1.43544665144904,-38.2742356127999,-9.82305600181057));
#61643=CARTESIAN_POINT('Ctrl Pts',(1.41326877283713,-38.2742356128,-9.8261930691028));
#61644=CARTESIAN_POINT('Ctrl Pts',(1.39094458750546,-38.2742356128,-9.8293370211813));
#61645=CARTESIAN_POINT('Ctrl Pts',(1.38335731497305,-38.2742356128,-9.83040554936694));
#61646=CARTESIAN_POINT('Ctrl Pts',(1.37575271635051,-38.2742356128,-9.83147493276944));
#61647=CARTESIAN_POINT('Ctrl Pts',(1.36812735591189,-38.2742356128,-9.83254573941051));
#61648=CARTESIAN_POINT('Ctrl Pts',(1.36056853098454,-38.2742356128,-9.83360720266801));
#61649=CARTESIAN_POINT('Ctrl Pts',(1.3530001371342,-38.2742356128,-9.83466855937952));
#61650=CARTESIAN_POINT('Ctrl Pts',(1.3453969549,-38.2742356128,-9.83573340734));
#61651=CARTESIAN_POINT('',(10.3535098587966,-38.2742356128,0.692261636805038));
#61652=CARTESIAN_POINT('',(2.11953732489483,-38.2742356128,-9.3109010209371));
#61653=CARTESIAN_POINT('Ctrl Pts',(10.3535104557559,-38.2742356128,0.692257828105415));
#61654=CARTESIAN_POINT('Ctrl Pts',(10.3544069581266,-38.2742356128,0.686538032597277));
#61655=CARTESIAN_POINT('Ctrl Pts',(10.3552979558028,-38.2742356128,0.680830538803156));
#61656=CARTESIAN_POINT('Ctrl Pts',(10.3561866610052,-38.2742356128,0.675114926919618));
#61657=CARTESIAN_POINT('Ctrl Pts',(10.366268957202,-38.2742356128,0.610271723800219));
#61658=CARTESIAN_POINT('Ctrl Pts',(10.3759130539615,-38.2742356128,0.54530562811968));
#61659=CARTESIAN_POINT('Ctrl Pts',(10.3851207453064,-38.2742356128,0.480185305521681));
#61660=CARTESIAN_POINT('Ctrl Pts',(10.3977033092524,-38.2742356128,0.391196590262687));
#61661=CARTESIAN_POINT('Ctrl Pts',(10.4094717744052,-38.2742356128,0.301923984939355));
#61662=CARTESIAN_POINT('Ctrl Pts',(10.4203818846726,-38.2742356128,0.212330742444658));
#61663=CARTESIAN_POINT('Ctrl Pts',(10.4318076654474,-38.2742356128,0.118502841300599));
#61664=CARTESIAN_POINT('Ctrl Pts',(10.4422917188659,-38.2742356128,0.0243231242626569));
#61665=CARTESIAN_POINT('Ctrl Pts',(10.4517319391243,-38.2742356128,-0.0702256999872293));
#61666=CARTESIAN_POINT('Ctrl Pts',(10.4539569878336,-38.2742356128,-0.0925107456319238));
#61667=CARTESIAN_POINT('Ctrl Pts',(10.4561238455536,-38.2742356128,-0.114816186554481));
#61668=CARTESIAN_POINT('Ctrl Pts',(10.4582308198332,-38.2742356128,-0.137142046414437));
#61669=CARTESIAN_POINT('Ctrl Pts',(10.46787464667,-38.2742356128,-0.239329685132882));
#61670=CARTESIAN_POINT('Ctrl Pts',(10.4762642537817,-38.2742356128652,-0.34193688806554));
#61671=CARTESIAN_POINT('Ctrl Pts',(10.4832063794709,-38.2742356126705,-0.444942932774762));
#61672=CARTESIAN_POINT('Ctrl Pts',(10.4907263606177,-38.2742356124595,-0.556523095523347));
#61673=CARTESIAN_POINT('Ctrl Pts',(10.4965469735829,-38.2742356121524,-0.668571745847588));
#61674=CARTESIAN_POINT('Ctrl Pts',(10.5003763583156,-38.2742356088356,-0.781018782404027));
#61675=CARTESIAN_POINT('Ctrl Pts',(10.5031108430682,-38.2742356064671,-0.861314894808877));
#61676=CARTESIAN_POINT('Ctrl Pts',(10.5048289106488,-38.2742356025357,-0.941813195868945));
#61677=CARTESIAN_POINT('Ctrl Pts',(10.5054162157459,-38.2742355941479,-1.02247432568956));
#61678=CARTESIAN_POINT('Ctrl Pts',(10.506280668347,-38.2742355818018,-1.14119919937776));
#61679=CARTESIAN_POINT('Ctrl Pts',(10.5047222260127,-38.2742355702844,-1.26035174466673));
#61680=CARTESIAN_POINT('Ctrl Pts',(10.5003661398209,-38.2742355689454,-1.37976394248105));
#61681=CARTESIAN_POINT('Ctrl Pts',(10.4962520805443,-38.2742355676808,-1.49254152274945));
#61682=CARTESIAN_POINT('Ctrl Pts',(10.4896410471889,-38.2742355754336,-1.60555021006541));
#61683=CARTESIAN_POINT('Ctrl Pts',(10.480234955494,-38.274235586815,-1.71860685456706));
#61684=CARTESIAN_POINT('Ctrl Pts',(10.4768077977861,-38.2742355909618,-1.75979962231792));
#61685=CARTESIAN_POINT('Ctrl Pts',(10.4730098701887,-38.2742355954618,-1.80099837490319));
#61686=CARTESIAN_POINT('Ctrl Pts',(10.4688279746376,-38.2742355996032,-1.84219295234867));
#61687=CARTESIAN_POINT('Ctrl Pts',(10.4585921454847,-38.2742356097399,-1.94302298303868));
#61688=CARTESIAN_POINT('Ctrl Pts',(10.4460369350901,-38.2742356122915,-2.04384845382126));
#61689=CARTESIAN_POINT('Ctrl Pts',(10.4309775984689,-38.2742356126884,-2.14448461737793));
#61690=CARTESIAN_POINT('Ctrl Pts',(10.425575455875,-38.2742356128308,-2.18058520529327));
#61691=CARTESIAN_POINT('Ctrl Pts',(10.4198514676322,-38.2742356128,-2.21666117475377));
#61692=CARTESIAN_POINT('Ctrl Pts',(10.4137985541642,-38.2742356128,-2.25270313970304));
#61693=CARTESIAN_POINT('Ctrl Pts',(10.3981876175369,-38.2742356128,-2.34565818254684));
#61694=CARTESIAN_POINT('Ctrl Pts',(10.3804038373573,-38.2742356128,-2.4383974632595));
#61695=CARTESIAN_POINT('Ctrl Pts',(10.360369967161,-38.2742356128,-2.53073330308211));
#61696=CARTESIAN_POINT('Ctrl Pts',(10.3509818947903,-38.2742356128,-2.57400280309234));
#61697=CARTESIAN_POINT('Ctrl Pts',(10.3411003824232,-38.2742356128,-2.61718347718347));
#61698=CARTESIAN_POINT('Ctrl Pts',(10.3307213130425,-38.2742356128,-2.66025483526559));
#61699=CARTESIAN_POINT('Ctrl Pts',(10.3088850088353,-38.2742356128,-2.75087175314097));
#61700=CARTESIAN_POINT('Ctrl Pts',(10.2848413058874,-38.2742356128,-2.84101405148704));
#61701=CARTESIAN_POINT('Ctrl Pts',(10.2585770843906,-38.2742356128,-2.93052069295465));
#61702=CARTESIAN_POINT('Ctrl Pts',(10.2332623103076,-38.2742356128,-3.01679168362346));
#61703=CARTESIAN_POINT('Ctrl Pts',(10.2058844678468,-38.2742356128,-3.1024720520646));
#61704=CARTESIAN_POINT('Ctrl Pts',(10.17647883038,-38.2742356128,-3.18740411871625));
#61705=CARTESIAN_POINT('Ctrl Pts',(10.1701327838924,-38.2742356128,-3.2057333538454));
#61706=CARTESIAN_POINT('Ctrl Pts',(10.1636924803055,-38.2742356128,-3.22402768868211));
#61707=CARTESIAN_POINT('Ctrl Pts',(10.1571585890214,-38.2742356128,-3.24228545796317));
#61708=CARTESIAN_POINT('Ctrl Pts',(10.1253246654115,-38.2742356128,-3.33123956009105));
#61709=CARTESIAN_POINT('Ctrl Pts',(10.0912547039976,-38.2742356128,-3.41935554389994));
#61710=CARTESIAN_POINT('Ctrl Pts',(10.055047525097,-38.2742356128,-3.506496931939));
#61711=CARTESIAN_POINT('Ctrl Pts',(10.0175120766863,-38.2742356128,-3.5968351238248));
#61712=CARTESIAN_POINT('Ctrl Pts',(9.9776798930849,-38.2742356128,-3.6861260009171));
#61713=CARTESIAN_POINT('Ctrl Pts',(9.93569575213086,-38.2742356128,-3.77426091291076));
#61714=CARTESIAN_POINT('Ctrl Pts',(9.93138836113134,-38.2742356128,-3.78330317310804));
#61715=CARTESIAN_POINT('Ctrl Pts',(9.92705834651865,-38.2742356128,-3.79233330120649));
#61716=CARTESIAN_POINT('Ctrl Pts',(9.92270588308604,-38.2742356128,-3.80135120370286));
#61717=CARTESIAN_POINT('Ctrl Pts',(9.87657224942915,-38.2742356128,-3.8969358344672));
#61718=CARTESIAN_POINT('Ctrl Pts',(9.82789890031301,-38.2742356128,-3.99117465821485));
#61719=CARTESIAN_POINT('Ctrl Pts',(9.77688915570328,-38.2742356128,-4.08401465291981));
#61720=CARTESIAN_POINT('Ctrl Pts',(9.72389056639723,-38.2742356128,-4.18047443306944));
#61721=CARTESIAN_POINT('Ctrl Pts',(9.66837026041182,-38.2742356128,-4.27542463113601));
#61722=CARTESIAN_POINT('Ctrl Pts',(9.61058522072467,-38.2742356128,-4.36885021802721));
#61723=CARTESIAN_POINT('Ctrl Pts',(9.57944428658444,-38.2742356128,-4.41919819847582));
#61724=CARTESIAN_POINT('Ctrl Pts',(9.54764507174215,-38.2742356128,-4.46910587319495));
#61725=CARTESIAN_POINT('Ctrl Pts',(9.51522480958567,-38.2742356128,-4.51858291647522));
#61726=CARTESIAN_POINT('Ctrl Pts',(9.44022898792422,-38.2742356128,-4.63303515305101));
#61727=CARTESIAN_POINT('Ctrl Pts',(9.36191723932152,-38.2742356128,-4.74516444844837));
#61728=CARTESIAN_POINT('Ctrl Pts',(9.28085520537354,-38.2742356128,-4.85501095685734));
#61729=CARTESIAN_POINT('Ctrl Pts',(9.25126730820571,-38.2742356128,-4.89510527767262));
#61730=CARTESIAN_POINT('Ctrl Pts',(9.221313265791,-38.2742356128,-4.93489597715081));
#61731=CARTESIAN_POINT('Ctrl Pts',(9.19102120554409,-38.2742356128,-4.97438641804631));
#61732=CARTESIAN_POINT('Ctrl Pts',(9.11515162680019,-38.2742356128,-5.07329428666702));
#61733=CARTESIAN_POINT('Ctrl Pts',(9.03715669685487,-38.2742356128,-5.17033255715841));
#61734=CARTESIAN_POINT('Ctrl Pts',(8.95733536342387,-38.2742356128,-5.26565777720866));
#61735=CARTESIAN_POINT('Ctrl Pts',(8.87614395347642,-38.2742356128,-5.36261918698168));
#61736=CARTESIAN_POINT('Ctrl Pts',(8.79306294442929,-38.2742356128,-5.45780803995178));
#61737=CARTESIAN_POINT('Ctrl Pts',(8.70837234666383,-38.2742356128,-5.55134671849507));
#61738=CARTESIAN_POINT('Ctrl Pts',(8.62213413938125,-38.2742356128,-5.64659469361852));
#61739=CARTESIAN_POINT('Ctrl Pts',(8.53422702575129,-38.2742356128,-5.74013141101811));
#61740=CARTESIAN_POINT('Ctrl Pts',(8.44491040792852,-38.2742356128,-5.83204571560467));
#61741=CARTESIAN_POINT('Ctrl Pts',(8.35291571815627,-38.2742356128,-5.92671598125279));
#61742=CARTESIAN_POINT('Ctrl Pts',(8.25942585235678,-38.2742356128,-6.01966488169897));
#61743=CARTESIAN_POINT('Ctrl Pts',(8.16468476449867,-38.2742356128,-6.11095020924391));
#61744=CARTESIAN_POINT('Ctrl Pts',(8.06824182207186,-38.2742356128,-6.20387531479065));
#61745=CARTESIAN_POINT('Ctrl Pts',(7.97050234489563,-38.2742356128,-6.2950762146568));
#61746=CARTESIAN_POINT('Ctrl Pts',(7.8716822016181,-38.2742356128,-6.38457794878723));
#61747=CARTESIAN_POINT('Ctrl Pts',(7.77009921254859,-38.2742356128,-6.47658200158788));
#61748=CARTESIAN_POINT('Ctrl Pts',(7.66737439888165,-38.2742356128,-6.56679020359953));
#61749=CARTESIAN_POINT('Ctrl Pts',(7.56369750800012,-38.2742356128,-6.65519724548669));
#61750=CARTESIAN_POINT('Ctrl Pts',(7.5159885341293,-38.2742356128,-6.69587949603962));
#61751=CARTESIAN_POINT('Ctrl Pts',(7.46807732954183,-38.2742356128,-6.73617992784729));
#61752=CARTESIAN_POINT('Ctrl Pts',(7.41997923973326,-38.2742356128,-6.77609613343191));
#61753=CARTESIAN_POINT('Ctrl Pts',(7.32791155601165,-38.2742356128,-6.85250234011827));
#61754=CARTESIAN_POINT('Ctrl Pts',(7.23515048086156,-38.2742356127366,-6.92750063651648));
#61755=CARTESIAN_POINT('Ctrl Pts',(7.14164675550522,-38.274235612635,-7.00113625961658));
#61756=CARTESIAN_POINT('Ctrl Pts',(7.08482858540921,-38.2742356125733,-7.04588144321736));
#61757=CARTESIAN_POINT('Ctrl Pts',(7.02773667956031,-38.2742356125682,-7.09012245084894));
#61758=CARTESIAN_POINT('Ctrl Pts',(6.97036425873578,-38.274235612668,-7.13386121169709));
#61759=CARTESIAN_POINT('Ctrl Pts',(6.86943011864084,-38.2742356128435,-7.21080992941861));
#61760=CARTESIAN_POINT('Ctrl Pts',(6.76757099008427,-38.2742356127991,-7.28622960703381));
#61761=CARTESIAN_POINT('Ctrl Pts',(6.66470672473084,-38.2742356127998,-7.36011874372879));
#61762=CARTESIAN_POINT('Ctrl Pts',(6.6128801431363,-38.2742356128002,-7.39734665138666));
#61763=CARTESIAN_POINT('Ctrl Pts',(6.5607987888592,-38.2742356128,-7.43418521583754));
#61764=CARTESIAN_POINT('Ctrl Pts',(6.50845458459114,-38.2742356128,-7.47062987547125));
#61765=CARTESIAN_POINT('Ctrl Pts',(6.38936601296616,-38.2742356128,-7.55354531032837));
#61766=CARTESIAN_POINT('Ctrl Pts',(6.26890066502405,-38.2742356128,-7.63443380526014));
#61767=CARTESIAN_POINT('Ctrl Pts',(6.14705288221731,-38.2742356128,-7.71315424109138));
#61768=CARTESIAN_POINT('Ctrl Pts',(6.01029189266294,-38.2742356128,-7.80150943684827));
#61769=CARTESIAN_POINT('Ctrl Pts',(5.87178900326465,-38.2742356128,-7.88713120988784));
#61770=CARTESIAN_POINT('Ctrl Pts',(5.73158927890684,-38.2742356128,-7.96978234287356));
#61771=CARTESIAN_POINT('Ctrl Pts',(5.66437973320283,-38.2742356128,-8.00940399780431));
#61772=CARTESIAN_POINT('Ctrl Pts',(5.59678215398082,-38.2742356128,-8.04834203293516));
#61773=CARTESIAN_POINT('Ctrl Pts',(5.52880173122316,-38.2742356128,-8.08657247318979));
#61774=CARTESIAN_POINT('Ctrl Pts',(5.39297979815478,-38.2742356128,-8.16295523291388));
#61775=CARTESIAN_POINT('Ctrl Pts',(5.25560722450796,-38.2742356128,-8.23652229137831));
#61776=CARTESIAN_POINT('Ctrl Pts',(5.11673653035794,-38.2742356128,-8.30710645917144));
#61777=CARTESIAN_POINT('Ctrl Pts',(4.99592856393252,-38.2742356128,-8.36850983750918));
#61778=CARTESIAN_POINT('Ctrl Pts',(4.873987551265,-38.2742356128,-8.42765509567402));
#61779=CARTESIAN_POINT('Ctrl Pts',(4.75096134365824,-38.2742356128,-8.48446936967895));
#61780=CARTESIAN_POINT('Ctrl Pts',(4.67791920577842,-38.2742356128,-8.518200686901));
#61781=CARTESIAN_POINT('Ctrl Pts',(4.60449475274289,-38.2742356128,-8.55111111808754));
#61782=CARTESIAN_POINT('Ctrl Pts',(4.53069936808626,-38.2742356128,-8.5831942594361));
#61783=CARTESIAN_POINT('Ctrl Pts',(4.39198916695835,-38.2742356128,-8.6434996431668));
#61784=CARTESIAN_POINT('Ctrl Pts',(4.25195587633228,-38.2742356128,-8.70088498843151));
#61785=CARTESIAN_POINT('Ctrl Pts',(4.11066678383247,-38.2742356128,-8.75528142586651));
#61786=CARTESIAN_POINT('Ctrl Pts',(3.96436874851434,-38.2742356128,-8.81160631113716));
#61787=CARTESIAN_POINT('Ctrl Pts',(3.81672386119578,-38.2742356128,-8.86472713193888));
#61788=CARTESIAN_POINT('Ctrl Pts',(3.6678316200746,-38.2742356128,-8.91461741066908));
#61789=CARTESIAN_POINT('Ctrl Pts',(3.51207949781546,-38.2742356127999,-8.96680627379463));
#61790=CARTESIAN_POINT('Ctrl Pts',(3.3549618224836,-38.2742356127999,-9.01546072920466));
#61791=CARTESIAN_POINT('Ctrl Pts',(3.19662740736046,-38.2742356127999,-9.06059499188016));
#61792=CARTESIAN_POINT('Ctrl Pts',(3.03129330521691,-38.2742356127999,-9.10772456121328));
#61793=CARTESIAN_POINT('Ctrl Pts',(2.8646317213971,-38.2742356127999,-9.15101681634443));
#61794=CARTESIAN_POINT('Ctrl Pts',(2.69686030237699,-38.2742356127999,-9.19052227789939));
#61795=CARTESIAN_POINT('Ctrl Pts',(2.52908888335688,-38.2742356127999,-9.23002773945435));
#61796=CARTESIAN_POINT('Ctrl Pts',(2.36020715659891,-38.2742356128,-9.26574773355228));
#61797=CARTESIAN_POINT('Ctrl Pts',(2.19048902652532,-38.2742356128,-9.2977482196728));
#61798=CARTESIAN_POINT('Ctrl Pts',(2.16685412882389,-38.2742356128,-9.3022045981135));
#61799=CARTESIAN_POINT('Ctrl Pts',(2.14320468147333,-38.2742356128,-9.30658854411333));
#61800=CARTESIAN_POINT('Ctrl Pts',(2.11953749589,-38.2742356128,-9.31090098978));
#61801=CARTESIAN_POINT('',(2.08573866528107,-38.2742356128,-9.31728218620194));
#61802=CARTESIAN_POINT('Ctrl Pts',(2.11953715342988,-38.2742356128,-9.31090105217976));
#61803=CARTESIAN_POINT('Ctrl Pts',(2.11797894915308,-38.2742356128,-9.31118497696086));
#61804=CARTESIAN_POINT('Ctrl Pts',(2.11642436145393,-38.2742356128002,-9.31146961094749));
#61805=CARTESIAN_POINT('Ctrl Pts',(2.11486501656171,-38.2742356127997,-9.31175659977283));
#61806=CARTESIAN_POINT('Ctrl Pts',(2.11438298834213,-38.2742356127995,-9.31184531440755));
#61807=CARTESIAN_POINT('Ctrl Pts',(2.11390088140109,-38.2742356127993,-9.31193417995486));
#61808=CARTESIAN_POINT('Ctrl Pts',(2.11341946076803,-38.2742356127989,-9.31202304609802));
#61809=CARTESIAN_POINT('Ctrl Pts',(2.11153045027428,-38.2742356127973,-9.3123717413251));
#61810=CARTESIAN_POINT('Ctrl Pts',(2.10961613871839,-38.2742356127953,-9.31272773883357));
#61811=CARTESIAN_POINT('Ctrl Pts',(2.1076821531108,-38.2742356127946,-9.31308956372315));
#61812=CARTESIAN_POINT('Ctrl Pts',(2.10497282330549,-38.2742356127937,-9.31359644596353));
#61813=CARTESIAN_POINT('Ctrl Pts',(2.10223212032299,-38.2742356127952,-9.31411334934674));
#61814=CARTESIAN_POINT('Ctrl Pts',(2.09955927298003,-38.2742356127967,-9.31462091916872));
#61815=CARTESIAN_POINT('Ctrl Pts',(2.09775952512019,-38.2742356127978,-9.31496268866904));
#61816=CARTESIAN_POINT('Ctrl Pts',(2.09599276630409,-38.2742356127987,-9.31529981756808));
#61817=CARTESIAN_POINT('Ctrl Pts',(2.09425998150645,-38.2742356127993,-9.31563221100442));
#61818=CARTESIAN_POINT('Ctrl Pts',(2.09279115396838,-38.2742356127997,-9.31591397053591));
#61819=CARTESIAN_POINT('Ctrl Pts',(2.09134719651597,-38.2742356127999,-9.31619224217171));
#61820=CARTESIAN_POINT('Ctrl Pts',(2.08989189609338,-38.2742356128,-9.31647410888022));
#61821=CARTESIAN_POINT('Ctrl Pts',(2.08892721858332,-38.2742356128,-9.31666095035317));
#61822=CARTESIAN_POINT('Ctrl Pts',(2.08795684384456,-38.2742356128,-9.31684950975924));
#61823=CARTESIAN_POINT('Ctrl Pts',(2.08695750245697,-38.2742356128,-9.31704430756847));
#61824=CARTESIAN_POINT('Ctrl Pts',(2.08655395799507,-38.2742356128,-9.31712296895295));
#61825=CARTESIAN_POINT('Ctrl Pts',(2.08614978311668,-38.2742356128,-9.31720185229));
#61826=CARTESIAN_POINT('Ctrl Pts',(2.08573866565001,-38.2742356128,-9.31728218809));
#61827=CARTESIAN_POINT('',(0.417273437277162,-38.2742356128,-7.9503178208061));
#61828=CARTESIAN_POINT('Ctrl Pts',(2.08573866481991,-38.2742356128,-9.31728218384186));
#61829=CARTESIAN_POINT('Ctrl Pts',(2.07763203559797,-38.2742356128,-9.31886622212027));
#61830=CARTESIAN_POINT('Ctrl Pts',(2.06950380369,-38.2742356128,-9.320380182645));
#61831=CARTESIAN_POINT('Ctrl Pts',(2.06136477179,-38.2742356128,-9.321821861545));
#61832=CARTESIAN_POINT('Ctrl Pts',(2.05322573989,-38.2742356128,-9.323263540445));
#61833=CARTESIAN_POINT('Ctrl Pts',(2.04507348953682,-38.2742356128,-9.32463342169253));
#61834=CARTESIAN_POINT('Ctrl Pts',(2.03690970729997,-38.2742356127999,-9.32593117246363));
#61835=CARTESIAN_POINT('Ctrl Pts',(2.02058253631524,-38.2742356127998,-9.32852661145511));
#61836=CARTESIAN_POINT('Ctrl Pts',(2.00420686669781,-38.2742356127997,-9.33083386430894));
#61837=CARTESIAN_POINT('Ctrl Pts',(1.98779626405356,-38.2742356127995,-9.33285066337887));
#61838=CARTESIAN_POINT('Ctrl Pts',(1.93350680188262,-38.2742356127992,-9.3395226265716));
#61839=CARTESIAN_POINT('Ctrl Pts',(1.87881722880592,-38.2742356127996,-9.34301407998262));
#61840=CARTESIAN_POINT('Ctrl Pts',(1.82410851328607,-38.2742356127998,-9.34329112627487));
#61841=CARTESIAN_POINT('Ctrl Pts',(1.77958953966205,-38.2742356128,-9.34351657146144));
#61842=CARTESIAN_POINT('Ctrl Pts',(1.73505802515345,-38.2742356128,-9.34161458422846));
#61843=CARTESIAN_POINT('Ctrl Pts',(1.69071856317199,-38.2742356128,-9.3375922987591));
#61844=CARTESIAN_POINT('Ctrl Pts',(1.63486128345798,-38.2742356128,-9.33252516635579));
#61845=CARTESIAN_POINT('Ctrl Pts',(1.57931009792603,-38.2742356128,-9.32409203444833));
#61846=CARTESIAN_POINT('Ctrl Pts',(1.52446757032607,-38.2742356128,-9.31235583273348));
#61847=CARTESIAN_POINT('Ctrl Pts',(1.46867636729189,-38.2742356128,-9.30041661619155));
#61848=CARTESIAN_POINT('Ctrl Pts',(1.41361897746577,-38.2742356128,-9.28505921699745));
#61849=CARTESIAN_POINT('Ctrl Pts',(1.35970641711599,-38.2742356128,-9.26640242007238));
#61850=CARTESIAN_POINT('Ctrl Pts',(1.30544267878404,-38.2742356128,-9.24762409569146));
#61851=CARTESIAN_POINT('Ctrl Pts',(1.25233916318076,-38.2742356128,-9.22550350962761));
#61852=CARTESIAN_POINT('Ctrl Pts',(1.20079564211786,-38.2742356128,-9.2002113020856));
#61853=CARTESIAN_POINT('Ctrl Pts',(1.14903365499695,-38.2742356128,-9.17481189408918));
#61854=CARTESIAN_POINT('Ctrl Pts',(1.09884535235233,-38.2742356128,-9.14621421029534));
#61855=CARTESIAN_POINT('Ctrl Pts',(1.05060964073121,-38.2742356128,-9.11463668493604));
#61856=CARTESIAN_POINT('Ctrl Pts',(1.01815169737214,-38.2742356128,-9.09338808104725));
#61857=CARTESIAN_POINT('Ctrl Pts',(0.98657734033846,-38.2742356128,-9.0707911498067));
#61858=CARTESIAN_POINT('Ctrl Pts',(0.955993931424741,-38.2742356128,-9.04692298582716));
#61859=CARTESIAN_POINT('Ctrl Pts',(0.909151723851522,-38.2742356128,-9.01036599197877));
#61860=CARTESIAN_POINT('Ctrl Pts',(0.864636917513829,-38.2742356128014,
-8.97082583521411));
#61861=CARTESIAN_POINT('Ctrl Pts',(0.822807595223311,-38.2742356127971,
-8.92862289484912));
#61862=CARTESIAN_POINT('Ctrl Pts',(0.781747848673634,-38.2742356127929,
-8.88719640404915));
#61863=CARTESIAN_POINT('Ctrl Pts',(0.743275948023315,-38.2742356127857,
-8.84320438706447));
#61864=CARTESIAN_POINT('Ctrl Pts',(0.707693495085963,-38.274235612732,-8.79698388515189));
#61865=CARTESIAN_POINT('Ctrl Pts',(0.698124380455637,-38.2742356127175,
-8.78455390226534));
#61866=CARTESIAN_POINT('Ctrl Pts',(0.688764013973583,-38.2742356126994,
-8.77196293551276));
#61867=CARTESIAN_POINT('Ctrl Pts',(0.679617753842452,-38.2742356126758,
-8.75921794590775));
#61868=CARTESIAN_POINT('Ctrl Pts',(0.64666137843158,-38.2742356125909,-8.71329440382516));
#61869=CARTESIAN_POINT('Ctrl Pts',(0.616487257383922,-38.2742356124953,
-8.66537096962203));
#61870=CARTESIAN_POINT('Ctrl Pts',(0.589321147407174,-38.2742356124624,
-8.61579545953694));
#61871=CARTESIAN_POINT('Ctrl Pts',(0.562636209375934,-38.27423561243,-8.56709804148113));
#61872=CARTESIAN_POINT('Ctrl Pts',(0.538853856273966,-38.2742356124619,
-8.51680672557378));
#61873=CARTESIAN_POINT('Ctrl Pts',(0.5181451821965,-38.2742356125444,-8.4652774514545));
#61874=CARTESIAN_POINT('Ctrl Pts',(0.510153982159852,-38.2742356125762,
-8.4453929945506));
#61875=CARTESIAN_POINT('Ctrl Pts',(0.502620005449637,-38.2742356126143,
-8.42532446288721));
#61876=CARTESIAN_POINT('Ctrl Pts',(0.49555124160412,-38.2742356126526,-8.40509330132935));
#61877=CARTESIAN_POINT('Ctrl Pts',(0.476947058283054,-38.2742356127534,
-8.3518471826803));
#61878=CARTESIAN_POINT('Ctrl Pts',(0.461573393384668,-38.274235612776,-8.29747876272508));
#61879=CARTESIAN_POINT('Ctrl Pts',(0.449535357169435,-38.2742356127884,
-8.24238015264472));
#61880=CARTESIAN_POINT('Ctrl Pts',(0.437781985872286,-38.2742356128005,
-8.18858446615129));
#61881=CARTESIAN_POINT('Ctrl Pts',(0.42920844174801,-38.2742356127996,-8.13409273336811));
#61882=CARTESIAN_POINT('Ctrl Pts',(0.423868058795757,-38.2742356127999,
-8.07929126394412));
#61883=CARTESIAN_POINT('Ctrl Pts',(0.420662885353337,-38.2742356128001,
-8.04640069860944));
#61884=CARTESIAN_POINT('Ctrl Pts',(0.418621474870239,-38.2742356128,-8.01339897157512));
#61885=CARTESIAN_POINT('Ctrl Pts',(0.417747123205582,-38.2742356128,-7.98037341588237));
#61886=CARTESIAN_POINT('Ctrl Pts',(0.417500472528033,-38.2742356128,-7.97105705495193));
#61887=CARTESIAN_POINT('Ctrl Pts',(0.417346628279231,-38.2742356128,-7.96173686793695));
#61888=CARTESIAN_POINT('Ctrl Pts',(0.417285628014923,-38.2742356128,-7.95241938665697));
#61889=CARTESIAN_POINT('Ctrl Pts',(0.417281041447002,-38.2742356128,-7.95171881164752));
#61890=CARTESIAN_POINT('Ctrl Pts',(0.417276979796764,-38.2742356128,-7.95101828445243));
#61891=CARTESIAN_POINT('Ctrl Pts',(0.417273442888032,-38.2742356128,-7.95031782080527));
#61892=CARTESIAN_POINT('',(0.417273426056,-38.2742356128,-3.28965091665));
#61893=CARTESIAN_POINT('',(0.417273426056,-38.2742356128,0.916320001688));
#61894=CARTESIAN_POINT('',(1.05996501343,-38.2742356128,-2.50526959142));
#61895=CARTESIAN_POINT('Ctrl Pts',(0.417273426056,-38.2742356128,-3.28965091665));
#61896=CARTESIAN_POINT('Ctrl Pts',(0.417273426056,-38.2742356128,-3.28687600563435));
#61897=CARTESIAN_POINT('Ctrl Pts',(0.417288267241563,-38.2742356128,-3.28403966420407));
#61898=CARTESIAN_POINT('Ctrl Pts',(0.417318551745409,-38.2742356128,-3.28120405870701));
#61899=CARTESIAN_POINT('Ctrl Pts',(0.417343821453037,-38.2742356128,-3.27883799974081));
#61900=CARTESIAN_POINT('Ctrl Pts',(0.417379796757908,-38.2742356128,-3.27647245778261));
#61901=CARTESIAN_POINT('Ctrl Pts',(0.417425416856367,-38.2742356128,-3.27414357493084));
#61902=CARTESIAN_POINT('Ctrl Pts',(0.41745011376523,-38.2742356128,-3.27288281027914));
#61903=CARTESIAN_POINT('Ctrl Pts',(0.417477564963489,-38.2742356128,-3.27163366066603));
#61904=CARTESIAN_POINT('Ctrl Pts',(0.417508047794076,-38.2742356128,-3.27038083299254));
#61905=CARTESIAN_POINT('Ctrl Pts',(0.417623703682738,-38.2742356128,-3.26562743919265));
#61906=CARTESIAN_POINT('Ctrl Pts',(0.417782029382677,-38.2742356128,-3.2608753558277));
#61907=CARTESIAN_POINT('Ctrl Pts',(0.417982831198984,-38.2742356128,-3.25612557957555));
#61908=CARTESIAN_POINT('Ctrl Pts',(0.419232573923149,-38.2742356128,-3.22656410238523));
#61909=CARTESIAN_POINT('Ctrl Pts',(0.422131989162464,-38.2742356128108,
-3.19706607707807));
#61910=CARTESIAN_POINT('Ctrl Pts',(0.426644322880871,-38.2742356127073,
-3.16783893396853));
#61911=CARTESIAN_POINT('Ctrl Pts',(0.431919124989423,-38.2742356125864,
-3.13367315507848));
#61912=CARTESIAN_POINT('Ctrl Pts',(0.439398461031886,-38.274235612256,-3.09987691259941));
#61913=CARTESIAN_POINT('Ctrl Pts',(0.449024112493034,-38.2742356120111,
-3.06670564901039));
#61914=CARTESIAN_POINT('Ctrl Pts',(0.452936926049543,-38.2742356119116,
-3.05322157778866));
#61915=CARTESIAN_POINT('Ctrl Pts',(0.457204357922259,-38.2742356118354,
-3.03984007280312));
#61916=CARTESIAN_POINT('Ctrl Pts',(0.461822173897898,-38.274235611817,-3.02657609664833));
#61917=CARTESIAN_POINT('Ctrl Pts',(0.474294774018725,-38.2742356117674,
-2.99075044411827));
#61918=CARTESIAN_POINT('Ctrl Pts',(0.489309772383553,-38.2742356121238,
-2.955834776464));
#61919=CARTESIAN_POINT('Ctrl Pts',(0.506727646325082,-38.2742356123874,
-2.92214655478451));
#61920=CARTESIAN_POINT('Ctrl Pts',(0.521654671661917,-38.2742356126133,
-2.89327592796457));
#61921=CARTESIAN_POINT('Ctrl Pts',(0.53834609093257,-38.2742356127471,-2.86530463487966));
#61922=CARTESIAN_POINT('Ctrl Pts',(0.55668064368847,-38.274235612782,-2.83844528990823));
#61923=CARTESIAN_POINT('Ctrl Pts',(0.568162427347117,-38.2742356128038,
-2.82162496206709));
#61924=CARTESIAN_POINT('Ctrl Pts',(0.580287959861297,-38.2742356128,-2.80524108228529));
#61925=CARTESIAN_POINT('Ctrl Pts',(0.593020083314608,-38.2742356128,-2.78935374684381));
#61926=CARTESIAN_POINT('Ctrl Pts',(0.616891823099495,-38.2742356128,-2.75956623033686));
#61927=CARTESIAN_POINT('Ctrl Pts',(0.642906462533144,-38.2742356128,-2.73151085070984));
#61928=CARTESIAN_POINT('Ctrl Pts',(0.670793009043573,-38.2742356128,-2.70545242330525));
#61929=CARTESIAN_POINT('Ctrl Pts',(0.699437797938788,-38.2742356128,-2.6786854605454));
#61930=CARTESIAN_POINT('Ctrl Pts',(0.730056969621417,-38.2742356128,-2.65402633543565));
#61931=CARTESIAN_POINT('Ctrl Pts',(0.762310842189897,-38.2742356128,-2.63173290731302));
#61932=CARTESIAN_POINT('Ctrl Pts',(0.773410204061867,-38.2742356128,-2.62406118276043));
#61933=CARTESIAN_POINT('Ctrl Pts',(0.784702809312063,-38.2742356128,-2.61666930347125));
#61934=CARTESIAN_POINT('Ctrl Pts',(0.796173849974241,-38.2742356128,-2.60956673778134));
#61935=CARTESIAN_POINT('Ctrl Pts',(0.830647647097411,-38.2742356128,-2.58822147226805));
#61936=CARTESIAN_POINT('Ctrl Pts',(0.866742606403394,-38.2742356128,-2.56948777529846));
#61937=CARTESIAN_POINT('Ctrl Pts',(0.904053286489635,-38.2742356128,-2.55358817651221));
#61938=CARTESIAN_POINT('Ctrl Pts',(0.940099610515895,-38.2742356127999,
-2.538227371284));
#61939=CARTESIAN_POINT('Ctrl Pts',(0.977279742329185,-38.2742356127999,
-2.52551220542387));
#61940=CARTESIAN_POINT('Ctrl Pts',(1.01521576655219,-38.2742356128,-2.51559656446267));
#61941=CARTESIAN_POINT('Ctrl Pts',(1.02599627385077,-38.2742356128,-2.51277877736078));
#61942=CARTESIAN_POINT('Ctrl Pts',(1.036837791067,-38.2742356128,-2.51018675230784));
#61943=CARTESIAN_POINT('Ctrl Pts',(1.04773160770174,-38.2742356128,-2.50782323579403));
#61944=CARTESIAN_POINT('Ctrl Pts',(1.05180229630503,-38.2742356128,-2.50694006141548));
#61945=CARTESIAN_POINT('Ctrl Pts',(1.05588045019742,-38.2742356128,-2.50608875312377));
#61946=CARTESIAN_POINT('Ctrl Pts',(1.05996501343,-38.2742356128,-2.50526959142));
#61947=CARTESIAN_POINT('',(2.29653396536691,-38.2742356128,-2.09683591201288));
#61948=CARTESIAN_POINT('Origin',(0.443861353289543,-38.2742356128,1.43817589094895));
#61949=CARTESIAN_POINT('',(6.27496281272,-38.2742356128,2.72284538598));
#61950=CARTESIAN_POINT('Ctrl Pts',(2.29653416635,-38.2742356128,-2.09683582206));
#61951=CARTESIAN_POINT('Ctrl Pts',(2.36220797012657,-38.2742356128,-2.06590956675441));
#61952=CARTESIAN_POINT('Ctrl Pts',(2.42765371624071,-38.2742356128,-2.03423134842919));
#61953=CARTESIAN_POINT('Ctrl Pts',(2.49302552130743,-38.2742356128,-2.00182212247038));
#61954=CARTESIAN_POINT('Ctrl Pts',(2.5004630785183,-38.2742356128,-1.99813482223471));
#61955=CARTESIAN_POINT('Ctrl Pts',(2.50789964478502,-38.2742356128,-1.99443801598111));
#61956=CARTESIAN_POINT('Ctrl Pts',(2.5153354213652,-38.2742356128,-1.99073170164066));
#61957=CARTESIAN_POINT('Ctrl Pts',(2.58810754953454,-38.2742356128,-1.95445890897253));
#61958=CARTESIAN_POINT('Ctrl Pts',(2.66068080708327,-38.2742356128,-1.91734068779584));
#61959=CARTESIAN_POINT('Ctrl Pts',(2.73288981233302,-38.2742356128,-1.879533522123));
#61960=CARTESIAN_POINT('Ctrl Pts',(2.76748989568229,-38.2742356128,-1.86141762260389));
#61961=CARTESIAN_POINT('Ctrl Pts',(2.80201510146988,-38.2742356128,-1.84313841771104));
#61962=CARTESIAN_POINT('Ctrl Pts',(2.83648773623042,-38.2742356128,-1.82468695240457));
#61963=CARTESIAN_POINT('Ctrl Pts',(2.87395812655656,-38.2742356128,-1.8046309395142));
#61964=CARTESIAN_POINT('Ctrl Pts',(2.91136644060994,-38.2742356128,-1.78437143803804));
#61965=CARTESIAN_POINT('Ctrl Pts',(2.94873835187512,-38.2742356128,-1.76389306709537));
#61966=CARTESIAN_POINT('Ctrl Pts',(3.02049221311562,-38.2742356128,-1.72457470907441));
#61967=CARTESIAN_POINT('Ctrl Pts',(3.09205299633584,-38.2742356128314,-1.68448376738218));
#61968=CARTESIAN_POINT('Ctrl Pts',(3.16330912697989,-38.2742356127677,-1.64363930500427));
#61969=CARTESIAN_POINT('Ctrl Pts',(3.24367404103224,-38.274235612696,-1.59757363067076));
#61970=CARTESIAN_POINT('Ctrl Pts',(3.3236414105591,-38.2742356125322,-1.55054807220068));
#61971=CARTESIAN_POINT('Ctrl Pts',(3.40304869483591,-38.2742356124157,-1.50252179228988));
#61972=CARTESIAN_POINT('Ctrl Pts',(3.48682359904184,-38.2742356122927,-1.45185393435296));
#61973=CARTESIAN_POINT('Ctrl Pts',(3.56997485440011,-38.2742356122232,-1.40007167360168));
#61974=CARTESIAN_POINT('Ctrl Pts',(3.65226355234279,-38.2742356122489,-1.34708967420857));
#61975=CARTESIAN_POINT('Ctrl Pts',(3.74435941007879,-38.2742356122777,-1.28779328478124));
#61976=CARTESIAN_POINT('Ctrl Pts',(3.83537474930273,-38.2742356124287,-1.22699330737691));
#61977=CARTESIAN_POINT('Ctrl Pts',(3.92491817722107,-38.2742356125816,-1.16453523334719));
#61978=CARTESIAN_POINT('Ctrl Pts',(3.94998723603213,-38.2742356126244,-1.14704913562369));
#61979=CARTESIAN_POINT('Ctrl Pts',(3.9749406287215,-38.2742356126663,-1.12943293494422));
#61980=CARTESIAN_POINT('Ctrl Pts',(3.99976913772119,-38.274235612702,-1.11168299588818));
#61981=CARTESIAN_POINT('Ctrl Pts',(4.1029832219094,-38.2742356128504,-1.03789508924876));
#61982=CARTESIAN_POINT('Ctrl Pts',(4.20409444599943,-38.2742356127998,-0.96176757421914));
#61983=CARTESIAN_POINT('Ctrl Pts',(4.3024268513798,-38.2742356128,-0.8830050686021));
#61984=CARTESIAN_POINT('Ctrl Pts',(4.33166644233314,-38.2742356128,-0.859584676943892));
#61985=CARTESIAN_POINT('Ctrl Pts',(4.36065997900015,-38.2742356128,-0.835931390211039));
#61986=CARTESIAN_POINT('Ctrl Pts',(4.38938894944612,-38.2742356128,-0.812037889005671));
#61987=CARTESIAN_POINT('Ctrl Pts',(4.47021753239654,-38.2742356128,-0.744813835578956));
#61988=CARTESIAN_POINT('Ctrl Pts',(4.54898225582855,-38.2742356128,-0.67565943355637));
#61989=CARTESIAN_POINT('Ctrl Pts',(4.62522401353323,-38.2742356128,-0.604467608051967));
#61990=CARTESIAN_POINT('Ctrl Pts',(4.66721344467678,-38.2742356128,-0.56525937958248));
#61991=CARTESIAN_POINT('Ctrl Pts',(4.70843765186859,-38.2742356128,-0.525433887573267));
#61992=CARTESIAN_POINT('Ctrl Pts',(4.74882153936151,-38.2742356128,-0.484980128874531));
#61993=CARTESIAN_POINT('Ctrl Pts',(4.80544979326116,-38.2742356128,-0.428253898167081));
#61994=CARTESIAN_POINT('Ctrl Pts',(4.86043388600898,-38.2742356128,-0.370281695042897));
#61995=CARTESIAN_POINT('Ctrl Pts',(4.9135816071207,-38.2742356128,-0.311043961171806));
#61996=CARTESIAN_POINT('Ctrl Pts',(4.96656054227607,-38.2742356128,-0.251994353853548));
#61997=CARTESIAN_POINT('Ctrl Pts',(5.01771478879239,-38.2742356128,-0.191686425068915));
#61998=CARTESIAN_POINT('Ctrl Pts',(5.06690551256612,-38.2742356128,-0.130100591119076));
#61999=CARTESIAN_POINT('Ctrl Pts',(5.11624778203621,-38.2742356128,-0.0683250248909378));
#62000=CARTESIAN_POINT('Ctrl Pts',(5.1636143955695,-38.2742356128,-0.0052628404116386));
#62001=CARTESIAN_POINT('Ctrl Pts',(5.20891710254948,-38.2742356128,0.0590936045073542));
#62002=CARTESIAN_POINT('Ctrl Pts',(5.25421980952947,-38.2742356128,0.123450049426347));
#62003=CARTESIAN_POINT('Ctrl Pts',(5.29745862035284,-38.2742356128,0.189101579445806));
#62004=CARTESIAN_POINT('Ctrl Pts',(5.3385970789696,-38.2742356128,0.256031336527183));
#62005=CARTESIAN_POINT('Ctrl Pts',(5.37557455438351,-38.2742356128,0.316191428328177));
#62006=CARTESIAN_POINT('Ctrl Pts',(5.41085446100392,-38.2742356128,0.377382687413388));
#62007=CARTESIAN_POINT('Ctrl Pts',(5.44446124996944,-38.2742356128,0.439578664361658));
#62008=CARTESIAN_POINT('Ctrl Pts',(5.47656905045249,-38.2742356128,0.499000468115407));
#62009=CARTESIAN_POINT('Ctrl Pts',(5.50714957085958,-38.2742356128,0.559339597971341));
#62010=CARTESIAN_POINT('Ctrl Pts',(5.53626992889454,-38.2742356128,0.620564294117294));
#62011=CARTESIAN_POINT('Ctrl Pts',(5.56110600265468,-38.2742356128,0.672781408604592));
#62012=CARTESIAN_POINT('Ctrl Pts',(5.58488055554933,-38.2742356128,0.725642638693521));
#62013=CARTESIAN_POINT('Ctrl Pts',(5.60766441565783,-38.2742356128,0.779121015828294));
#62014=CARTESIAN_POINT('Ctrl Pts',(5.61969038696963,-38.2742356128,0.807348428837395));
#62015=CARTESIAN_POINT('Ctrl Pts',(5.63144225779155,-38.2742356128,0.835752782091019));
#62016=CARTESIAN_POINT('Ctrl Pts',(5.64294118123923,-38.2742356128,0.86435562270076));
#62017=CARTESIAN_POINT('Ctrl Pts',(5.65633061319254,-38.2742356128,0.897660982959721));
#62018=CARTESIAN_POINT('Ctrl Pts',(5.66937655460697,-38.2742356128,0.931233997989407));
#62019=CARTESIAN_POINT('Ctrl Pts',(5.68209585008665,-38.2742356128,0.965033637032103));
#62020=CARTESIAN_POINT('Ctrl Pts',(5.69609333621808,-38.2742356128,1.00222987793265));
#62021=CARTESIAN_POINT('Ctrl Pts',(5.70969363110763,-38.2742356128,1.03969538642074));
#62022=CARTESIAN_POINT('Ctrl Pts',(5.72291809444913,-38.2742356128,1.07734587531081));
#62023=CARTESIAN_POINT('Ctrl Pts',(5.7334870169713,-38.2742356128,1.1074359507812));
#62024=CARTESIAN_POINT('Ctrl Pts',(5.74381549485532,-38.2742356128,1.13764226861823));
#62025=CARTESIAN_POINT('Ctrl Pts',(5.75392556483009,-38.2742356128,1.16794836395337));
#62026=CARTESIAN_POINT('Ctrl Pts',(5.76310014927473,-38.2742356128,1.19545023402284));
#62027=CARTESIAN_POINT('Ctrl Pts',(5.7720946772672,-38.2742356128,1.2230334474181));
#62028=CARTESIAN_POINT('Ctrl Pts',(5.78093944060798,-38.2742356128,1.25072622636446));
#62029=CARTESIAN_POINT('Ctrl Pts',(5.78906855841899,-38.2742356128,1.27617833332265));
#62030=CARTESIAN_POINT('Ctrl Pts',(5.79707109396125,-38.2742356128,1.30172265704213));
#62031=CARTESIAN_POINT('Ctrl Pts',(5.80498454924915,-38.2742356128,1.32742448428365));
#62032=CARTESIAN_POINT('Ctrl Pts',(5.8067223616598,-38.2742356128,1.33306866280388));
#62033=CARTESIAN_POINT('Ctrl Pts',(5.80845593782368,-38.2742356128,1.33872062536267));
#62034=CARTESIAN_POINT('Ctrl Pts',(5.81018578013775,-38.2742356128,1.34438139725192));
#62035=CARTESIAN_POINT('Ctrl Pts',(5.81567140688787,-38.2742356128,1.36233267607618));
#62036=CARTESIAN_POINT('Ctrl Pts',(5.82110692689557,-38.2742356127995,1.38032842460541));
#62037=CARTESIAN_POINT('Ctrl Pts',(5.82650005324596,-38.2742356127995,1.39836590318722));
#62038=CARTESIAN_POINT('Ctrl Pts',(5.82697260131895,-38.2742356127996,1.39994635489403));
#62039=CARTESIAN_POINT('Ctrl Pts',(5.82744483120366,-38.2742356127996,1.4015271585344));
#62040=CARTESIAN_POINT('Ctrl Pts',(5.82791675210203,-38.2742356127996,1.40310832963793));
#62041=CARTESIAN_POINT('Ctrl Pts',(5.83360773127681,-38.2742356127999,1.4221759569734));
#62042=CARTESIAN_POINT('Ctrl Pts',(5.83924444553751,-38.2742356127999,1.44126285712189));
#62043=CARTESIAN_POINT('Ctrl Pts',(5.84480916037222,-38.2742356128,1.46027646702416));
#62044=CARTESIAN_POINT('Ctrl Pts',(5.85080823572841,-38.2742356128,1.48077420715733));
#62045=CARTESIAN_POINT('Ctrl Pts',(5.85672364156798,-38.2742356128,1.50118680709605));
#62046=CARTESIAN_POINT('Ctrl Pts',(5.86255182978096,-38.2742356128,1.52146040862887));
#62047=CARTESIAN_POINT('Ctrl Pts',(5.86801153465465,-38.2742356128,1.54045222513357));
#62048=CARTESIAN_POINT('Ctrl Pts',(5.87339510515199,-38.2742356128,1.55932342003616));
#62049=CARTESIAN_POINT('Ctrl Pts',(5.87871159455216,-38.2742356128,1.57806935091714));
#62050=CARTESIAN_POINT('Ctrl Pts',(5.88587811874549,-38.2742356128,1.60333850074009));
#62051=CARTESIAN_POINT('Ctrl Pts',(5.89292575369051,-38.2742356128,1.6283904733301));
#62052=CARTESIAN_POINT('Ctrl Pts',(5.8999252541189,-38.2742356128,1.65338209442216));
#62053=CARTESIAN_POINT('Ctrl Pts',(5.9087612742733,-38.2742356128,1.68493098422072));
#62054=CARTESIAN_POINT('Ctrl Pts',(5.91752179783635,-38.2742356128,1.71638910609064));
#62055=CARTESIAN_POINT('Ctrl Pts',(5.92636835988832,-38.2742356128,1.74812750090717));
#62056=CARTESIAN_POINT('Ctrl Pts',(5.93257015502608,-38.2742356128,1.7703773897902));
#62057=CARTESIAN_POINT('Ctrl Pts',(5.93881483092627,-38.2742356128,1.79276689613811));
#62058=CARTESIAN_POINT('Ctrl Pts',(5.94515464644725,-38.2742356128,1.81540405784503));
#62059=CARTESIAN_POINT('Ctrl Pts',(5.9510135097083,-38.2742356128,1.83632391499546));
#62060=CARTESIAN_POINT('Ctrl Pts',(5.95695343702594,-38.2742356128,1.85745455864831));
#62061=CARTESIAN_POINT('Ctrl Pts',(5.96300290943211,-38.2742356128,1.87882926010439));
#62062=CARTESIAN_POINT('Ctrl Pts',(5.96868836264847,-38.2742356128,1.89891776650344));
#62063=CARTESIAN_POINT('Ctrl Pts',(5.97447073827174,-38.2742356128,1.91922240784038));
#62064=CARTESIAN_POINT('Ctrl Pts',(5.98036338205917,-38.2742356128,1.93972857692636));
#62065=CARTESIAN_POINT('Ctrl Pts',(5.98585680097295,-38.2742356128,1.95884545912217));
#62066=CARTESIAN_POINT('Ctrl Pts',(5.99144611848614,-38.2742356128,1.97813769237131));
#62067=CARTESIAN_POINT('Ctrl Pts',(5.99713141052935,-38.2742356128,1.99755056933384));
#62068=CARTESIAN_POINT('Ctrl Pts',(6.00188504763554,-38.2742356128,2.01378223721752));
#62069=CARTESIAN_POINT('Ctrl Pts',(6.00670564982786,-38.2742356128,2.03009770750313));
#62070=CARTESIAN_POINT('Ctrl Pts',(6.01158632787636,-38.2742356128,2.04643771535537));
#62071=CARTESIAN_POINT('Ctrl Pts',(6.02553662212153,-38.2742356128,2.09314186491048));
#62072=CARTESIAN_POINT('Ctrl Pts',(6.03996335521539,-38.2742356128,2.1400074331509));
#62073=CARTESIAN_POINT('Ctrl Pts',(6.05510272454428,-38.2742356128,2.18697705047249));
#62074=CARTESIAN_POINT('Ctrl Pts',(6.0707480680562,-38.2742356128,2.23551644347202));
#62075=CARTESIAN_POINT('Ctrl Pts',(6.08715459885474,-38.2742356128,2.28416696934139));
#62076=CARTESIAN_POINT('Ctrl Pts',(6.10461272043758,-38.2742356128,2.33281749388226));
#62077=CARTESIAN_POINT('Ctrl Pts',(6.12243742488736,-38.2742356128,2.38248957441811));
#62078=CARTESIAN_POINT('Ctrl Pts',(6.14135856879351,-38.2742356128,2.43216154123912));
#62079=CARTESIAN_POINT('Ctrl Pts',(6.16171298081537,-38.2742356128,2.4816669788947));
#62080=CARTESIAN_POINT('Ctrl Pts',(6.18281606494677,-38.2742356128,2.53299331613722));
#62081=CARTESIAN_POINT('Ctrl Pts',(6.20546001019525,-38.2742356128,2.58414062053214));
#62082=CARTESIAN_POINT('Ctrl Pts',(6.23004640194285,-38.2742356128,2.63487313183816));
#62083=CARTESIAN_POINT('Ctrl Pts',(6.24412952051531,-38.2742356128,2.66393278319065));
#62084=CARTESIAN_POINT('Ctrl Pts',(6.25885041805261,-38.2742356128,2.69285542631629));
#62085=CARTESIAN_POINT('Ctrl Pts',(6.27428775967426,-38.2742356128,2.7215898409063));
#62086=CARTESIAN_POINT('Ctrl Pts',(6.2745126230389,-38.2742356128,2.72200839206001));
#62087=CARTESIAN_POINT('Ctrl Pts',(6.27473763842,-38.2742356128,2.72242690309667));
#62088=CARTESIAN_POINT('Ctrl Pts',(6.27496281272,-38.2742356128,2.72284538598));
#62089=CARTESIAN_POINT('',(9.72829290598,-38.2742356128,2.64854903634));
#62090=CARTESIAN_POINT('Ctrl Pts',(6.27496281272,-38.2742356128,2.72284538598));
#62091=CARTESIAN_POINT('Ctrl Pts',(6.28175989394697,-38.2742356128,2.73547766265914));
#62092=CARTESIAN_POINT('Ctrl Pts',(6.28867511539028,-38.2742356128,2.74803334580149));
#62093=CARTESIAN_POINT('Ctrl Pts',(6.29570579837365,-38.2742356128,2.7605119793025));
#62094=CARTESIAN_POINT('Ctrl Pts',(6.31679767088927,-38.2742356128,2.79794756665514));
#62095=CARTESIAN_POINT('Ctrl Pts',(6.33892929501013,-38.2742356128,2.8346928281563));
#62096=CARTESIAN_POINT('Ctrl Pts',(6.36204152758071,-38.2742356128,2.87074139528003));
#62097=CARTESIAN_POINT('Ctrl Pts',(6.39312958850154,-38.2742356128,2.91923000612405));
#62098=CARTESIAN_POINT('Ctrl Pts',(6.42599242410214,-38.2742356128005,2.96646286247323));
#62099=CARTESIAN_POINT('Ctrl Pts',(6.46053080560081,-38.274235612799,3.01241529465755));
#62100=CARTESIAN_POINT('Ctrl Pts',(6.49461335324637,-38.2742356127974,3.05776125157252));
#62101=CARTESIAN_POINT('Ctrl Pts',(6.53032758958246,-38.2742356127949,3.10186048887922));
#62102=CARTESIAN_POINT('Ctrl Pts',(6.56761546044982,-38.274235612774,3.1446555715695));
#62103=CARTESIAN_POINT('Ctrl Pts',(6.60490333131718,-38.274235612753,3.18745065425978));
#62104=CARTESIAN_POINT('Ctrl Pts',(6.64376481920528,-38.2742356127153,3.22894179606692));
#62105=CARTESIAN_POINT('Ctrl Pts',(6.68417908704671,-38.2742356126072,3.26903493627089));
#62106=CARTESIAN_POINT('Ctrl Pts',(6.72499216754563,-38.2742356124981,3.30952372020778));
#62107=CARTESIAN_POINT('Ctrl Pts',(6.76739214163738,-38.2742356125106,3.34859605472038));
#62108=CARTESIAN_POINT('Ctrl Pts',(6.81138643758061,-38.2742356125827,3.38610169378874));
#62109=CARTESIAN_POINT('Ctrl Pts',(6.85538073352383,-38.2742356126549,3.4236073328571));
#62110=CARTESIAN_POINT('Ctrl Pts',(6.90096932910499,-38.2742356127469,3.45954646193985));
#62111=CARTESIAN_POINT('Ctrl Pts',(6.94819533003811,-38.2742356127783,3.49372702645337));
#62112=CARTESIAN_POINT('Ctrl Pts',(6.99542200208882,-38.2742356128096,3.52790807669885));
#62113=CARTESIAN_POINT('Ctrl Pts',(7.04429746417697,-38.2742356128,3.56033518713764));
#62114=CARTESIAN_POINT('Ctrl Pts',(7.09483438027948,-38.2742356128,3.59073893044824));
#62115=CARTESIAN_POINT('Ctrl Pts',(7.12010478766847,-38.2742356128,3.60594197485347));
#62116=CARTESIAN_POINT('Ctrl Pts',(7.1457927882084,-38.2742356128,3.62063995899852));
#62117=CARTESIAN_POINT('Ctrl Pts',(7.17190833253584,-38.2742356128,3.63479573700106));
#62118=CARTESIAN_POINT('Ctrl Pts',(7.21559274834165,-38.2742356128,3.65847461899427));
#62119=CARTESIAN_POINT('Ctrl Pts',(7.26049747083368,-38.2742356128,3.68064523031944));
#62120=CARTESIAN_POINT('Ctrl Pts',(7.30649486896597,-38.2742356128,3.70105528680162));
#62121=CARTESIAN_POINT('Ctrl Pts',(7.35087125777577,-38.2742356128,3.72074606582086));
#62122=CARTESIAN_POINT('Ctrl Pts',(7.3962665568332,-38.2742356128,3.73879895785097));
#62123=CARTESIAN_POINT('Ctrl Pts',(7.44252054843875,-38.2742356128,3.75500665859511));
#62124=CARTESIAN_POINT('Ctrl Pts',(7.49474913383961,-38.2742356128,3.77330789602529));
#62125=CARTESIAN_POINT('Ctrl Pts',(7.54806637498204,-38.2742356128,3.78925398043707));
#62126=CARTESIAN_POINT('Ctrl Pts',(7.60222777550352,-38.2742356128,3.80259777613426));
#62127=CARTESIAN_POINT('Ctrl Pts',(7.63544961672591,-38.2742356128,3.81078267271537));
#62128=CARTESIAN_POINT('Ctrl Pts',(7.66898820965766,-38.2742356128,3.81798915253491));
#62129=CARTESIAN_POINT('Ctrl Pts',(7.70277859341121,-38.2742356128,3.82416796478963));
#62130=CARTESIAN_POINT('Ctrl Pts',(7.72631962642329,-38.2742356128,3.82847261028655));
#62131=CARTESIAN_POINT('Ctrl Pts',(7.74998525345287,-38.2742356128,3.83227917534982));
#62132=CARTESIAN_POINT('Ctrl Pts',(7.77376022135309,-38.2742356128,3.83557357412904));
#62133=CARTESIAN_POINT('Ctrl Pts',(7.82237592899862,-38.2742356128,3.84231005127553));
#62134=CARTESIAN_POINT('Ctrl Pts',(7.87143743462109,-38.2742356128,3.84689957799316));
#62135=CARTESIAN_POINT('Ctrl Pts',(7.9207084710963,-38.2742356128,3.84923698483134));
#62136=CARTESIAN_POINT('Ctrl Pts',(7.96871304847685,-38.2742356128,3.85151431113621));
#62137=CARTESIAN_POINT('Ctrl Pts',(8.01691594294803,-38.2742356128,3.85165340893818));
#62138=CARTESIAN_POINT('Ctrl Pts',(8.06508596156888,-38.2742356128,3.84960442308835));
#62139=CARTESIAN_POINT('Ctrl Pts',(8.11160303203354,-38.2742356128,3.84762574793133));
#62140=CARTESIAN_POINT('Ctrl Pts',(8.15808896531939,-38.2742356128,3.84360638048735));
#62141=CARTESIAN_POINT('Ctrl Pts',(8.20433122212088,-38.2742356128,3.83755036990893));
#62142=CARTESIAN_POINT('Ctrl Pts',(8.21146146922977,-38.2742356128,3.83661657353079));
#62143=CARTESIAN_POINT('Ctrl Pts',(8.21858592202528,-38.2742356128,3.83563445576886));
#62144=CARTESIAN_POINT('Ctrl Pts',(8.22570380264635,-38.2742356128,3.83460414414139));
#62145=CARTESIAN_POINT('Ctrl Pts',(8.26916917773586,-38.2742356128,3.82831254082139));
#62146=CARTESIAN_POINT('Ctrl Pts',(8.31238904500106,-38.2742356128,3.82022080412619));
#62147=CARTESIAN_POINT('Ctrl Pts',(8.35515073174464,-38.2742356128,3.8103893337697));
#62148=CARTESIAN_POINT('Ctrl Pts',(8.39587250007142,-38.2742356128,3.80102686730364));
#62149=CARTESIAN_POINT('Ctrl Pts',(8.43617935502698,-38.2742356128,3.79008717922198));
#62150=CARTESIAN_POINT('Ctrl Pts',(8.47592446037656,-38.2742356128,3.77764625378023));
#62151=CARTESIAN_POINT('Ctrl Pts',(8.51817884137633,-38.2742356128,3.76441988039459));
#62152=CARTESIAN_POINT('Ctrl Pts',(8.55978146889371,-38.2742356128,3.7495011054138));
#62153=CARTESIAN_POINT('Ctrl Pts',(8.6005665880081,-38.2742356128,3.73302424017688));
#62154=CARTESIAN_POINT('Ctrl Pts',(8.63470715191798,-38.2742356128,3.71923172263934));
#62155=CARTESIAN_POINT('Ctrl Pts',(8.66827574390385,-38.2742356128,3.70434819246818));
#62156=CARTESIAN_POINT('Ctrl Pts',(8.70119857853243,-38.2742356128,3.68846751861937));
#62157=CARTESIAN_POINT('Ctrl Pts',(8.73601365099068,-38.2742356128,3.67167410404952));
#62158=CARTESIAN_POINT('Ctrl Pts',(8.77011496511053,-38.2742356128,3.65376173724068));
#62159=CARTESIAN_POINT('Ctrl Pts',(8.80344116958025,-38.2742356128,3.63485089925167));
#62160=CARTESIAN_POINT('Ctrl Pts',(8.83063668774854,-38.2742356128,3.61941889772942));
#62161=CARTESIAN_POINT('Ctrl Pts',(8.85731345058671,-38.2742356128,3.60332407304967));
#62162=CARTESIAN_POINT('Ctrl Pts',(8.88345088080642,-38.2742356128,3.58663584779668));
#62163=CARTESIAN_POINT('Ctrl Pts',(8.9259593054728,-38.2742356128,3.55949507075703));
#62164=CARTESIAN_POINT('Ctrl Pts',(8.96705449595305,-38.2742356128,3.53077491258169));
#62165=CARTESIAN_POINT('Ctrl Pts',(9.00671405321108,-38.2742356128,3.50076505793843));
#62166=CARTESIAN_POINT('Ctrl Pts',(9.02448445149716,-38.2742356128,3.48731843608009));
#62167=CARTESIAN_POINT('Ctrl Pts',(9.0419679384425,-38.2742356128,3.47361257263251));
#62168=CARTESIAN_POINT('Ctrl Pts',(9.05917102804987,-38.2742356128,3.45966884100842));
#62169=CARTESIAN_POINT('Ctrl Pts',(9.09613287534507,-38.2742356128,3.42970991556087));
#62170=CARTESIAN_POINT('Ctrl Pts',(9.13178298861802,-38.2742356128,3.39866330865085));
#62171=CARTESIAN_POINT('Ctrl Pts',(9.16610497039632,-38.2742356128,3.36683543275146));
#62172=CARTESIAN_POINT('Ctrl Pts',(9.19617038556613,-38.2742356128,3.33895480776106));
#62173=CARTESIAN_POINT('Ctrl Pts',(9.22522040844852,-38.2742356128,3.31047255605014));
#62174=CARTESIAN_POINT('Ctrl Pts',(9.2532655075239,-38.2742356128,3.28159842813157));
#62175=CARTESIAN_POINT('Ctrl Pts',(9.26335772601788,-38.2742356128,3.27120787800393));
#62176=CARTESIAN_POINT('Ctrl Pts',(9.27331759521306,-38.2742356128,3.26076909600295));
#62177=CARTESIAN_POINT('Ctrl Pts',(9.28315033923572,-38.2742356128,3.25028745674481));
#62178=CARTESIAN_POINT('Ctrl Pts',(9.28944952698189,-38.2742356128,3.24357256480595));
#62179=CARTESIAN_POINT('Ctrl Pts',(9.29569777098763,-38.2742356128,3.23683882068643));
#62180=CARTESIAN_POINT('Ctrl Pts',(9.30190371288055,-38.2742356128,3.23007938120359));
#62181=CARTESIAN_POINT('Ctrl Pts',(9.33233023873494,-38.2742356128,3.19693916433808));
#62182=CARTESIAN_POINT('Ctrl Pts',(9.36168036792281,-38.2742356128,3.163242504528));
#62183=CARTESIAN_POINT('Ctrl Pts',(9.38997095611936,-38.2742356128,3.12926408303275));
#62184=CARTESIAN_POINT('Ctrl Pts',(9.4175861925723,-38.2742356128,3.09609679300081));
#62185=CARTESIAN_POINT('Ctrl Pts',(9.44419272126028,-38.2742356128,3.06266214394091));
#62186=CARTESIAN_POINT('Ctrl Pts',(9.46984227971996,-38.2742356128,3.0291824106293));
#62187=CARTESIAN_POINT('Ctrl Pts',(9.48358594054153,-38.2742356128,3.01124315059272));
#62188=CARTESIAN_POINT('Ctrl Pts',(9.49705539415298,-38.2742356128,2.99329026953402));
#62189=CARTESIAN_POINT('Ctrl Pts',(9.51026170167303,-38.2742356128,2.97535239382229));
#62190=CARTESIAN_POINT('Ctrl Pts',(9.52286799378051,-38.2742356128,2.95822950760549));
#62191=CARTESIAN_POINT('Ctrl Pts',(9.53522797161959,-38.2742356128,2.94113004374477));
#62192=CARTESIAN_POINT('Ctrl Pts',(9.54740400575136,-38.2742356128,2.92400110327784));
#62193=CARTESIAN_POINT('Ctrl Pts',(9.56979774633823,-38.2742356128,2.89249814876958));
#62194=CARTESIAN_POINT('Ctrl Pts',(9.59154723077383,-38.2742356128,2.86092587153871));
#62195=CARTESIAN_POINT('Ctrl Pts',(9.61272092465214,-38.2742356128,2.82935643568641));
#62196=CARTESIAN_POINT('Ctrl Pts',(9.63294559994359,-38.2742356128,2.79920196226685));
#62197=CARTESIAN_POINT('Ctrl Pts',(9.65264538214872,-38.2742356128,2.76905020393921));
#62198=CARTESIAN_POINT('Ctrl Pts',(9.67188544590519,-38.2742356128,2.73891828907923));
#62199=CARTESIAN_POINT('Ctrl Pts',(9.68150547778342,-38.2742356128,2.72385233164924));
#62200=CARTESIAN_POINT('Ctrl Pts',(9.69101062804654,-38.2742356128,2.7087905913421));
#62201=CARTESIAN_POINT('Ctrl Pts',(9.70040909814045,-38.2742356128,2.69373054093805));
#62202=CARTESIAN_POINT('Ctrl Pts',(9.70510833318741,-38.2742356128,2.68620051573602));
#62203=CARTESIAN_POINT('Ctrl Pts',(9.70978089686981,-38.2742356128,2.67867086274479));
#62204=CARTESIAN_POINT('Ctrl Pts',(9.71442779933124,-38.2742356128,2.67114095997344));
#62205=CARTESIAN_POINT('Ctrl Pts',(9.71734973513711,-38.2742356128,2.66640621619413));
#62206=CARTESIAN_POINT('Ctrl Pts',(9.72026152477054,-38.2742356128,2.66167136955722));
#62207=CARTESIAN_POINT('Ctrl Pts',(9.72316341608076,-38.2742356128,2.65693622339584));
#62208=CARTESIAN_POINT('Ctrl Pts',(9.7248765494556,-38.2742356128,2.65414082685731));
#62209=CARTESIAN_POINT('Ctrl Pts',(9.72658528778543,-38.2742356128,2.65134687498826));
#62210=CARTESIAN_POINT('Ctrl Pts',(9.72829290598,-38.2742356128,2.64854903634));
#62211=CARTESIAN_POINT('Ctrl Pts',(9.72829290598,-38.2742356128,2.64854903634));
#62212=CARTESIAN_POINT('Ctrl Pts',(9.73633081950354,-38.2742356128,2.63537941280583));
#62213=CARTESIAN_POINT('Ctrl Pts',(9.74437282162921,-38.2742356128,2.62207734293453));
#62214=CARTESIAN_POINT('Ctrl Pts',(9.75239609347846,-38.2742356128,2.60866170311115));
#62215=CARTESIAN_POINT('Ctrl Pts',(9.7706178726226,-38.2742356128,2.57819323207684));
#62216=CARTESIAN_POINT('Ctrl Pts',(9.78873121305153,-38.2742356128045,2.54715338833482));
#62217=CARTESIAN_POINT('Ctrl Pts',(9.80656454330723,-38.2742356127903,2.51565633011237));
#62218=CARTESIAN_POINT('Ctrl Pts',(9.82522540644807,-38.2742356127755,2.48269769118174));
#62219=CARTESIAN_POINT('Ctrl Pts',(9.84357974189825,-38.2742356127495,2.44923836084657));
#62220=CARTESIAN_POINT('Ctrl Pts',(9.8614863558543,-38.2742356125523,2.41538824559926));
#62221=CARTESIAN_POINT('Ctrl Pts',(9.87920707925459,-38.2742356123572,2.38188953217205));
#62222=CARTESIAN_POINT('Ctrl Pts',(9.89648992214151,-38.2742356120062,2.34800784985536));
#62223=CARTESIAN_POINT('Ctrl Pts',(9.91324521507938,-38.2742356110565,2.31383240769414));
#62224=CARTESIAN_POINT('Ctrl Pts',(9.93224345730128,-38.2742356099796,2.27508206589903));
#62225=CARTESIAN_POINT('Ctrl Pts',(9.95057689163532,-38.2742356082693,2.2359335436681));
#62226=CARTESIAN_POINT('Ctrl Pts',(9.96819415283343,-38.2742356072486,2.19645698119026));
#62227=CARTESIAN_POINT('Ctrl Pts',(9.97735837586944,-38.2742356067177,2.17592189238311));
#62228=CARTESIAN_POINT('Ctrl Pts',(9.98632969007421,-38.2742356064057,2.15529765960282));
#62229=CARTESIAN_POINT('Ctrl Pts',(9.99510586294375,-38.2742356065093,2.13459208982059));
#62230=CARTESIAN_POINT('Ctrl Pts',(10.007929849719,-38.2742356066606,2.10433653799763));
#62231=CARTESIAN_POINT('Ctrl Pts',(10.0203432583176,-38.2742356075538,2.07388879803855));
#62232=CARTESIAN_POINT('Ctrl Pts',(10.032324733776,-38.2742356086601,2.04332373370437));
#62233=CARTESIAN_POINT('Ctrl Pts',(10.0443062092338,-38.2742356097665,2.01275866937166));
#62234=CARTESIAN_POINT('Ctrl Pts',(10.0558513452567,-38.2742356112677,1.98209385668015));
#62235=CARTESIAN_POINT('Ctrl Pts',(10.0669588760154,-38.2742356120342,1.95138103326328));
#62236=CARTESIAN_POINT('Ctrl Pts',(10.0891452831127,-38.2742356135653,1.89003461719298));
#62237=CARTESIAN_POINT('Ctrl Pts',(10.1095692104436,-38.2742356128,1.82848655467785));
#62238=CARTESIAN_POINT('Ctrl Pts',(10.128456408996,-38.2742356128,1.76681870077139));
#62239=CARTESIAN_POINT('Ctrl Pts',(10.1379001404091,-38.2742356128,1.73598434238294));
#62240=CARTESIAN_POINT('Ctrl Pts',(10.14696167855,-38.2742356128,1.70511412639515));
#62241=CARTESIAN_POINT('Ctrl Pts',(10.1556583365498,-38.2742356128,1.67424279728339));
#62242=CARTESIAN_POINT('Ctrl Pts',(10.16435499455,-38.2742356128,1.64337146817015));
#62243=CARTESIAN_POINT('Ctrl Pts',(10.1726823665861,-38.2742356128,1.61251259232094));
#62244=CARTESIAN_POINT('Ctrl Pts',(10.1806640744349,-38.2742356128,1.58173198537152));
#62245=CARTESIAN_POINT('Ctrl Pts',(10.1922325743438,-38.2742356128,1.53711929652927));
#62246=CARTESIAN_POINT('Ctrl Pts',(10.203080052512,-38.2742356128,1.49265202704484));
#62247=CARTESIAN_POINT('Ctrl Pts',(10.2133104720004,-38.2742356128,1.44845116652768));
#62248=CARTESIAN_POINT('Ctrl Pts',(10.2231958315931,-38.2742356128,1.40574114852592));
#62249=CARTESIAN_POINT('Ctrl Pts',(10.2325058502182,-38.2742356128,1.36328013780716));
#62250=CARTESIAN_POINT('Ctrl Pts',(10.2413469161846,-38.2742356128,1.32113143513957));
#62251=CARTESIAN_POINT('Ctrl Pts',(10.248425021219,-38.2742356128,1.28738743349139));
#62252=CARTESIAN_POINT('Ctrl Pts',(10.2552029211007,-38.2742356128,1.25384284282264));
#62253=CARTESIAN_POINT('Ctrl Pts',(10.2617364169019,-38.2742356128,1.22050596333499));
#62254=CARTESIAN_POINT('Ctrl Pts',(10.2694791647119,-38.2742356128,1.18099892782147));
#62255=CARTESIAN_POINT('Ctrl Pts',(10.2768783835795,-38.2742356128,1.14178928445506));
#62256=CARTESIAN_POINT('Ctrl Pts',(10.2840216413865,-38.2742356128,1.10284902512591));
#62257=CARTESIAN_POINT('Ctrl Pts',(10.2908559963421,-38.2742356128,1.06559269733981));
#62258=CARTESIAN_POINT('Ctrl Pts',(10.2974564253937,-38.2742356128,1.02858294877892));
#62259=CARTESIAN_POINT('Ctrl Pts',(10.3038885583826,-38.2742356128,0.991749116652807));
#62260=CARTESIAN_POINT('Ctrl Pts',(10.310175485487,-38.2742356128,0.955746811048525));
#62261=CARTESIAN_POINT('Ctrl Pts',(10.3163019642676,-38.2742356128,0.919912681263671));
#62262=CARTESIAN_POINT('Ctrl Pts',(10.3223133025257,-38.2742356128,0.884134704814115));
#62263=CARTESIAN_POINT('Ctrl Pts',(10.3281353526992,-38.2742356128,0.849483323531461));
#62264=CARTESIAN_POINT('Ctrl Pts',(10.3338496369459,-38.2742356128,0.814884622669424));
#62265=CARTESIAN_POINT('Ctrl Pts',(10.3394780744938,-38.2742356128,0.780192405435676));
#62266=CARTESIAN_POINT('Ctrl Pts',(10.3433361101194,-38.2742356128,0.756412482698574));
#62267=CARTESIAN_POINT('Ctrl Pts',(10.3471534165005,-38.2742356128,0.73258771295533));
#62268=CARTESIAN_POINT('Ctrl Pts',(10.3509307018976,-38.2742356128,0.708658267877187));
#62269=CARTESIAN_POINT('Ctrl Pts',(10.3517926022542,-38.2742356128,0.703198051061031));
#62270=CARTESIAN_POINT('Ctrl Pts',(10.3526516477296,-38.2742356128,0.697737184145745));
#62271=CARTESIAN_POINT('Ctrl Pts',(10.3535092619,-38.2742356128,0.692265445118));
#62272=CARTESIAN_POINT('',(-2.11954040870134,-38.2742356128,-9.31090046842523));
#62273=CARTESIAN_POINT('',(-10.3535102065,-38.2742356128,0.692259352582));
#62274=CARTESIAN_POINT('Ctrl Pts',(-2.119540611027,-38.2742356128,-9.31090043155947));
#62275=CARTESIAN_POINT('Ctrl Pts',(-2.13364472791917,-38.2742356128,-9.3083306064183));
#62276=CARTESIAN_POINT('Ctrl Pts',(-2.14773674018183,-38.2742356128,-9.30573625661834));
#62277=CARTESIAN_POINT('Ctrl Pts',(-2.16182796614952,-38.2742356128,-9.30311552892601));
#62278=CARTESIAN_POINT('Ctrl Pts',(-2.32376865139767,-38.2742356127999,
-9.27299732350397));
#62279=CARTESIAN_POINT('Ctrl Pts',(-2.48495687112191,-38.2742356127996,
-9.239499459851));
#62280=CARTESIAN_POINT('Ctrl Pts',(-2.64515420185416,-38.2742356127995,
-9.20256165403099));
#62281=CARTESIAN_POINT('Ctrl Pts',(-2.80768594553618,-38.2742356127993,
-9.16508558648185));
#62282=CARTESIAN_POINT('Ctrl Pts',(-2.96919808080522,-38.2742356127992,
-9.12406802380528));
#62283=CARTESIAN_POINT('Ctrl Pts',(-3.1294916921194,-38.2742356127992,-9.07946595465591));
#62284=CARTESIAN_POINT('Ctrl Pts',(-3.29639584579064,-38.2742356127992,
-9.03302448676254));
#62285=CARTESIAN_POINT('Ctrl Pts',(-3.46197915083997,-38.2742356127993,
-8.98269593782396));
#62286=CARTESIAN_POINT('Ctrl Pts',(-3.62606644740541,-38.2742356127994,
-8.92846416277601));
#62287=CARTESIAN_POINT('Ctrl Pts',(-3.78404198900947,-38.2742356127996,
-8.87625235714162));
#62288=CARTESIAN_POINT('Ctrl Pts',(-3.94063166288899,-38.2742356127997,
-8.82042234815021));
#62289=CARTESIAN_POINT('Ctrl Pts',(-4.09571540570172,-38.2742356127998,
-8.76099703017426));
#62290=CARTESIAN_POINT('Ctrl Pts',(-4.24910473352082,-38.2742356127999,
-8.70222098173459));
#62291=CARTESIAN_POINT('Ctrl Pts',(-4.40102139726561,-38.2742356127999,
-8.63992732111316));
#62292=CARTESIAN_POINT('Ctrl Pts',(-4.55137602984186,-38.2742356128,-8.57418123317398));
#62293=CARTESIAN_POINT('Ctrl Pts',(-4.69850394264876,-38.2742356128,-8.50984610409968));
#62294=CARTESIAN_POINT('Ctrl Pts',(-4.84413666293673,-38.2742356128,-8.4422048415258));
#62295=CARTESIAN_POINT('Ctrl Pts',(-4.98820847473103,-38.2742356128,-8.37136522774251));
#62296=CARTESIAN_POINT('Ctrl Pts',(-5.01189799059617,-38.2742356128,-8.35971717436067));
#62297=CARTESIAN_POINT('Ctrl Pts',(-5.03554533520149,-38.2742356128,-8.34798275813522));
#62298=CARTESIAN_POINT('Ctrl Pts',(-5.05915024982113,-38.2742356128,-8.33616259113913));
#62299=CARTESIAN_POINT('Ctrl Pts',(-5.19613226349434,-38.2742356128,-8.26756881297181));
#62300=CARTESIAN_POINT('Ctrl Pts',(-5.33169516861775,-38.2742356128,-8.19607801844391));
#62301=CARTESIAN_POINT('Ctrl Pts',(-5.46577814671631,-38.2742356128,-8.12182944272581));
#62302=CARTESIAN_POINT('Ctrl Pts',(-5.61311054623041,-38.2742356128,-8.04024398738926));
#62303=CARTESIAN_POINT('Ctrl Pts',(-5.75865383549873,-38.2742356128,-7.95533085578545));
#62304=CARTESIAN_POINT('Ctrl Pts',(-5.90234076261512,-38.2742356128,-7.86732671859547));
#62305=CARTESIAN_POINT('Ctrl Pts',(-6.02299132476987,-38.2742356128,-7.79343169671003));
#62306=CARTESIAN_POINT('Ctrl Pts',(-6.14232928483772,-38.2742356128,-7.71736146010781));
#62307=CARTESIAN_POINT('Ctrl Pts',(-6.26035030960864,-38.2742356128,-7.63925451488464));
#62308=CARTESIAN_POINT('Ctrl Pts',(-6.37527408486149,-38.2742356128,-7.56319734595277));
#62309=CARTESIAN_POINT('Ctrl Pts',(-6.4889488059138,-38.2742356128,-7.48520986313824));
#62310=CARTESIAN_POINT('Ctrl Pts',(-6.60140601560954,-38.2742356128,-7.40540258312093));
#62311=CARTESIAN_POINT('Ctrl Pts',(-6.65006200218209,-38.2742356128,-7.37087298777154));
#62312=CARTESIAN_POINT('Ctrl Pts',(-6.69849058187879,-38.2742356128,-7.33600241844901));
#62313=CARTESIAN_POINT('Ctrl Pts',(-6.74669690172057,-38.2742356128,-7.30079801871046));
#62314=CARTESIAN_POINT('Ctrl Pts',(-6.82975104074592,-38.2742356128,-7.24014474503625));
#62315=CARTESIAN_POINT('Ctrl Pts',(-6.9121479426546,-38.2742356128,-7.17849976034897));
#62316=CARTESIAN_POINT('Ctrl Pts',(-6.99396258843833,-38.2742356128,-7.11583561689136));
#62317=CARTESIAN_POINT('Ctrl Pts',(-7.03977098542883,-38.2742356128,-7.08074967435529));
#62318=CARTESIAN_POINT('Ctrl Pts',(-7.0853959556089,-38.2742356128,-7.04534466400566));
#62319=CARTESIAN_POINT('Ctrl Pts',(-7.13084411519291,-38.2742356128,-7.00961848116238));
#62320=CARTESIAN_POINT('Ctrl Pts',(-7.17503106878152,-38.2742356128,-6.97488371527431));
#62321=CARTESIAN_POINT('Ctrl Pts',(-7.21905664702566,-38.2742356128,-6.93984085852948));
#62322=CARTESIAN_POINT('Ctrl Pts',(-7.26292627354035,-38.2742356128,-6.90448613736163));
#62323=CARTESIAN_POINT('Ctrl Pts',(-7.35159910518294,-38.2742356128,-6.83302431999608));
#62324=CARTESIAN_POINT('Ctrl Pts',(-7.43963202886674,-38.2742356128,-6.76029286715303));
#62325=CARTESIAN_POINT('Ctrl Pts',(-7.52698205911756,-38.2742356128,-6.68630420512345));
#62326=CARTESIAN_POINT('Ctrl Pts',(-7.61357936644008,-38.2742356128,-6.61295312687243));
#62327=CARTESIAN_POINT('Ctrl Pts',(-7.699504982201,-38.2742356128,-6.53836760366721));
#62328=CARTESIAN_POINT('Ctrl Pts',(-7.78468609109267,-38.2742356128,-6.46254133509157));
#62329=CARTESIAN_POINT('Ctrl Pts',(-7.87064681191647,-38.2742356128,-6.38602107386287));
#62330=CARTESIAN_POINT('Ctrl Pts',(-7.95584901699601,-38.2742356128,-6.30823809256242));
#62331=CARTESIAN_POINT('Ctrl Pts',(-8.04016575030431,-38.2742356128,-6.22917475735306));
#62332=CARTESIAN_POINT('Ctrl Pts',(-8.12178277687235,-38.2742356128,-6.15264292224573));
#62333=CARTESIAN_POINT('Ctrl Pts',(-8.20256954986649,-38.2742356128,-6.07491203715707));
#62334=CARTESIAN_POINT('Ctrl Pts',(-8.28236940693681,-38.2742356128,-5.99594511180924));
#62335=CARTESIAN_POINT('Ctrl Pts',(-8.35550578536951,-38.2742356128,-5.92357211331106));
#62336=CARTESIAN_POINT('Ctrl Pts',(-8.4278174655938,-38.2742356128084,-5.85015814590171));
#62337=CARTESIAN_POINT('Ctrl Pts',(-8.49920181258907,-38.2742356127916,
-5.77567763240077));
#62338=CARTESIAN_POINT('Ctrl Pts',(-8.57629785140191,-38.2742356127735,
-5.69523769281501));
#62339=CARTESIAN_POINT('Ctrl Pts',(-8.65231208372804,-38.2742356128263,
-5.61355320700452));
#62340=CARTESIAN_POINT('Ctrl Pts',(-8.72705743520762,-38.2742356121211,
-5.53056955773554));
#62341=CARTESIAN_POINT('Ctrl Pts',(-8.75811629125898,-38.274235611828,-5.49608745060457));
#62342=CARTESIAN_POINT('Ctrl Pts',(-8.78895542105945,-38.2742356113856,
-5.46138081859757));
#62343=CARTESIAN_POINT('Ctrl Pts',(-8.81955894353799,-38.2742356106072,
-5.42644509309065));
#62344=CARTESIAN_POINT('Ctrl Pts',(-8.90083523945013,-38.2742356085398,
-5.33366340868826));
#62345=CARTESIAN_POINT('Ctrl Pts',(-8.98046977411646,-38.2742356029034,
-5.23924732892919));
#62346=CARTESIAN_POINT('Ctrl Pts',(-9.05817344688913,-38.2742355974438,
-5.14307642848394));
#62347=CARTESIAN_POINT('Ctrl Pts',(-9.14533591774263,-38.2742355913196,
-5.03519873097103));
#62348=CARTESIAN_POINT('Ctrl Pts',(-9.23006783067603,-38.2742355884836,
-4.92511093215123));
#62349=CARTESIAN_POINT('Ctrl Pts',(-9.31189953927549,-38.2742355969756,
-4.81264955992679));
#62350=CARTESIAN_POINT('Ctrl Pts',(-9.38468149790253,-38.2742356045285,
-4.71262526518252));
#62351=CARTESIAN_POINT('Ctrl Pts',(-9.45510686120649,-38.2742356077932,
-4.61074833045805));
#62352=CARTESIAN_POINT('Ctrl Pts',(-9.52280503538855,-38.2742356097278,
-4.5069508612583));
#62353=CARTESIAN_POINT('Ctrl Pts',(-9.58549262089299,-38.2742356115191,
-4.4108358211672));
#62354=CARTESIAN_POINT('Ctrl Pts',(-9.64584072223927,-38.2742356120949,
-4.31307350300637));
#62355=CARTESIAN_POINT('Ctrl Pts',(-9.70356017216965,-38.274235612415,-4.21364954117544));
#62356=CARTESIAN_POINT('Ctrl Pts',(-9.75795283707027,-38.2742356127166,
-4.11995609389752));
#62357=CARTESIAN_POINT('Ctrl Pts',(-9.81001048715776,-38.2742356127563,
-4.02478670142455));
#62358=CARTESIAN_POINT('Ctrl Pts',(-9.85950734173672,-38.2742356127813,
-3.92817163468304));
#62359=CARTESIAN_POINT('Ctrl Pts',(-9.90588532561234,-38.2742356128046,
-3.83764442753836));
#62360=CARTESIAN_POINT('Ctrl Pts',(-9.95001471143252,-38.2742356127998,
-3.74584789685752));
#62361=CARTESIAN_POINT('Ctrl Pts',(-9.99173117763725,-38.2742356128,-3.65284794031525));
#62362=CARTESIAN_POINT('Ctrl Pts',(-10.0066488616391,-38.2742356128,-3.61959143299102));
#62363=CARTESIAN_POINT('Ctrl Pts',(-10.0212582251145,-38.2742356128,-3.58618144349341));
#62364=CARTESIAN_POINT('Ctrl Pts',(-10.0355526046835,-38.2742356128,-3.552622411423));
#62365=CARTESIAN_POINT('Ctrl Pts',(-10.0741195067863,-38.2742356128,-3.46207857926293));
#62366=CARTESIAN_POINT('Ctrl Pts',(-10.1103924680514,-38.2742356128,-3.37044307950816));
#62367=CARTESIAN_POINT('Ctrl Pts',(-10.144251066512,-38.2742356128,-3.27786011867359));
#62368=CARTESIAN_POINT('Ctrl Pts',(-10.175727743706,-38.2742356128,-3.19179028399764));
#62369=CARTESIAN_POINT('Ctrl Pts',(-10.2051178215566,-38.2742356128,-3.10490182707557));
#62370=CARTESIAN_POINT('Ctrl Pts',(-10.2323555261849,-38.2742356128,-3.01735062523928));
#62371=CARTESIAN_POINT('Ctrl Pts',(-10.2344166734751,-38.2742356128,-3.01072540021072));
#62372=CARTESIAN_POINT('Ctrl Pts',(-10.2364655111735,-38.2742356128,-3.00409639946743));
#62373=CARTESIAN_POINT('Ctrl Pts',(-10.2385020185954,-38.2742356128,-2.99746370018176));
#62374=CARTESIAN_POINT('Ctrl Pts',(-10.2652522054426,-38.2742356128,-2.91034103945238));
#62375=CARTESIAN_POINT('Ctrl Pts',(-10.289883505425,-38.2742356128,-2.82254091265382));
#62376=CARTESIAN_POINT('Ctrl Pts',(-10.31239561938,-38.2742356128,-2.7342474625325));
#62377=CARTESIAN_POINT('Ctrl Pts',(-10.3357459688454,-38.2742356128,-2.64266641776911));
#62378=CARTESIAN_POINT('Ctrl Pts',(-10.3568166272029,-38.2742356128,-2.55055473011936));
#62379=CARTESIAN_POINT('Ctrl Pts',(-10.3756579174403,-38.2742356128,-2.45809496166693));
#62380=CARTESIAN_POINT('Ctrl Pts',(-10.3779672486567,-38.2742356128,-2.44676239224857));
#62381=CARTESIAN_POINT('Ctrl Pts',(-10.3802431458191,-38.2742356128,-2.43542456529753));
#62382=CARTESIAN_POINT('Ctrl Pts',(-10.3824857483227,-38.2742356128,-2.42408179326659));
#62383=CARTESIAN_POINT('Ctrl Pts',(-10.4015615745755,-38.2742356128,-2.3275989131542));
#62384=CARTESIAN_POINT('Ctrl Pts',(-10.4182263197844,-38.2742356132236,
-2.23074979392517));
#62385=CARTESIAN_POINT('Ctrl Pts',(-10.4325715436647,-38.2742356123768,
-2.13373877808311));
#62386=CARTESIAN_POINT('Ctrl Pts',(-10.4384491467123,-38.2742356120298,
-2.09399089773411));
#62387=CARTESIAN_POINT('Ctrl Pts',(-10.4439379332837,-38.2742356114086,
-2.05421557115579));
#62388=CARTESIAN_POINT('Ctrl Pts',(-10.4490464009529,-38.2742356094761,
-2.01442572807813));
#62389=CARTESIAN_POINT('Ctrl Pts',(-10.4624519394082,-38.2742356044048,
-1.91001001948507));
#62390=CARTESIAN_POINT('Ctrl Pts',(-10.4732528313444,-38.2742355890201,
-1.80547263371963));
#62391=CARTESIAN_POINT('Ctrl Pts',(-10.4816751574859,-38.2742355691515,
-1.70099454498701));
#62392=CARTESIAN_POINT('Ctrl Pts',(-10.4842956528958,-38.2742355629696,
-1.66848756919981));
#62393=CARTESIAN_POINT('Ctrl Pts',(-10.4866861639936,-38.2742355566081,
-1.63598605690851));
#62394=CARTESIAN_POINT('Ctrl Pts',(-10.4888541645596,-38.2742355508364,
-1.6034947186437));
#62395=CARTESIAN_POINT('Ctrl Pts',(-10.4966767706617,-38.2742355300108,
-1.48625907536859));
#62396=CARTESIAN_POINT('Ctrl Pts',(-10.5016038327303,-38.2742355215113,
-1.36916012272759));
#62397=CARTESIAN_POINT('Ctrl Pts',(-10.5039692096414,-38.2742355269209,
-1.25235963069119));
#62398=CARTESIAN_POINT('Ctrl Pts',(-10.5063926047028,-38.2742355324631,
-1.13269424703444));
#62399=CARTESIAN_POINT('Ctrl Pts',(-10.5061290346563,-38.2742355509457,
-1.01334217949223));
#62400=CARTESIAN_POINT('Ctrl Pts',(-10.5035454403602,-38.2742355688688,
-0.894425537132182));
#62401=CARTESIAN_POINT('Ctrl Pts',(-10.5027611104684,-38.2742355743099,
-0.858324715351389));
#62402=CARTESIAN_POINT('Ctrl Pts',(-10.501762905098,-38.2742355796852,-0.822263666891019));
#62403=CARTESIAN_POINT('Ctrl Pts',(-10.5005608009666,-38.2742355846559,
-0.786244887924867));
#62404=CARTESIAN_POINT('Ctrl Pts',(-10.4969275725192,-38.2742355996795,
-0.677382062346776));
#62405=CARTESIAN_POINT('Ctrl Pts',(-10.4914181220826,-38.2742356052499,
-0.56887949337425));
#62406=CARTESIAN_POINT('Ctrl Pts',(-10.4842985290207,-38.274235608431,-0.46080570269692));
#62407=CARTESIAN_POINT('Ctrl Pts',(-10.4775343560835,-38.2742356114532,
-0.358127108041158));
#62408=CARTESIAN_POINT('Ctrl Pts',(-10.4693176834151,-38.2742356120957,
-0.255835196844215));
#62409=CARTESIAN_POINT('Ctrl Pts',(-10.4598437918636,-38.2742356124577,
-0.153959246988123));
#62410=CARTESIAN_POINT('Ctrl Pts',(-10.4508887624302,-38.2742356127998,
-0.0576627964168982));
#62411=CARTESIAN_POINT('Ctrl Pts',(-10.440810958642,-38.2742356127839,0.038262303108895));
#62412=CARTESIAN_POINT('Ctrl Pts',(-10.4297355589646,-38.2742356127946,
0.133813795867807));
#62413=CARTESIAN_POINT('Ctrl Pts',(-10.4186601592872,-38.2742356128053,
0.229365288626718));
#62414=CARTESIAN_POINT('Ctrl Pts',(-10.4065879660116,-38.2742356128,0.324543251269931));
#62415=CARTESIAN_POINT('Ctrl Pts',(-10.39359317545,-38.2742356128,0.419366129591117));
#62416=CARTESIAN_POINT('Ctrl Pts',(-10.3849069819887,-38.2742356128,0.482749210815547));
#62417=CARTESIAN_POINT('Ctrl Pts',(-10.3758063040751,-38.2742356128,0.545983232075174));
#62418=CARTESIAN_POINT('Ctrl Pts',(-10.3662947439406,-38.2742356128,0.60909237278372));
#62419=CARTESIAN_POINT('Ctrl Pts',(-10.3621130485487,-38.2742356128,0.636837894985739));
#62420=CARTESIAN_POINT('Ctrl Pts',(-10.3578515477501,-38.2742356128,0.664560643170705));
#62421=CARTESIAN_POINT('Ctrl Pts',(-10.3535102065,-38.2742356128,0.692259352582));
#62422=CARTESIAN_POINT('',(-9.72829242121,-38.2742356128,2.64854983337));
#62423=CARTESIAN_POINT('Ctrl Pts',(-10.3535102065,-38.2742356128,0.692259352582));
#62424=CARTESIAN_POINT('Ctrl Pts',(-10.348101240468,-38.2742356128,0.726769549321815));
#62425=CARTESIAN_POINT('Ctrl Pts',(-10.3426100454796,-38.2742356128,0.761029055591791));
#62426=CARTESIAN_POINT('Ctrl Pts',(-10.3370342145885,-38.2742356128,0.795218909178925));
#62427=CARTESIAN_POINT('Ctrl Pts',(-10.3312466866877,-38.2742356128,0.830706845492452));
#62428=CARTESIAN_POINT('Ctrl Pts',(-10.3253677818713,-38.2742356128,0.866119791080294));
#62429=CARTESIAN_POINT('Ctrl Pts',(-10.3193700787744,-38.2742356128,0.901609037191189));
#62430=CARTESIAN_POINT('Ctrl Pts',(-10.3132171268777,-38.2742356128,0.93801691211283));
#62431=CARTESIAN_POINT('Ctrl Pts',(-10.306938841305,-38.2742356128,0.974505008243299));
#62432=CARTESIAN_POINT('Ctrl Pts',(-10.3004839950347,-38.2742356128,1.01118418143873));
#62433=CARTESIAN_POINT('Ctrl Pts',(-10.2938473921693,-38.2742356128,1.04889617266743));
#62434=CARTESIAN_POINT('Ctrl Pts',(-10.2870237702254,-38.2742356128,1.08681005209566));
#62435=CARTESIAN_POINT('Ctrl Pts',(-10.2799401349208,-38.2742356128,1.12499289079426));
#62436=CARTESIAN_POINT('Ctrl Pts',(-10.2726428438253,-38.2742356128,1.16432739586815));
#62437=CARTESIAN_POINT('Ctrl Pts',(-10.2650691490111,-38.2742356128,1.20394719453697));
#62438=CARTESIAN_POINT('Ctrl Pts',(-10.2571276523262,-38.2742356128,1.24387150137696));
#62439=CARTESIAN_POINT('Ctrl Pts',(-10.2488260848449,-38.2742356128,1.28560599306385));
#62440=CARTESIAN_POINT('Ctrl Pts',(-10.2401219944262,-38.2742356128,1.32767315514082));
#62441=CARTESIAN_POINT('Ctrl Pts',(-10.2309068988015,-38.2742356128,1.37003813026781));
#62442=CARTESIAN_POINT('Ctrl Pts',(-10.2214777127999,-38.2742356128,1.41338735274933));
#62443=CARTESIAN_POINT('Ctrl Pts',(-10.211512734,-38.2742356128,1.45704802894355));
#62444=CARTESIAN_POINT('Ctrl Pts',(-10.2009022991903,-38.2742356128,1.50092829815079));
#62445=CARTESIAN_POINT('Ctrl Pts',(-10.1900848893554,-38.2742356128,1.54566452849331));
#62446=CARTESIAN_POINT('Ctrl Pts',(-10.1785957116405,-38.2742356128,1.59062853587755));
#62447=CARTESIAN_POINT('Ctrl Pts',(-10.166337985387,-38.2742356128,1.63567333892064));
#62448=CARTESIAN_POINT('Ctrl Pts',(-10.1651785470143,-38.2742356128,1.63993405351455));
#62449=CARTESIAN_POINT('Ctrl Pts',(-10.1640122525023,-38.2742356128,1.64419545815897));
#62450=CARTESIAN_POINT('Ctrl Pts',(-10.1628390332839,-38.2742356128,1.64845740848264));
#62451=CARTESIAN_POINT('Ctrl Pts',(-10.1452994394432,-38.2742356128,1.71217344421608));
#62452=CARTESIAN_POINT('Ctrl Pts',(-10.1262142672278,-38.2742356128,1.77600560337412));
#62453=CARTESIAN_POINT('Ctrl Pts',(-10.1054102946297,-38.2742356128,1.83964368181909));
#62454=CARTESIAN_POINT('Ctrl Pts',(-10.0886973273238,-38.2742356128,1.89076762554912));
#62455=CARTESIAN_POINT('Ctrl Pts',(-10.0708718635335,-38.2742356128,1.94176903797927));
#62456=CARTESIAN_POINT('Ctrl Pts',(-10.0518653199246,-38.2742356128,1.99250278927512));
#62457=CARTESIAN_POINT('Ctrl Pts',(-10.0354055571795,-38.2742356128,2.03643847409421));
#62458=CARTESIAN_POINT('Ctrl Pts',(-10.0180592615806,-38.2742356128,2.08017418180857));
#62459=CARTESIAN_POINT('Ctrl Pts',(-9.99982048572652,-38.2742356128,2.1236102911859));
#62460=CARTESIAN_POINT('Ctrl Pts',(-9.98302404946877,-38.2742356128,2.16361143206724));
#62461=CARTESIAN_POINT('Ctrl Pts',(-9.96547026680263,-38.2742356128,2.20335885372652));
#62462=CARTESIAN_POINT('Ctrl Pts',(-9.94719756114367,-38.2742356128,2.24276275517514));
#62463=CARTESIAN_POINT('Ctrl Pts',(-9.93038362357603,-38.2742356128,2.27902091810099));
#62464=CARTESIAN_POINT('Ctrl Pts',(-9.91296086855031,-38.2742356128,2.31498837465569));
#62465=CARTESIAN_POINT('Ctrl Pts',(-9.89500060023452,-38.2742356128,2.35058121284723));
#62466=CARTESIAN_POINT('Ctrl Pts',(-9.87764982370093,-38.2742356128,2.38496618810477));
#62467=CARTESIAN_POINT('Ctrl Pts',(-9.85979710564341,-38.2742356128,2.41900172326089));
#62468=CARTESIAN_POINT('Ctrl Pts',(-9.84155018037255,-38.2742356128,2.45259607912348));
#62469=CARTESIAN_POINT('Ctrl Pts',(-9.82324565167511,-38.2742356128,2.48629648847082));
#62470=CARTESIAN_POINT('Ctrl Pts',(-9.80454387289279,-38.2742356128,2.51955320597992));
#62471=CARTESIAN_POINT('Ctrl Pts',(-9.78560470964861,-38.2742356128,2.55225359104964));
#62472=CARTESIAN_POINT('Ctrl Pts',(-9.76789593607952,-38.2742356128,2.58282958362946));
#62473=CARTESIAN_POINT('Ctrl Pts',(-9.74997974302908,-38.2742356128,2.61291917292839));
#62474=CARTESIAN_POINT('Ctrl Pts',(-9.73203341524801,-38.2742356128,2.64241129302391));
#62475=CARTESIAN_POINT('Ctrl Pts',(-9.73078652051974,-38.2742356128,2.64446037902754));
#62476=CARTESIAN_POINT('Ctrl Pts',(-9.7295394997446,-38.2742356128,2.6465065727843));
#62477=CARTESIAN_POINT('Ctrl Pts',(-9.72829242121,-38.2742356128,2.64854983337));
#62478=CARTESIAN_POINT('',(-6.27496226640491,-38.2742356128,2.72284437887685));
#62479=CARTESIAN_POINT('Ctrl Pts',(-9.72829242121,-38.2742356128,2.64854983337));
#62480=CARTESIAN_POINT('Ctrl Pts',(-9.72206121244163,-38.2742356128,2.65875928126896));
#62481=CARTESIAN_POINT('Ctrl Pts',(-9.71578443101656,-38.2742356128,2.66896737401849));
#62482=CARTESIAN_POINT('Ctrl Pts',(-9.70945997971752,-38.2742356128,2.67917591849475));
#62483=CARTESIAN_POINT('Ctrl Pts',(-9.68961023804503,-38.2742356128,2.71121616374684));
#62484=CARTESIAN_POINT('Ctrl Pts',(-9.66928954578558,-38.2742356128159,
2.74326894858221));
#62485=CARTESIAN_POINT('Ctrl Pts',(-9.64842622432582,-38.2742356127842,
2.77533913689464));
#62486=CARTESIAN_POINT('Ctrl Pts',(-9.62681851214317,-38.2742356127513,
2.80855357017819));
#62487=CARTESIAN_POINT('Ctrl Pts',(-9.60462804880873,-38.2742356128199,
2.84178667887765));
#62488=CARTESIAN_POINT('Ctrl Pts',(-9.58176124412416,-38.2742356116715,
2.87499009644905));
#62489=CARTESIAN_POINT('Ctrl Pts',(-9.57746571331455,-38.2742356114558,
2.88122736068993));
#62490=CARTESIAN_POINT('Ctrl Pts',(-9.57314629616008,-38.274235611189,2.88746343032177));
#62491=CARTESIAN_POINT('Ctrl Pts',(-9.56880235347363,-38.2742356108485,
2.89369778504064));
#62492=CARTESIAN_POINT('Ctrl Pts',(-9.55457338499666,-38.2742356097332,
2.91411896533052));
#62493=CARTESIAN_POINT('Ctrl Pts',(-9.54008537245569,-38.2742356075311,
2.93451375044048));
#62494=CARTESIAN_POINT('Ctrl Pts',(-9.52529795253179,-38.274235603801,2.95489149144129));
#62495=CARTESIAN_POINT('Ctrl Pts',(-9.51051053260789,-38.2742356000709,
2.97526923244211));
#62496=CARTESIAN_POINT('Ctrl Pts',(-9.49539922664665,-38.2742355942278,
2.99565922465192));
#62497=CARTESIAN_POINT('Ctrl Pts',(-9.47992884555872,-38.2742355857358,
3.01604818304434));
#62498=CARTESIAN_POINT('Ctrl Pts',(-9.45461973979981,-38.2742355718433,
3.04940394211287));
#62499=CARTESIAN_POINT('Ctrl Pts',(-9.42835325782335,-38.274235553646,3.08276228151732));
#62500=CARTESIAN_POINT('Ctrl Pts',(-9.40112223778464,-38.2742355507865,
3.11587315896628));
#62501=CARTESIAN_POINT('Ctrl Pts',(-9.39506355579132,-38.2742355501503,
3.12324006173738));
#62502=CARTESIAN_POINT('Ctrl Pts',(-9.38895728119517,-38.2742355502767,
3.1305945808947));
#62503=CARTESIAN_POINT('Ctrl Pts',(-9.38280362499654,-38.2742355512933,
3.13793375497978));
#62504=CARTESIAN_POINT('Ctrl Pts',(-9.36533624499038,-38.2742355541788,
3.15876627121689));
#62505=CARTESIAN_POINT('Ctrl Pts',(-9.34748426667175,-38.2742355624319,
3.17947444717405));
#62506=CARTESIAN_POINT('Ctrl Pts',(-9.32922579032951,-38.2742355701077,
3.20000463237014));
#62507=CARTESIAN_POINT('Ctrl Pts',(-9.31096731398727,-38.2742355777835,
3.22053481756623));
#62508=CARTESIAN_POINT('Ctrl Pts',(-9.29231098634183,-38.2742355844588,
3.24087680479964));
#62509=CARTESIAN_POINT('Ctrl Pts',(-9.27317694561511,-38.2742355906155,
3.26105029981677));
#62510=CARTESIAN_POINT('Ctrl Pts',(-9.24445970593352,-38.2742355998558,
3.29132759983388));
#62511=CARTESIAN_POINT('Ctrl Pts',(-9.2146430488724,-38.2742356060047,3.32123956762131));
#62512=CARTESIAN_POINT('Ctrl Pts',(-9.1837237029298,-38.2742356090617,3.35053363451095));
#62513=CARTESIAN_POINT('Ctrl Pts',(-9.17344190202117,-38.2742356100783,
3.36027497134655));
#62514=CARTESIAN_POINT('Ctrl Pts',(-9.16303855804864,-38.2742356107937,
3.36994782914819));
#62515=CARTESIAN_POINT('Ctrl Pts',(-9.15251479486197,-38.2742356113,3.37954254011418));
#62516=CARTESIAN_POINT('Ctrl Pts',(-9.12005297789161,-38.2742356128614,
3.40913858344363));
#62517=CARTESIAN_POINT('Ctrl Pts',(-9.08643042979346,-38.2742356127779,
3.43800495025951));
#62518=CARTESIAN_POINT('Ctrl Pts',(-9.05165103904656,-38.274235612796,3.46590721443792));
#62519=CARTESIAN_POINT('Ctrl Pts',(-9.04124376010983,-38.2742356128014,
3.47425660297047));
#62520=CARTESIAN_POINT('Ctrl Pts',(-9.03073321972762,-38.2742356128,3.48251953511692));
#62521=CARTESIAN_POINT('Ctrl Pts',(-9.02012039388568,-38.2742356128,3.49068942360137));
#62522=CARTESIAN_POINT('Ctrl Pts',(-8.98898741571359,-38.2742356128,3.51465598666788));
#62523=CARTESIAN_POINT('Ctrl Pts',(-8.95695978201797,-38.2742356127997,
3.53783475496327));
#62524=CARTESIAN_POINT('Ctrl Pts',(-8.92403276743319,-38.2742356127993,
3.56007714970093));
#62525=CARTESIAN_POINT('Ctrl Pts',(-8.90822535481241,-38.2742356127992,
3.57075515120596));
#62526=CARTESIAN_POINT('Ctrl Pts',(-8.89221146739688,-38.2742356127992,
3.58121732420375));
#62527=CARTESIAN_POINT('Ctrl Pts',(-8.87599478577521,-38.2742356127994,
3.59144734775174));
#62528=CARTESIAN_POINT('Ctrl Pts',(-8.838986370624,-38.2742356128,3.61479349015639));
#62529=CARTESIAN_POINT('Ctrl Pts',(-8.80091222203195,-38.2742356128,3.63693279720875));
#62530=CARTESIAN_POINT('Ctrl Pts',(-8.76183764917323,-38.2742356128,3.65768687538109));
#62531=CARTESIAN_POINT('Ctrl Pts',(-8.72811628805191,-38.2742356128,3.67559764736368));
#62532=CARTESIAN_POINT('Ctrl Pts',(-8.69365111458049,-38.2742356128,3.69247656469757));
#62533=CARTESIAN_POINT('Ctrl Pts',(-8.6585144938953,-38.2742356128,3.70821531441722));
#62534=CARTESIAN_POINT('Ctrl Pts',(-8.62258077045391,-38.2742356128,3.72431111044742));
#62535=CARTESIAN_POINT('Ctrl Pts',(-8.58593577278161,-38.2742356128,3.73921800415691));
#62536=CARTESIAN_POINT('Ctrl Pts',(-8.54868983724074,-38.2742356128,3.75282640854491));
#62537=CARTESIAN_POINT('Ctrl Pts',(-8.52053919883706,-38.2742356128,3.76311169915756));
#62538=CARTESIAN_POINT('Ctrl Pts',(-8.49203815841643,-38.2742356128,3.77265815994509));
#62539=CARTESIAN_POINT('Ctrl Pts',(-8.46324819816481,-38.2742356128,3.78142244205252));
#62540=CARTESIAN_POINT('Ctrl Pts',(-8.4190268755565,-38.2742356128,3.79488436221898));
#62541=CARTESIAN_POINT('Ctrl Pts',(-8.37413308186376,-38.2742356128,3.80649598015092));
#62542=CARTESIAN_POINT('Ctrl Pts',(-8.32878118257724,-38.2742356128,3.81614800469356));
#62543=CARTESIAN_POINT('Ctrl Pts',(-8.28437937400409,-38.2742356128,3.82559782604234));
#62544=CARTESIAN_POINT('Ctrl Pts',(-8.23953875934846,-38.2742356128,3.83316896757169));
#62545=CARTESIAN_POINT('Ctrl Pts',(-8.1944704803585,-38.2742356128,3.8388044770508));
#62546=CARTESIAN_POINT('Ctrl Pts',(-8.150885627809,-38.2742356128,3.84425449323055));
#62547=CARTESIAN_POINT('Ctrl Pts',(-8.10708856365568,-38.2742356128,3.84789392309733));
#62548=CARTESIAN_POINT('Ctrl Pts',(-8.06326914099037,-38.2742356128,3.84971947920494));
#62549=CARTESIAN_POINT('Ctrl Pts',(-8.02135496316993,-38.2742356128,3.85146566111837));
#62550=CARTESIAN_POINT('Ctrl Pts',(-7.97942083965261,-38.2742356128,3.85155218090322));
#62551=CARTESIAN_POINT('Ctrl Pts',(-7.93762323916678,-38.2742356128,3.85002349382485));
#62552=CARTESIAN_POINT('Ctrl Pts',(-7.93004509331808,-38.2742356128,3.84974633404769));
#62553=CARTESIAN_POINT('Ctrl Pts',(-7.92247139718219,-38.2742356128,3.84941621215186));
#62554=CARTESIAN_POINT('Ctrl Pts',(-7.91490302783018,-38.2742356128,3.8490335730693));
#62555=CARTESIAN_POINT('Ctrl Pts',(-7.86845145763927,-38.2742356128,3.84668509014325));
#62556=CARTESIAN_POINT('Ctrl Pts',(-7.82219973451753,-38.2742356127606,
3.84234260710909));
#62557=CARTESIAN_POINT('Ctrl Pts',(-7.77633328742756,-38.2742356120254,
3.83608056160565));
#62558=CARTESIAN_POINT('Ctrl Pts',(-7.73831945958442,-38.274235611416,3.83089061699872));
#62559=CARTESIAN_POINT('Ctrl Pts',(-7.70056988557531,-38.274235610423,3.82438341370477));
#62560=CARTESIAN_POINT('Ctrl Pts',(-7.66317673260836,-38.2742356104353,
3.81662470151561));
#62561=CARTESIAN_POINT('Ctrl Pts',(-7.62192562203549,-38.2742356104488,
3.80806550099296));
#62562=CARTESIAN_POINT('Ctrl Pts',(-7.58110415372514,-38.2742356113252,
3.7979804666135));
#62563=CARTESIAN_POINT('Ctrl Pts',(-7.54080563372603,-38.2742356118068,
3.78645483313038));
#62564=CARTESIAN_POINT('Ctrl Pts',(-7.50050711372516,-38.2742356122885,
3.77492919964675));
#62565=CARTESIAN_POINT('Ctrl Pts',(-7.4607274036797,-38.2742356123951,3.76195892946109));
#62566=CARTESIAN_POINT('Ctrl Pts',(-7.4215996682472,-38.2742356124429,3.74767352673602));
#62567=CARTESIAN_POINT('Ctrl Pts',(-7.37576953416442,-38.2742356124989,
3.73094110112845));
#62568=CARTESIAN_POINT('Ctrl Pts',(-7.33080966098452,-38.2742356125197,
3.71239779074037));
#62569=CARTESIAN_POINT('Ctrl Pts',(-7.28688698368685,-38.274235612542,3.69227097596761));
#62570=CARTESIAN_POINT('Ctrl Pts',(-7.27485803495137,-38.2742356125482,
3.68675891618425));
#62571=CARTESIAN_POINT('Ctrl Pts',(-7.26290659591565,-38.2742356125543,
3.68112819714996));
#62572=CARTESIAN_POINT('Ctrl Pts',(-7.25103543965387,-38.2742356125609,
3.67538366592419));
#62573=CARTESIAN_POINT('Ctrl Pts',(-7.22342437675913,-38.2742356125763,
3.6620224895166));
#62574=CARTESIAN_POINT('Ctrl Pts',(-7.1962409699365,-38.27423561257,3.64804144895993));
#62575=CARTESIAN_POINT('Ctrl Pts',(-7.16951458768156,-38.2742356125657,
3.6335010353345));
#62576=CARTESIAN_POINT('Ctrl Pts',(-7.14278820542818,-38.2742356125615,
3.61896062170992));
#62577=CARTESIAN_POINT('Ctrl Pts',(-7.11650711974314,-38.2742356125844,
3.60385590787456));
#62578=CARTESIAN_POINT('Ctrl Pts',(-7.09066450610827,-38.2742356125935,
3.58822340182743));
#62579=CARTESIAN_POINT('Ctrl Pts',(-7.05214811130959,-38.274235612607,3.56492437398485));
#62580=CARTESIAN_POINT('Ctrl Pts',(-7.01458513687742,-38.2742356126672,
3.54044242465216));
#62581=CARTESIAN_POINT('Ctrl Pts',(-6.97799376259113,-38.2742356127132,
3.51491020294578));
#62582=CARTESIAN_POINT('Ctrl Pts',(-6.94358319795952,-38.2742356127564,
3.49089967635714));
#62583=CARTESIAN_POINT('Ctrl Pts',(-6.91003167756674,-38.2742356127845,
3.46596081997936));
#62584=CARTESIAN_POINT('Ctrl Pts',(-6.87732102706461,-38.2742356127938,
3.44017356082324));
#62585=CARTESIAN_POINT('Ctrl Pts',(-6.85147274014318,-38.2742356128012,
3.41979620777913));
#62586=CARTESIAN_POINT('Ctrl Pts',(-6.82614890728275,-38.2742356128,3.39888862739908));
#62587=CARTESIAN_POINT('Ctrl Pts',(-6.80132545127044,-38.2742356128,3.37747264929914));
#62588=CARTESIAN_POINT('Ctrl Pts',(-6.76339210431094,-38.2742356128,3.34474635496934));
#62589=CARTESIAN_POINT('Ctrl Pts',(-6.72665003782783,-38.2742356128499,
3.31084645522773));
#62590=CARTESIAN_POINT('Ctrl Pts',(-6.69110550144799,-38.2742356122268,
3.27587871692887));
#62591=CARTESIAN_POINT('Ctrl Pts',(-6.65332467546997,-38.2742356115645,
3.23871097836573));
#62592=CARTESIAN_POINT('Ctrl Pts',(-6.61689595956591,-38.2742356099512,
3.20033652698392));
#62593=CARTESIAN_POINT('Ctrl Pts',(-6.58182417042585,-38.2742356089708,
3.16082406650467));
#62594=CARTESIAN_POINT('Ctrl Pts',(-6.57342708240585,-38.274235608736,3.15136376759588));
#62595=CARTESIAN_POINT('Ctrl Pts',(-6.56510780276211,-38.2742356085496,
3.14183799650869));
#62596=CARTESIAN_POINT('Ctrl Pts',(-6.55686646545738,-38.2742356084435,
3.13224727289733));
#62597=CARTESIAN_POINT('Ctrl Pts',(-6.51731755512019,-38.2742356079345,
3.08622286518904));
#62598=CARTESIAN_POINT('Ctrl Pts',(-6.4795690142431,-38.2742356094994,3.03871550253006));
#62599=CARTESIAN_POINT('Ctrl Pts',(-6.44370529454587,-38.2742356107499,
2.98978551465853));
#62600=CARTESIAN_POINT('Ctrl Pts',(-6.41151588994877,-38.2742356118723,
2.94586850912135));
#62601=CARTESIAN_POINT('Ctrl Pts',(-6.38084419077031,-38.2742356125538,
2.90080380260923));
#62602=CARTESIAN_POINT('Ctrl Pts',(-6.35177864059283,-38.2742356127166,
2.8546119171942));
#62603=CARTESIAN_POINT('Ctrl Pts',(-6.32630607497036,-38.2742356128592,
2.81413011570496));
#62604=CARTESIAN_POINT('Ctrl Pts',(-6.30206526745315,-38.2742356128,2.77277584410025));
#62605=CARTESIAN_POINT('Ctrl Pts',(-6.27913862688043,-38.2742356128,2.73056930062515));
#62606=CARTESIAN_POINT('Ctrl Pts',(-6.27774176197317,-38.2742356128,2.72799775774035));
#62607=CARTESIAN_POINT('Ctrl Pts',(-6.27634984587968,-38.2742356128,2.72542318548171));
#62608=CARTESIAN_POINT('Ctrl Pts',(-6.27496226376,-38.2742356128,2.7228443803));
#62609=CARTESIAN_POINT('',(-2.29653415164,-38.2742356128,-2.09683582826));
#62610=CARTESIAN_POINT('Ctrl Pts',(-6.27496226971104,-38.2742356128,2.72284437709791));
#62611=CARTESIAN_POINT('Ctrl Pts',(-6.25343867541546,-38.2742356128,2.68284304096698));
#62612=CARTESIAN_POINT('Ctrl Pts',(-6.23329489033184,-38.2742356128021,
2.64244474672542));
#62613=CARTESIAN_POINT('Ctrl Pts',(-6.2143366952227,-38.2742356127979,2.60182941082557));
#62614=CARTESIAN_POINT('Ctrl Pts',(-6.19786423880922,-38.2742356127943,
2.56653942955479));
#62615=CARTESIAN_POINT('Ctrl Pts',(-6.18228642632628,-38.2742356127937,
2.53108405257986));
#62616=CARTESIAN_POINT('Ctrl Pts',(-6.16747377524522,-38.2742356127121,
2.4955497011575));
#62617=CARTESIAN_POINT('Ctrl Pts',(-6.14601564749822,-38.2742356125939,
2.44407338891229));
#62618=CARTESIAN_POINT('Ctrl Pts',(-6.12614048873929,-38.2742356124173,
2.39239502058356));
#62619=CARTESIAN_POINT('Ctrl Pts',(-6.10746783960564,-38.2742356124274,
2.3407042372701));
#62620=CARTESIAN_POINT('Ctrl Pts',(-6.0984087265777,-38.2742356124324,2.31562623975684));
#62621=CARTESIAN_POINT('Ctrl Pts',(-6.08963297438635,-38.2742356124787,
2.29054439503083));
#62622=CARTESIAN_POINT('Ctrl Pts',(-6.08109996571743,-38.2742356125507,
2.26547728984694));
#62623=CARTESIAN_POINT('Ctrl Pts',(-6.06532733137766,-38.2742356126837,
2.21914260306032));
#62624=CARTESIAN_POINT('Ctrl Pts',(-6.05038236765882,-38.2742356127776,
2.17285465240021));
#62625=CARTESIAN_POINT('Ctrl Pts',(-6.03602763222168,-38.2742356127936,
2.12669144192736));
#62626=CARTESIAN_POINT('Ctrl Pts',(-6.03255557415966,-38.2742356127975,
2.11552569472197));
#62627=CARTESIAN_POINT('Ctrl Pts',(-6.02911825580295,-38.2742356127989,
2.1043673476744));
#62628=CARTESIAN_POINT('Ctrl Pts',(-6.02571273819095,-38.2742356127995,
2.09321776498803));
#62629=CARTESIAN_POINT('Ctrl Pts',(-6.01988428400387,-38.2742356128005,
2.07413554627808));
#62630=CARTESIAN_POINT('Ctrl Pts',(-6.0141467501015,-38.2742356128,2.05507181057947));
#62631=CARTESIAN_POINT('Ctrl Pts',(-6.00849013333293,-38.2742356128,2.03604840855248));
#62632=CARTESIAN_POINT('Ctrl Pts',(-6.00270430180311,-38.2742356128,2.01659045271859));
#62633=CARTESIAN_POINT('Ctrl Pts',(-5.99700616637023,-38.2742356128,1.99718554365947));
#62634=CARTESIAN_POINT('Ctrl Pts',(-5.9914048278946,-38.2742356128,1.97792452860784));
#62635=CARTESIAN_POINT('Ctrl Pts',(-5.98556329602797,-38.2742356128,1.95783757373137));
#62636=CARTESIAN_POINT('Ctrl Pts',(-5.97982692637279,-38.2742356128,1.93790670946469));
#62637=CARTESIAN_POINT('Ctrl Pts',(-5.97419138868625,-38.2742356128,1.91817685111571));
#62638=CARTESIAN_POINT('Ctrl Pts',(-5.96803366204245,-38.2742356128,1.8966188239688));
#62639=CARTESIAN_POINT('Ctrl Pts',(-5.96199623521128,-38.2742356128,1.87530052368112));
#62640=CARTESIAN_POINT('Ctrl Pts',(-5.95605774049402,-38.2742356128,1.85421720432329));
#62641=CARTESIAN_POINT('Ctrl Pts',(-5.9522628450401,-38.2742356128,1.8407442626783));
#62642=CARTESIAN_POINT('Ctrl Pts',(-5.94850803272726,-38.2742356128,1.82736599721998));
#62643=CARTESIAN_POINT('Ctrl Pts',(-5.94478517864091,-38.2742356128,1.81407063595496));
#62644=CARTESIAN_POINT('Ctrl Pts',(-5.93738839707275,-38.2742356128,1.78765464412012));
#62645=CARTESIAN_POINT('Ctrl Pts',(-5.93012019351236,-38.2742356128,1.76157544910232));
#62646=CARTESIAN_POINT('Ctrl Pts',(-5.92289628650845,-38.2742356128,1.73565584384684));
#62647=CARTESIAN_POINT('Ctrl Pts',(-5.914084877134,-38.2742356128,1.70404023021749));
#62648=CARTESIAN_POINT('Ctrl Pts',(-5.90533754480164,-38.2742356128,1.67265553896624));
#62649=CARTESIAN_POINT('Ctrl Pts',(-5.89649392943623,-38.2742356128,1.64113094127172));
#62650=CARTESIAN_POINT('Ctrl Pts',(-5.89117577007019,-38.2742356128,1.62217344170142));
#62651=CARTESIAN_POINT('Ctrl Pts',(-5.88582275743926,-38.2742356128,1.60316479414047));
#62652=CARTESIAN_POINT('Ctrl Pts',(-5.88040459967885,-38.2742356128,1.58403821721294));
#62653=CARTESIAN_POINT('Ctrl Pts',(-5.87474911442545,-38.2742356128,1.56407385320862));
#62654=CARTESIAN_POINT('Ctrl Pts',(-5.86902251787269,-38.2742356128,1.54398063176711));
#62655=CARTESIAN_POINT('Ctrl Pts',(-5.86320917856773,-38.2742356128,1.52374749789215));
#62656=CARTESIAN_POINT('Ctrl Pts',(-5.85808049136635,-38.2742356128,1.50589727286574));
#62657=CARTESIAN_POINT('Ctrl Pts',(-5.85288428367078,-38.2742356128,1.4879380970169));
#62658=CARTESIAN_POINT('Ctrl Pts',(-5.84761945870423,-38.2742356128,1.46989499107882));
#62659=CARTESIAN_POINT('Ctrl Pts',(-5.8421991165419,-38.2742356128,1.45131891144139));
#62660=CARTESIAN_POINT('Ctrl Pts',(-5.83670655669577,-38.2742356128,1.43265575185725));
#62661=CARTESIAN_POINT('Ctrl Pts',(-5.83115983090085,-38.2742356128,1.41399731968152));
#62662=CARTESIAN_POINT('Ctrl Pts',(-5.83086484275531,-38.2742356128,1.41300501962742));
#62663=CARTESIAN_POINT('Ctrl Pts',(-5.830569704989,-38.2742356128,1.4120127447957));
#62664=CARTESIAN_POINT('Ctrl Pts',(-5.83027442154199,-38.2742356128,1.41102051304804));
#62665=CARTESIAN_POINT('Ctrl Pts',(-5.82494465487051,-38.2742356127999,
1.39311106450725));
#62666=CARTESIAN_POINT('Ctrl Pts',(-5.81957326542789,-38.2742356128,1.37523596643992));
#62667=CARTESIAN_POINT('Ctrl Pts',(-5.81415451162564,-38.2742356128,1.35740490081377));
#62668=CARTESIAN_POINT('Ctrl Pts',(-5.81362807119891,-38.2742356128,1.35567258483487));
#62669=CARTESIAN_POINT('Ctrl Pts',(-5.81310119326957,-38.2742356128,1.35394072452064));
#62670=CARTESIAN_POINT('Ctrl Pts',(-5.81257387902922,-38.2742356128,1.3522093558744));
#62671=CARTESIAN_POINT('Ctrl Pts',(-5.80520753857709,-38.2742356128,1.32802292220685));
#62672=CARTESIAN_POINT('Ctrl Pts',(-5.79777116024211,-38.2742356128,1.30398347871627));
#62673=CARTESIAN_POINT('Ctrl Pts',(-5.79022912459579,-38.2742356128,1.28002336192701));
#62674=CARTESIAN_POINT('Ctrl Pts',(-5.78202497565214,-38.2742356128,1.25395979287694));
#62675=CARTESIAN_POINT('Ctrl Pts',(-5.77369596379631,-38.2742356128,1.22799072420539));
#62676=CARTESIAN_POINT('Ctrl Pts',(-5.7652157517049,-38.2742356128,1.20209112335984));
#62677=CARTESIAN_POINT('Ctrl Pts',(-5.75504575170402,-38.2742356128,1.17103070437704));
#62678=CARTESIAN_POINT('Ctrl Pts',(-5.74465852701919,-38.2742356128,1.14007133411449));
#62679=CARTESIAN_POINT('Ctrl Pts',(-5.73403313082186,-38.2742356128,1.10924352573199));
#62680=CARTESIAN_POINT('Ctrl Pts',(-5.72151165526241,-38.2742356128,1.07291456048266));
#62681=CARTESIAN_POINT('Ctrl Pts',(-5.70866115126366,-38.2742356128,1.03677487726414));
#62682=CARTESIAN_POINT('Ctrl Pts',(-5.69546311036074,-38.2742356128,1.00090701483098));
#62683=CARTESIAN_POINT('Ctrl Pts',(-5.68570249198199,-38.2742356128,0.974380917522556));
#62684=CARTESIAN_POINT('Ctrl Pts',(-5.67575238409884,-38.2742356128,0.948005045359147));
#62685=CARTESIAN_POINT('Ctrl Pts',(-5.66559884051821,-38.2742356128,0.92178185094905));
#62686=CARTESIAN_POINT('Ctrl Pts',(-5.66202304049715,-38.2742356128,0.912546759930898));
#62687=CARTESIAN_POINT('Ctrl Pts',(-5.65842190859526,-38.2742356128,0.90333018961899));
#62688=CARTESIAN_POINT('Ctrl Pts',(-5.65479443282628,-38.2742356128,0.89413063357453));
#62689=CARTESIAN_POINT('Ctrl Pts',(-5.63120997437853,-38.2742356128,0.834318642789297));
#62690=CARTESIAN_POINT('Ctrl Pts',(-5.60650655989423,-38.2742356128,0.775223123984615));
#62691=CARTESIAN_POINT('Ctrl Pts',(-5.58056333005086,-38.2742356128,0.716890523122717));
#62692=CARTESIAN_POINT('Ctrl Pts',(-5.55256032032622,-38.2742356128,0.653926566858942));
#62693=CARTESIAN_POINT('Ctrl Pts',(-5.52311298107293,-38.2742356128,0.591851719963286));
#62694=CARTESIAN_POINT('Ctrl Pts',(-5.49213034599839,-38.2742356128,0.530709651061986));
#62695=CARTESIAN_POINT('Ctrl Pts',(-5.45933890499242,-38.2742356128,0.465998029841364));
#62696=CARTESIAN_POINT('Ctrl Pts',(-5.42482839106383,-38.2742356128,0.402331539315345));
#62697=CARTESIAN_POINT('Ctrl Pts',(-5.38854948129966,-38.2742356128,0.339742119926858));
#62698=CARTESIAN_POINT('Ctrl Pts',(-5.34797421744951,-38.2742356128,0.269740506801641));
#62699=CARTESIAN_POINT('Ctrl Pts',(-5.30518791818639,-38.2742356128,0.201086868540641));
#62700=CARTESIAN_POINT('Ctrl Pts',(-5.2601797548669,-38.2742356128,0.13379375830936));
#62701=CARTESIAN_POINT('Ctrl Pts',(-5.24442214693411,-38.2742356128,0.110234066702396));
#62702=CARTESIAN_POINT('Ctrl Pts',(-5.22839258827465,-38.2742356128,0.0868408264598558));
#62703=CARTESIAN_POINT('Ctrl Pts',(-5.21209158864003,-38.2742356128,0.0636135438118852));
#62704=CARTESIAN_POINT('Ctrl Pts',(-5.16303895840601,-38.2742356128,-0.00628151370670113));
#62705=CARTESIAN_POINT('Ctrl Pts',(-5.11152067541813,-38.2742356128,-0.0746775353743387));
#62706=CARTESIAN_POINT('Ctrl Pts',(-5.05770039912222,-38.2742356128,-0.141553198717477));
#62707=CARTESIAN_POINT('Ctrl Pts',(-5.00070653692266,-38.2742356128,-0.212372276645049));
#62708=CARTESIAN_POINT('Ctrl Pts',(-4.94113150722171,-38.2742356128,-0.281486624304317));
#62709=CARTESIAN_POINT('Ctrl Pts',(-4.87920687688789,-38.2742356128,-0.348920019142021));
#62710=CARTESIAN_POINT('Ctrl Pts',(-4.81218558689648,-38.2742356128,-0.421903468314986));
#62711=CARTESIAN_POINT('Ctrl Pts',(-4.74241250105015,-38.2742356128,-0.492918183244864));
#62712=CARTESIAN_POINT('Ctrl Pts',(-4.67021747606694,-38.2742356128,-0.562046414701979));
#62713=CARTESIAN_POINT('Ctrl Pts',(-4.63784417473622,-38.2742356128,-0.593044521121934));
#62714=CARTESIAN_POINT('Ctrl Pts',(-4.60498324021259,-38.2742356128,-0.623664886468992));
#62715=CARTESIAN_POINT('Ctrl Pts',(-4.5716693681391,-38.2742356128,-0.653914580276434));
#62716=CARTESIAN_POINT('Ctrl Pts',(-4.48958434544408,-38.2742356128,-0.728449500661054));
#62717=CARTESIAN_POINT('Ctrl Pts',(-4.40477413851654,-38.2742356128,-0.800708714336258));
#62718=CARTESIAN_POINT('Ctrl Pts',(-4.31774788686279,-38.2742356128,-0.870862803916576));
#62719=CARTESIAN_POINT('Ctrl Pts',(-4.27180201100859,-38.2742356128,-0.907900950789164));
#62720=CARTESIAN_POINT('Ctrl Pts',(-4.22524096850355,-38.2742356128,-0.944351251618469));
#62721=CARTESIAN_POINT('Ctrl Pts',(-4.17813182275849,-38.2742356128,-0.980247599868581));
#62722=CARTESIAN_POINT('Ctrl Pts',(-4.09980474547713,-38.2742356128,-1.03993146802277));
#62723=CARTESIAN_POINT('Ctrl Pts',(-4.01995584057801,-38.2742356128,-1.09809026518485));
#62724=CARTESIAN_POINT('Ctrl Pts',(-3.93889540951161,-38.2742356128,-1.15486566991628));
#62725=CARTESIAN_POINT('Ctrl Pts',(-3.89820004443583,-38.2742356128,-1.1833690444046));
#62726=CARTESIAN_POINT('Ctrl Pts',(-3.8571990327442,-38.2742356128,-1.21152368000513));
#62727=CARTESIAN_POINT('Ctrl Pts',(-3.8159293073926,-38.2742356128,-1.23934650848657));
#62728=CARTESIAN_POINT('Ctrl Pts',(-3.77240858136084,-38.2742356128,-1.26868689506422));
#62729=CARTESIAN_POINT('Ctrl Pts',(-3.72858183608195,-38.2742356128,-1.29766321120108));
#62730=CARTESIAN_POINT('Ctrl Pts',(-3.68449058042176,-38.2742356128,-1.32629284236997));
#62731=CARTESIAN_POINT('Ctrl Pts',(-3.60314006363722,-38.2742356128,-1.37911590798846));
#62732=CARTESIAN_POINT('Ctrl Pts',(-3.52089527451447,-38.2742356128,-1.43075803920082));
#62733=CARTESIAN_POINT('Ctrl Pts',(-3.43801071125674,-38.2742356128,-1.48129673933209));
#62734=CARTESIAN_POINT('Ctrl Pts',(-3.3604874182667,-38.2742356128,-1.52856641541676));
#62735=CARTESIAN_POINT('Ctrl Pts',(-3.28240471810566,-38.2742356128,-1.57487116471378));
#62736=CARTESIAN_POINT('Ctrl Pts',(-3.20393382874924,-38.2742356128,-1.62024778862748));
#62737=CARTESIAN_POINT('Ctrl Pts',(-3.12983202014925,-38.2742356128,-1.66309794526191));
#62738=CARTESIAN_POINT('Ctrl Pts',(-3.05538418311467,-38.2742356128,-1.70512065770332));
#62739=CARTESIAN_POINT('Ctrl Pts',(-2.98069750636388,-38.2742356128,-1.74631839971243));
#62740=CARTESIAN_POINT('Ctrl Pts',(-2.95738588423248,-38.2742356128,-1.75917726873921));
#62741=CARTESIAN_POINT('Ctrl Pts',(-2.93405203055978,-38.2742356128,-1.77195479357069));
#62742=CARTESIAN_POINT('Ctrl Pts',(-2.91070243365683,-38.2742356128,-1.78464824943072));
#62743=CARTESIAN_POINT('Ctrl Pts',(-2.86043357653793,-38.2742356128,-1.81197572414581));
#62744=CARTESIAN_POINT('Ctrl Pts',(-2.81007886487402,-38.2742356128,-1.83892187073565));
#62745=CARTESIAN_POINT('Ctrl Pts',(-2.75958339447557,-38.2742356128,-1.86551280695808));
#62746=CARTESIAN_POINT('Ctrl Pts',(-2.72930698729957,-38.2742356128,-1.88145637587443));
#62747=CARTESIAN_POINT('Ctrl Pts',(-2.69897964236885,-38.2742356128,-1.89727208811875));
#62748=CARTESIAN_POINT('Ctrl Pts',(-2.66858803344439,-38.2742356128,-1.91296318395376));
#62749=CARTESIAN_POINT('Ctrl Pts',(-2.6077524293637,-38.2742356128,-1.94437242247689));
#62750=CARTESIAN_POINT('Ctrl Pts',(-2.54669259970672,-38.2742356128,-1.9752662642291));
#62751=CARTESIAN_POINT('Ctrl Pts',(-2.48550737802581,-38.2742356128,-2.00554502912596));
#62752=CARTESIAN_POINT('Ctrl Pts',(-2.4507304139965,-38.2742356128,-2.02275512477883));
#62753=CARTESIAN_POINT('Ctrl Pts',(-2.4159125560593,-38.2742356128,-2.03976628509963));
#62754=CARTESIAN_POINT('Ctrl Pts',(-2.38106878359342,-38.2742356128,-2.05655838691403));
#62755=CARTESIAN_POINT('Ctrl Pts',(-2.3546097942447,-38.2742356128,-2.06930964808947));
#62756=CARTESIAN_POINT('Ctrl Pts',(-2.32813281720675,-38.2742356128,-2.08193609605139));
#62757=CARTESIAN_POINT('Ctrl Pts',(-2.30161949261477,-38.2742356128,-2.09443938197145));
#62758=CARTESIAN_POINT('Ctrl Pts',(-2.29992454402612,-38.2742356128,-2.09523869428516));
#62759=CARTESIAN_POINT('Ctrl Pts',(-2.29822962710667,-38.2742356128,-2.09603741777667));
#62760=CARTESIAN_POINT('Ctrl Pts',(-2.29653415164,-38.2742356128,-2.09683582826));
#62761=CARTESIAN_POINT('',(-1.05996521274483,-38.2742356128,-2.50526954715394));
#62762=CARTESIAN_POINT('Origin',(-0.442664407162939,-38.2742356128,1.43778039829082));
#62763=CARTESIAN_POINT('',(-0.417273426023,-38.2742356128,-3.28965093269));
#62764=CARTESIAN_POINT('Ctrl Pts',(-1.05996499772,-38.2742356128,-2.50526959461));
#62765=CARTESIAN_POINT('Ctrl Pts',(-1.0545628851308,-38.2742356128,-2.50635300094287));
#62766=CARTESIAN_POINT('Ctrl Pts',(-1.04893587647229,-38.2742356128,-2.50754377045459));
#62767=CARTESIAN_POINT('Ctrl Pts',(-1.04355928227185,-38.2742356128,-2.50874100265385));
#62768=CARTESIAN_POINT('Ctrl Pts',(-1.03810376887435,-38.2742356128,-2.5099558081719));
#62769=CARTESIAN_POINT('Ctrl Pts',(-1.03266139142698,-38.2742356128,-2.51122815763621));
#62770=CARTESIAN_POINT('Ctrl Pts',(-1.02723368169931,-38.2742356128,-2.51255742238625));
#62771=CARTESIAN_POINT('Ctrl Pts',(-0.998495061676567,-38.2742356128,-2.51959560911282));
#62772=CARTESIAN_POINT('Ctrl Pts',(-0.970143039745548,-38.2742356128108,
-2.52823878716873));
#62773=CARTESIAN_POINT('Ctrl Pts',(-0.942373769726441,-38.2742356127073,
-2.53841013176227));
#62774=CARTESIAN_POINT('Ctrl Pts',(-0.909912208880344,-38.2742356125864,
-2.55030017140619));
#62775=CARTESIAN_POINT('Ctrl Pts',(-0.878246461049334,-38.274235612256,
-2.56427904455269));
#62776=CARTESIAN_POINT('Ctrl Pts',(-0.847615534382662,-38.2742356120111,
-2.58023943993716));
#62777=CARTESIAN_POINT('Ctrl Pts',(-0.835164165836895,-38.2742356119116,
-2.58672728691713));
#62778=CARTESIAN_POINT('Ctrl Pts',(-0.822883090372356,-38.2742356118354,
-2.59354265810511));
#62779=CARTESIAN_POINT('Ctrl Pts',(-0.810786145712179,-38.2742356118171,
-2.60067845985212));
#62780=CARTESIAN_POINT('Ctrl Pts',(-0.778112483915285,-38.2742356117674,
-2.61995215081137));
#62781=CARTESIAN_POINT('Ctrl Pts',(-0.746830967014757,-38.2742356121238,
-2.64153966888173));
#62782=CARTESIAN_POINT('Ctrl Pts',(-0.71722542326134,-38.2742356123874,
-2.66524179112785));
#62783=CARTESIAN_POINT('Ctrl Pts',(-0.691853613893979,-38.2742356126133,
-2.68555439650471));
#62784=CARTESIAN_POINT('Ctrl Pts',(-0.667710524559884,-38.2742356127472,
-2.70742011010636));
#62785=CARTESIAN_POINT('Ctrl Pts',(-0.644980774960419,-38.274235612782,
-2.73067823100576));
#62786=CARTESIAN_POINT('Ctrl Pts',(-0.63074658199222,-38.2742356128038,
-2.74524330923115));
#62787=CARTESIAN_POINT('Ctrl Pts',(-0.617066898747946,-38.2742356128,-2.76035374556724));
#62788=CARTESIAN_POINT('Ctrl Pts',(-0.603993341432776,-38.2742356128,-2.7759612906689));
#62789=CARTESIAN_POINT('Ctrl Pts',(-0.579481412026907,-38.2742356128,-2.80522425517872));
#62790=CARTESIAN_POINT('Ctrl Pts',(-0.557089172077376,-38.2742356128,-2.83624768270283));
#62791=CARTESIAN_POINT('Ctrl Pts',(-0.537022980088056,-38.2742356128,-2.86871379934565));
#62792=CARTESIAN_POINT('Ctrl Pts',(-0.516411183247313,-38.2742356128,-2.90206267793734));
#62793=CARTESIAN_POINT('Ctrl Pts',(-0.498254305254846,-38.2742356128,-2.9369329166477));
#62794=CARTESIAN_POINT('Ctrl Pts',(-0.482738377586076,-38.2742356128,-2.97294076116154));
#62795=CARTESIAN_POINT('Ctrl Pts',(-0.47739895586098,-38.2742356128,-2.98533196788636));
#62796=CARTESIAN_POINT('Ctrl Pts',(-0.472371914802775,-38.2742356128,-2.99785761789655));
#62797=CARTESIAN_POINT('Ctrl Pts',(-0.467663626133187,-38.2742356128,-3.01050133048556));
#62798=CARTESIAN_POINT('Ctrl Pts',(-0.453513865456522,-38.2742356128,-3.04849932078608));
#62799=CARTESIAN_POINT('Ctrl Pts',(-0.442243464789961,-38.2742356128,-3.08757329554101));
#62800=CARTESIAN_POINT('Ctrl Pts',(-0.433990885022559,-38.2742356128,-3.12728197170967));
#62801=CARTESIAN_POINT('Ctrl Pts',(-0.426017960141965,-38.2742356127999,
-3.16564504133441));
#62802=CARTESIAN_POINT('Ctrl Pts',(-0.42086197130703,-38.2742356127999,
-3.204599556636));
#62803=CARTESIAN_POINT('Ctrl Pts',(-0.418599488142137,-38.2742356128,-3.24374472071435));
#62804=CARTESIAN_POINT('Ctrl Pts',(-0.417956545491016,-38.2742356128,-3.25486882362997));
#62805=CARTESIAN_POINT('Ctrl Pts',(-0.417546953560373,-38.2742356128,-3.26600835246778));
#62806=CARTESIAN_POINT('Ctrl Pts',(-0.417371692423965,-38.2742356128,-3.27715422675297));
#62807=CARTESIAN_POINT('Ctrl Pts',(-0.417306202598934,-38.2742356128,-3.2813191053548));
#62808=CARTESIAN_POINT('Ctrl Pts',(-0.417273424670102,-38.2742356128,-3.28548503749));
#62809=CARTESIAN_POINT('Ctrl Pts',(-0.417273426023,-38.2742356128,-3.28965093269));
#62810=CARTESIAN_POINT('',(-0.417297207341341,-38.2742356124858,-7.95031781344913));
#62811=CARTESIAN_POINT('',(-0.417273426056,-38.2742356128,0.916320001688));
#62812=CARTESIAN_POINT('',(-2.08574231668,-38.2742356128,-9.3172814696));
#62813=CARTESIAN_POINT('Ctrl Pts',(-0.417320987633984,-38.2742356128,-7.9503177501852));
#62814=CARTESIAN_POINT('Ctrl Pts',(-0.417572749059598,-38.2742356128,-7.98992259023869));
#62815=CARTESIAN_POINT('Ctrl Pts',(-0.419478320445827,-38.2742356128,-8.02968070118645));
#62816=CARTESIAN_POINT('Ctrl Pts',(-0.423055995654528,-38.2742356128,-8.06934147447744));
#62817=CARTESIAN_POINT('Ctrl Pts',(-0.42677560847607,-38.2742356128,-8.11057571521752));
#62818=CARTESIAN_POINT('Ctrl Pts',(-0.432302579823145,-38.2742356128,-8.15170500580991));
#62819=CARTESIAN_POINT('Ctrl Pts',(-0.439630146125636,-38.2742356128,-8.19249683682004));
#62820=CARTESIAN_POINT('Ctrl Pts',(-0.447522256504563,-38.2742356128,-8.23643142841576));
#62821=CARTESIAN_POINT('Ctrl Pts',(-0.45750317150351,-38.2742356128,-8.27997470252336));
#62822=CARTESIAN_POINT('Ctrl Pts',(-0.469532954288344,-38.2742356128,-8.32288925071818));
#62823=CARTESIAN_POINT('Ctrl Pts',(-0.482341712347726,-38.2742356128,-8.36858268300095));
#62824=CARTESIAN_POINT('Ctrl Pts',(-0.497473211468047,-38.2742356128,-8.41356385330956));
#62825=CARTESIAN_POINT('Ctrl Pts',(-0.514844778617922,-38.2742356128,-8.45759880680696));
#62826=CARTESIAN_POINT('Ctrl Pts',(-0.533782263511972,-38.2742356128,-8.50560318427461));
#62827=CARTESIAN_POINT('Ctrl Pts',(-0.555381809168105,-38.2742356128,-8.55248392532889));
#62828=CARTESIAN_POINT('Ctrl Pts',(-0.579497316992987,-38.2742356128,-8.59798785499368));
#62829=CARTESIAN_POINT('Ctrl Pts',(-0.609099788346512,-38.2742356128,-8.65384522213503));
#62830=CARTESIAN_POINT('Ctrl Pts',(-0.642493917780337,-38.2742356128,-8.70762998352329));
#62831=CARTESIAN_POINT('Ctrl Pts',(-0.679347289484414,-38.2742356128,-8.75892505849224));
#62832=CARTESIAN_POINT('Ctrl Pts',(-0.712858980986859,-38.2742356128,-8.80556895153294));
#62833=CARTESIAN_POINT('Ctrl Pts',(-0.749229201825039,-38.2742356128,-8.85015749719262));
#62834=CARTESIAN_POINT('Ctrl Pts',(-0.788176879238902,-38.2742356128,-8.8923704480671));
#62835=CARTESIAN_POINT('Ctrl Pts',(-0.824990130602421,-38.2742356128,-8.93227002808121));
#62836=CARTESIAN_POINT('Ctrl Pts',(-0.864105064693452,-38.2742356128,-8.97004925769915));
#62837=CARTESIAN_POINT('Ctrl Pts',(-0.905273940415647,-38.2742356128,-9.00539581352769));
#62838=CARTESIAN_POINT('Ctrl Pts',(-0.956525180854692,-38.2742356128,-9.0493988327912));
#62839=CARTESIAN_POINT('Ctrl Pts',(-1.01096309064526,-38.2742356128,-9.08962219803601));
#62840=CARTESIAN_POINT('Ctrl Pts',(-1.06801175261871,-38.2742356128,-9.12571954250596));
#62841=CARTESIAN_POINT('Ctrl Pts',(-1.12236508635952,-38.2742356128,-9.16011142731555));
#62842=CARTESIAN_POINT('Ctrl Pts',(-1.17908764585001,-38.2742356128,-9.19075679716307));
#62843=CARTESIAN_POINT('Ctrl Pts',(-1.23764596567446,-38.2742356128,-9.21738500781742));
#62844=CARTESIAN_POINT('Ctrl Pts',(-1.29309164983784,-38.2742356128,-9.24259781040812));
#62845=CARTESIAN_POINT('Ctrl Pts',(-1.35018262233756,-38.2742356128,-9.26420845056948));
#62846=CARTESIAN_POINT('Ctrl Pts',(-1.40844166177688,-38.2742356128,-9.28202664749419));
#62847=CARTESIAN_POINT('Ctrl Pts',(-1.46299899906197,-38.2742356128,-9.29871269980107));
#62848=CARTESIAN_POINT('Ctrl Pts',(-1.51858030850855,-38.2742356128,-9.31207260921611));
#62849=CARTESIAN_POINT('Ctrl Pts',(-1.57477777606112,-38.2742356128,-9.32199254814538));
#62850=CARTESIAN_POINT('Ctrl Pts',(-1.62868478067783,-38.2742356128,-9.33150817610776));
#62851=CARTESIAN_POINT('Ctrl Pts',(-1.68315851183546,-38.2742356128,-9.33785820793617));
#62852=CARTESIAN_POINT('Ctrl Pts',(-1.73782801715715,-38.2742356128,-9.34098723621135));
#62853=CARTESIAN_POINT('Ctrl Pts',(-1.79089269674258,-38.2742356128,-9.34402441172372));
#62854=CARTESIAN_POINT('Ctrl Pts',(-1.84414165890464,-38.2742356128,-9.34402660305071));
#62855=CARTESIAN_POINT('Ctrl Pts',(-1.89722788544739,-38.2742356128,-9.34099112391457));
#62856=CARTESIAN_POINT('Ctrl Pts',(-1.94839107668105,-38.2742356128,-9.33806560425264));
#62857=CARTESIAN_POINT('Ctrl Pts',(-1.99940296981809,-38.2742356128,-9.33231833411543));
#62858=CARTESIAN_POINT('Ctrl Pts',(-2.04994776736356,-38.2742356128,-9.32379549157948));
#62859=CARTESIAN_POINT('Ctrl Pts',(-2.06190685559861,-38.2742356128,-9.32177895514348));
#62860=CARTESIAN_POINT('Ctrl Pts',(-2.07383977686135,-38.2742356128,-9.31960726587291));
#62861=CARTESIAN_POINT('Ctrl Pts',(-2.08574231668,-38.2742356128,-9.3172814696));
#62862=CARTESIAN_POINT('Ctrl Pts',(-2.08574231668,-38.2742356128,-9.3172814696));
#62863=CARTESIAN_POINT('Ctrl Pts',(-2.08729719662647,-38.2742356128,-9.31697764277153));
#62864=CARTESIAN_POINT('Ctrl Pts',(-2.08885006320223,-38.2742356128002,
-9.3166755848767));
#62865=CARTESIAN_POINT('Ctrl Pts',(-2.09040818399078,-38.2742356127997,
-9.31637399587293));
#62866=CARTESIAN_POINT('Ctrl Pts',(-2.09088805053492,-38.2742356127995,
-9.31628111316829));
#62867=CARTESIAN_POINT('Ctrl Pts',(-2.09136804121834,-38.2742356127993,
-9.31618834238779));
#62868=CARTESIAN_POINT('Ctrl Pts',(-2.09184736274659,-38.2742356127989,
-9.31609582751137));
#62869=CARTESIAN_POINT('Ctrl Pts',(-2.09373347566305,-38.2742356127973,
-9.31573178481124));
#62870=CARTESIAN_POINT('Ctrl Pts',(-2.0956458104322,-38.2742356127953,-9.31536531693948));
#62871=CARTESIAN_POINT('Ctrl Pts',(-2.0975785896359,-38.2742356127946,-9.31499710213531));
#62872=CARTESIAN_POINT('Ctrl Pts',(-2.10028622939785,-38.2742356127937,
-9.31448126823001));
#62873=CARTESIAN_POINT('Ctrl Pts',(-2.10302673644695,-38.2742356127952,
-9.31396332695846));
#62874=CARTESIAN_POINT('Ctrl Pts',(-2.10570065575222,-38.2742356127967,
-9.31346143484423));
#62875=CARTESIAN_POINT('Ctrl Pts',(-2.10750112540457,-38.2742356127978,
-9.31312348840036));
#62876=CARTESIAN_POINT('Ctrl Pts',(-2.10926918488457,-38.2742356127987,
-9.31279324863373));
#62877=CARTESIAN_POINT('Ctrl Pts',(-2.11100388243363,-38.2742356127993,
-9.31247098633571));
#62878=CARTESIAN_POINT('Ctrl Pts',(-2.11247433135277,-38.2742356127997,
-9.31219781465339));
#62879=CARTESIAN_POINT('Ctrl Pts',(-2.11392035045784,-38.2742356127999,
-9.31193046282621));
#62880=CARTESIAN_POINT('Ctrl Pts',(-2.11537824249551,-38.2742356128,-9.31166232294267));
#62881=CARTESIAN_POINT('Ctrl Pts',(-2.11634463787306,-38.2742356128,-9.31148458060147));
#62882=CARTESIAN_POINT('Ctrl Pts',(-2.11731696466449,-38.2742356128,-9.3113063607223));
#62883=CARTESIAN_POINT('Ctrl Pts',(-2.11831853867763,-38.2742356128,-9.31112338855063));
#62884=CARTESIAN_POINT('Ctrl Pts',(-2.11872298471233,-38.2742356128,-9.31104950247899));
#62885=CARTESIAN_POINT('Ctrl Pts',(-2.11912809869579,-38.2742356128,-9.31097559323517));
#62886=CARTESIAN_POINT('Ctrl Pts',(-2.11954020693,-38.2742356128,-9.31090050519));
#62887=CARTESIAN_POINT('',(-2.3929454134173E-5,-38.2742356128,10.9643459683816));
#62888=CARTESIAN_POINT('',(5.53988693785,-38.2742356128,5.6069786219));
#62889=CARTESIAN_POINT('Ctrl Pts',(2.41089864840838E-5,-38.2742356128,10.9643459827));
#62890=CARTESIAN_POINT('Ctrl Pts',(0.00400146984433971,-38.2742356128,10.9643456323764));
#62891=CARTESIAN_POINT('Ctrl Pts',(0.00791495370935219,-38.2742356128,10.9643411554458));
#62892=CARTESIAN_POINT('Ctrl Pts',(0.011860445155913,-38.2742356128,10.9643324386718));
#62893=CARTESIAN_POINT('Ctrl Pts',(0.165738700552314,-38.2742356128,10.9639924754519));
#62894=CARTESIAN_POINT('Ctrl Pts',(0.319616215076356,-38.2742356128,10.957256326624));
#62895=CARTESIAN_POINT('Ctrl Pts',(0.472948512224986,-38.2742356128,10.9441347145538));
#62896=CARTESIAN_POINT('Ctrl Pts',(0.630182100908691,-38.2742356128,10.9306792443529));
#62897=CARTESIAN_POINT('Ctrl Pts',(0.786842159219016,-38.2742356128,10.9105091862989));
#62898=CARTESIAN_POINT('Ctrl Pts',(0.942351550939209,-38.2742356128,10.8836912177522));
#62899=CARTESIAN_POINT('Ctrl Pts',(1.09720894779707,-38.2742356128,10.8569856872874));
#62900=CARTESIAN_POINT('Ctrl Pts',(1.25092513683212,-38.2742356128,10.8236880870954));
#62901=CARTESIAN_POINT('Ctrl Pts',(1.40294280938938,-38.2742356128,10.7839166298021));
#62902=CARTESIAN_POINT('Ctrl Pts',(1.55603723521693,-38.2742356128,10.7438634681123));
#62903=CARTESIAN_POINT('Ctrl Pts',(1.70740879773239,-38.2742356128,10.6972445345565));
#62904=CARTESIAN_POINT('Ctrl Pts',(1.85650388541951,-38.2742356128,10.6442314384632));
#62905=CARTESIAN_POINT('Ctrl Pts',(2.00655796045027,-38.2742356128,10.5908773593839));
#62906=CARTESIAN_POINT('Ctrl Pts',(2.15430597357976,-38.2742356128,10.5310467305738));
#62907=CARTESIAN_POINT('Ctrl Pts',(2.29920241562008,-38.2742356128,10.464963920862));
#62908=CARTESIAN_POINT('Ctrl Pts',(2.44531547700217,-38.2742356128,10.3983262484957));
#62909=CARTESIAN_POINT('Ctrl Pts',(2.58852865334315,-38.2742356128,10.325331087339));
#62910=CARTESIAN_POINT('Ctrl Pts',(2.72830498882052,-38.2742356128,10.24625667601));
#62911=CARTESIAN_POINT('Ctrl Pts',(2.86857898067867,-38.2742356128,10.1669007300048));
#62912=CARTESIAN_POINT('Ctrl Pts',(3.00539139940937,-38.2742356128,10.0814223376914));
#62913=CARTESIAN_POINT('Ctrl Pts',(3.1382253222981,-38.2742356128,9.99014874576276));
#62914=CARTESIAN_POINT('Ctrl Pts',(3.27158660817497,-38.2742356128,9.89851278921275));
#62915=CARTESIAN_POINT('Ctrl Pts',(3.40093752166825,-38.2742356128,9.80103569854775));
#62916=CARTESIAN_POINT('Ctrl Pts',(3.52578422220404,-38.2742356128,9.69809237381965));
#62917=CARTESIAN_POINT('Ctrl Pts',(3.63868710847119,-38.2742356128,9.60499741469088));
#62918=CARTESIAN_POINT('Ctrl Pts',(3.74790663024948,-38.2742356128,9.50743272839668));
#62919=CARTESIAN_POINT('Ctrl Pts',(3.85310031128157,-38.2742356128,9.40570437828926));
#62920=CARTESIAN_POINT('Ctrl Pts',(3.96946942632073,-38.2742356128,9.29316873964397));
#62921=CARTESIAN_POINT('Ctrl Pts',(4.08091079548935,-38.2742356128,9.17553770727189));
#62922=CARTESIAN_POINT('Ctrl Pts',(4.18699742316105,-38.2742356128,9.05326075891791));
#62923=CARTESIAN_POINT('Ctrl Pts',(4.29267288764379,-38.2742356128,8.93145772307417));
#62924=CARTESIAN_POINT('Ctrl Pts',(4.39303483490137,-38.2742356128,8.8050449466975));
#62925=CARTESIAN_POINT('Ctrl Pts',(4.48769986111669,-38.2742356128,8.67450088215508));
#62926=CARTESIAN_POINT('Ctrl Pts',(4.58196381342408,-38.2742356128,8.54450990274046));
#62927=CARTESIAN_POINT('Ctrl Pts',(4.67057882212817,-38.2742356128,8.41042279546363));
#62928=CARTESIAN_POINT('Ctrl Pts',(4.75320767903444,-38.2742356128,8.27274247619464));
#62929=CARTESIAN_POINT('Ctrl Pts',(4.83538544616229,-38.2742356128,8.13581378519496));
#62930=CARTESIAN_POINT('Ctrl Pts',(4.91164206561261,-38.2742356128,7.99533123305691));
#62931=CARTESIAN_POINT('Ctrl Pts',(4.98168954890516,-38.2742356128,7.85181640625091));
#62932=CARTESIAN_POINT('Ctrl Pts',(5.05128204576803,-38.2742356128,7.70923376566466));
#62933=CARTESIAN_POINT('Ctrl Pts',(5.11474564573329,-38.2742356128,7.56365833443839));
#62934=CARTESIAN_POINT('Ctrl Pts',(5.17184371427649,-38.2742356128,7.41562486313624));
#62935=CARTESIAN_POINT('Ctrl Pts',(5.22816763835185,-38.2742356128,7.26959845259441));
#62936=CARTESIAN_POINT('Ctrl Pts',(5.27829737858524,-38.2742356128,7.12118043150776));
#62937=CARTESIAN_POINT('Ctrl Pts',(5.3220522683345,-38.2742356128,6.97090344328457));
#62938=CARTESIAN_POINT('Ctrl Pts',(5.36561634579287,-38.2742356128,6.8212818034477));
#62939=CARTESIAN_POINT('Ctrl Pts',(5.40286095423434,-38.2742356128,6.66981726674409));
#62940=CARTESIAN_POINT('Ctrl Pts',(5.43365592808345,-38.2742356128,6.51705274736088));
#62941=CARTESIAN_POINT('Ctrl Pts',(5.46427229224842,-38.2742356128,6.36517425641491));
#62942=CARTESIAN_POINT('Ctrl Pts',(5.48851348780113,-38.2742356128,6.21201176152061));
#62943=CARTESIAN_POINT('Ctrl Pts',(5.50630233117215,-38.2742356128,6.05810659766053));
#62944=CARTESIAN_POINT('Ctrl Pts',(5.52221910466512,-38.2742356128,5.92039817100981));
#62945=CARTESIAN_POINT('Ctrl Pts',(5.5329706903284,-38.2742356128,5.7820954092002));
#62946=CARTESIAN_POINT('Ctrl Pts',(5.53853645057666,-38.2742356128,5.6435933685011));
#62947=CARTESIAN_POINT('Ctrl Pts',(5.5390268466287,-38.2742356128,5.63139003042518));
#62948=CARTESIAN_POINT('Ctrl Pts',(5.53947703988333,-38.2742356128,5.61918414506667));
#62949=CARTESIAN_POINT('Ctrl Pts',(5.53988693785,-38.2742356128,5.6069786219));
#62950=CARTESIAN_POINT('',(4.6779495981,-38.2742356128,1.76615927471));
#62951=CARTESIAN_POINT('Ctrl Pts',(5.53988693785,-38.2742356128,5.6069786219));
#62952=CARTESIAN_POINT('Ctrl Pts',(5.5408707778169,-38.2742356128,5.57768291907289));
#62953=CARTESIAN_POINT('Ctrl Pts',(5.5417145820876,-38.2742356128,5.54821580128025));
#62954=CARTESIAN_POINT('Ctrl Pts',(5.54238546405316,-38.2742356128,5.51860736517105));
#62955=CARTESIAN_POINT('Ctrl Pts',(5.54360264640407,-38.2742356128,5.46488872654174));
#62956=CARTESIAN_POINT('Ctrl Pts',(5.54424776974383,-38.2742356128,5.41070491753419));
#62957=CARTESIAN_POINT('Ctrl Pts',(5.54416647607367,-38.2742356128,5.356201243868));
#62958=CARTESIAN_POINT('Ctrl Pts',(5.54408327235616,-38.2742356128,5.30041697114259));
#62959=CARTESIAN_POINT('Ctrl Pts',(5.54323922336175,-38.2742356128,5.24429785430791));
#62960=CARTESIAN_POINT('Ctrl Pts',(5.54152183085376,-38.2742356128,5.18799081545841));
#62961=CARTESIAN_POINT('Ctrl Pts',(5.53976334092991,-38.2742356128,5.13033634218082));
#62962=CARTESIAN_POINT('Ctrl Pts',(5.53708939114766,-38.2742356128,5.07248493669536));
#62963=CARTESIAN_POINT('Ctrl Pts',(5.533431865951,-38.2742356128,5.01457955231402));
#62964=CARTESIAN_POINT('Ctrl Pts',(5.53019201388825,-38.2742356128,4.9632867056636));
#62965=CARTESIAN_POINT('Ctrl Pts',(5.52618150714167,-38.2742356128,4.91195309409164));
#62966=CARTESIAN_POINT('Ctrl Pts',(5.52138355179064,-38.2742356128,4.86066207249638));
#62967=CARTESIAN_POINT('Ctrl Pts',(5.51558760341417,-38.2742356128,4.79870232264617));
#62968=CARTESIAN_POINT('Ctrl Pts',(5.50864099523777,-38.2742356128,4.73680019248161));
#62969=CARTESIAN_POINT('Ctrl Pts',(5.50056362356443,-38.2742356128,4.67509378178074));
#62970=CARTESIAN_POINT('Ctrl Pts',(5.49221771425977,-38.2742356128,4.61133590012658));
#62971=CARTESIAN_POINT('Ctrl Pts',(5.48266496019185,-38.2742356128,4.54778714929663));
#62972=CARTESIAN_POINT('Ctrl Pts',(5.47197926103978,-38.2742356128,4.48457601750013));
#62973=CARTESIAN_POINT('Ctrl Pts',(5.46089265811182,-38.2742356128,4.41899334397718));
#62974=CARTESIAN_POINT('Ctrl Pts',(5.4485869730846,-38.2742356128,4.35377433151512));
#62975=CARTESIAN_POINT('Ctrl Pts',(5.43519340909869,-38.2742356128,4.28903396005194));
#62976=CARTESIAN_POINT('Ctrl Pts',(5.42264344003186,-38.2742356128,4.22837126712776));
#62977=CARTESIAN_POINT('Ctrl Pts',(5.40913973384347,-38.2742356128,4.16813036669957));
#62978=CARTESIAN_POINT('Ctrl Pts',(5.39481880192551,-38.2742356128,4.10837559914741));
#62979=CARTESIAN_POINT('Ctrl Pts',(5.3781374913988,-38.2742356128,4.0387720399168));
#62980=CARTESIAN_POINT('Ctrl Pts',(5.36034716023229,-38.2742356128,3.96982796097921));
#62981=CARTESIAN_POINT('Ctrl Pts',(5.3417000881902,-38.2742356128,3.90161742158706));
#62982=CARTESIAN_POINT('Ctrl Pts',(5.32221924839775,-38.2742356128,3.83035697989119));
#62983=CARTESIAN_POINT('Ctrl Pts',(5.3018051238064,-38.2742356128,3.75989900003693));
#62984=CARTESIAN_POINT('Ctrl Pts',(5.28076410474724,-38.2742356128,3.69026592387477));
#62985=CARTESIAN_POINT('Ctrl Pts',(5.27503606815184,-38.2742356128,3.67130957925166));
#62986=CARTESIAN_POINT('Ctrl Pts',(5.26926164898527,-38.2742356128,3.65241415260537));
#62987=CARTESIAN_POINT('Ctrl Pts',(5.26344711753933,-38.2742356128,3.63357953459848));
#62988=CARTESIAN_POINT('Ctrl Pts',(5.24611610407497,-38.2742356128,3.57744035617824));
#62989=CARTESIAN_POINT('Ctrl Pts',(5.22843389032803,-38.2742356128,3.52185747179269));
#62990=CARTESIAN_POINT('Ctrl Pts',(5.2105541140774,-38.2742356128,3.46672743974292));
#62991=CARTESIAN_POINT('Ctrl Pts',(5.1858694840972,-38.2742356128,3.39061550059619));
#62992=CARTESIAN_POINT('Ctrl Pts',(5.1607833225832,-38.274235612979,3.31530922761688));
#62993=CARTESIAN_POINT('Ctrl Pts',(5.13571635392379,-38.2742356120079,3.24065429314394));
#62994=CARTESIAN_POINT('Ctrl Pts',(5.11431248675456,-38.2742356111787,3.17690887890189));
#62995=CARTESIAN_POINT('Ctrl Pts',(5.09292396027743,-38.2742356093749,3.11363951367482));
#62996=CARTESIAN_POINT('Ctrl Pts',(5.07177465707568,-38.2742356058314,3.05075329270464));
#62997=CARTESIAN_POINT('Ctrl Pts',(5.05292453439443,-38.2742356026731,2.99470355106825));
#62998=CARTESIAN_POINT('Ctrl Pts',(5.03426482326032,-38.2742355981201,2.93895860539514));
#62999=CARTESIAN_POINT('Ctrl Pts',(5.01591135851897,-38.2742355924515,2.88344603236812));
#63000=CARTESIAN_POINT('Ctrl Pts',(5.0101086493214,-38.2742355906593,2.86589494200869));
#63001=CARTESIAN_POINT('Ctrl Pts',(5.00433618370494,-38.2742355887626,2.84836700203233));
#63002=CARTESIAN_POINT('Ctrl Pts',(4.99859652036895,-38.2742355867898,2.83085967177776));
#63003=CARTESIAN_POINT('Ctrl Pts',(4.98176280681453,-38.2742355810037,2.77951286529167));
#63004=CARTESIAN_POINT('Ctrl Pts',(4.96522842306461,-38.2742355779867,2.72836284548135));
#63005=CARTESIAN_POINT('Ctrl Pts',(4.94899975664859,-38.2742355797489,2.67725154299494));
#63006=CARTESIAN_POINT('Ctrl Pts',(4.93277109023257,-38.2742355815112,2.62614024050852));
#63007=CARTESIAN_POINT('Ctrl Pts',(4.91684884973871,-38.2742355882266,2.57506820416811));
#63008=CARTESIAN_POINT('Ctrl Pts',(4.90118858468214,-38.2742355962476,2.52386041864114));
#63009=CARTESIAN_POINT('Ctrl Pts',(4.8873576701826,-38.2742356033317,2.47863445977162));
#63010=CARTESIAN_POINT('Ctrl Pts',(4.87370757924121,-38.2742356092055,2.43323262376226));
#63011=CARTESIAN_POINT('Ctrl Pts',(4.86023592795867,-38.2742356113118,2.38779762831885));
#63012=CARTESIAN_POINT('Ctrl Pts',(4.85845407162556,-38.2742356115904,2.38178807294382));
#63013=CARTESIAN_POINT('Ctrl Pts',(4.8566752645847,-38.274235611819,2.37577791889541));
#63014=CARTESIAN_POINT('Ctrl Pts',(4.8548994354018,-38.2742356120049,2.36976748068112));
#63015=CARTESIAN_POINT('Ctrl Pts',(4.84118585806346,-38.2742356134407,2.32335276349828));
#63016=CARTESIAN_POINT('Ctrl Pts',(4.82764687675358,-38.2742356128,2.27693340916131));
#63017=CARTESIAN_POINT('Ctrl Pts',(4.81416496783716,-38.2742356128,2.23034909238133));
#63018=CARTESIAN_POINT('Ctrl Pts',(4.81270177571342,-38.2742356128,2.2252932945841));
#63019=CARTESIAN_POINT('Ctrl Pts',(4.81123920827819,-38.2742356128,2.22023553573263));
#63020=CARTESIAN_POINT('Ctrl Pts',(4.80977707990551,-38.2742356128,2.21517559722572));
#63021=CARTESIAN_POINT('Ctrl Pts',(4.79712845252832,-38.2742356128,2.17140291767094));
#63022=CARTESIAN_POINT('Ctrl Pts',(4.78448254464563,-38.2742356128,2.12735099607628));
#63023=CARTESIAN_POINT('Ctrl Pts',(4.77169660280957,-38.2742356128,2.08292184394826));
#63024=CARTESIAN_POINT('Ctrl Pts',(4.75910524756551,-38.2742356128,2.03916884985447));
#63025=CARTESIAN_POINT('Ctrl Pts',(4.74637822653476,-38.2742356128,1.99505008609926));
#63026=CARTESIAN_POINT('Ctrl Pts',(4.73333245418105,-38.2742356128,1.95045340767228));
#63027=CARTESIAN_POINT('Ctrl Pts',(4.72050617381001,-38.2742356128,1.90660705763549));
#63028=CARTESIAN_POINT('Ctrl Pts',(4.70737184763075,-38.2742356128,1.86229877714485));
#63029=CARTESIAN_POINT('Ctrl Pts',(4.69370843473059,-38.2742356128,1.8174031505342));
#63030=CARTESIAN_POINT('Ctrl Pts',(4.69099699337357,-38.2742356128,1.80849382022039));
#63031=CARTESIAN_POINT('Ctrl Pts',(4.68826456393529,-38.2742356128,1.79956129861167));
#63032=CARTESIAN_POINT('Ctrl Pts',(4.68550919055206,-38.2742356128,1.79060451360579));
#63033=CARTESIAN_POINT('Ctrl Pts',(4.68300579177684,-38.2742356128,1.78246681265023));
#63034=CARTESIAN_POINT('Ctrl Pts',(4.68048944473333,-38.2742356128,1.77432846099333));
#63035=CARTESIAN_POINT('Ctrl Pts',(4.6779495981,-38.2742356128,1.76615927471));
#63036=CARTESIAN_POINT('',(0.665818565616232,-38.2742356128,-2.24488964565501));
#63037=CARTESIAN_POINT('Ctrl Pts',(4.67793826508075,-38.2742356128,1.76612282898476));
#63038=CARTESIAN_POINT('Ctrl Pts',(4.66625916152122,-38.2742356128,1.72856428599569));
#63039=CARTESIAN_POINT('Ctrl Pts',(4.6543341741093,-38.2742356127995,1.69115199273253));
#63040=CARTESIAN_POINT('Ctrl Pts',(4.64214427561065,-38.2742356127994,1.65382542234142));
#63041=CARTESIAN_POINT('Ctrl Pts',(4.61351356519473,-38.274235612799,1.5661556006603));
#63042=CARTESIAN_POINT('Ctrl Pts',(4.58345943425045,-38.2742356127991,1.47908977905003));
#63043=CARTESIAN_POINT('Ctrl Pts',(4.55201232353028,-38.2742356127993,1.39274184425048));
#63044=CARTESIAN_POINT('Ctrl Pts',(4.52087865885848,-38.2742356127995,1.30725457417742));
#63045=CARTESIAN_POINT('Ctrl Pts',(4.48838047126944,-38.2742356127998,1.22247155017572));
#63046=CARTESIAN_POINT('Ctrl Pts',(4.45453692836458,-38.2742356127999,1.13845087330955));
#63047=CARTESIAN_POINT('Ctrl Pts',(4.42346864479657,-38.2742356128,1.06132011244941));
#63048=CARTESIAN_POINT('Ctrl Pts',(4.39126697360346,-38.2742356128,0.98483161327673));
#63049=CARTESIAN_POINT('Ctrl Pts',(4.3579300357631,-38.2742356128,0.908984266315246));
#63050=CARTESIAN_POINT('Ctrl Pts',(4.35495212268333,-38.2742356128,0.902208994763186));
#63051=CARTESIAN_POINT('Ctrl Pts',(4.351965136915,-38.2742356128,0.895438807446463));
#63052=CARTESIAN_POINT('Ctrl Pts',(4.34896906853151,-38.2742356128,0.888673684522422));
#63053=CARTESIAN_POINT('Ctrl Pts',(4.31737828769537,-38.2742356128,0.817341695973576));
#63054=CARTESIAN_POINT('Ctrl Pts',(4.28477673375403,-38.2742356128,0.746569834090829));
#63055=CARTESIAN_POINT('Ctrl Pts',(4.2511436165332,-38.2742356128,0.676318084245987));
#63056=CARTESIAN_POINT('Ctrl Pts',(4.218057486707,-38.2742356128,0.607208863693416));
#63057=CARTESIAN_POINT('Ctrl Pts',(4.18397338482654,-38.2742356128,0.538603157868374));
#63058=CARTESIAN_POINT('Ctrl Pts',(4.14884788520354,-38.2742356128,0.47041966398888));
#63059=CARTESIAN_POINT('Ctrl Pts',(4.113432034225,-38.2742356128,0.401672557631684));
#63060=CARTESIAN_POINT('Ctrl Pts',(4.0769545471813,-38.2742356128921,0.333349597983933));
#63061=CARTESIAN_POINT('Ctrl Pts',(4.03940122487231,-38.274235612524,0.265434758630409));
#63062=CARTESIAN_POINT('Ctrl Pts',(4.00184790256332,-38.2742356121559,0.197519919276885));
#63063=CARTESIAN_POINT('Ctrl Pts',(3.96321789575712,-38.2742356113281,0.130011089054838));
#63064=CARTESIAN_POINT('Ctrl Pts',(3.92344185138896,-38.2742356083775,0.0629003525950581));
#63065=CARTESIAN_POINT('Ctrl Pts',(3.88612562855177,-38.2742356056093,-6.01362187938465E-5));
#63066=CARTESIAN_POINT('Ctrl Pts',(3.84781048176032,-38.2742356015818,-0.0626636364542783));
#63067=CARTESIAN_POINT('Ctrl Pts',(3.80840389490981,-38.2742355992333,-0.124899081227493));
#63068=CARTESIAN_POINT('Ctrl Pts',(3.77176973331138,-38.27423559705,-0.18275599102843));
#63069=CARTESIAN_POINT('Ctrl Pts',(3.73419160393593,-38.2742355967026,-0.240295480291296));
#63070=CARTESIAN_POINT('Ctrl Pts',(3.69557523382837,-38.2742355994774,-0.297467499682426));
#63071=CARTESIAN_POINT('Ctrl Pts',(3.68694928634095,-38.2742356000972,-0.310238322927692));
#63072=CARTESIAN_POINT('Ctrl Pts',(3.67827147240523,-38.2742356008542,-0.3229906163664));
#63073=CARTESIAN_POINT('Ctrl Pts',(3.66954064238787,-38.2742356017192,-0.335723465675104));
#63074=CARTESIAN_POINT('Ctrl Pts',(3.63311022119051,-38.2742356053286,-0.388852785846986));
#63075=CARTESIAN_POINT('Ctrl Pts',(3.59575012859676,-38.274235608571,-0.441644506020237));
#63076=CARTESIAN_POINT('Ctrl Pts',(3.5573773434737,-38.2742356103788,-0.493982525844108));
#63077=CARTESIAN_POINT('Ctrl Pts',(3.52096146858376,-38.2742356120944,-0.543651445516754));
#63078=CARTESIAN_POINT('Ctrl Pts',(3.48363327179107,-38.274235612611,-0.592911952877165));
#63079=CARTESIAN_POINT('Ctrl Pts',(3.4453206588264,-38.274235612743,-0.641618100247041));
#63080=CARTESIAN_POINT('Ctrl Pts',(3.4244230264332,-38.2742356128151,-0.668184890770134));
#63081=CARTESIAN_POINT('Ctrl Pts',(3.40323251844803,-38.2742356128,-0.69458590493586));
#63082=CARTESIAN_POINT('Ctrl Pts',(3.38173771803535,-38.2742356128,-0.720790831280737));
#63083=CARTESIAN_POINT('Ctrl Pts',(3.33624725963509,-38.2742356128,-0.77624955101233));
#63084=CARTESIAN_POINT('Ctrl Pts',(3.28938062812393,-38.2742356128,-0.830852886945385));
#63085=CARTESIAN_POINT('Ctrl Pts',(3.24111081333509,-38.2742356128,-0.884357982845603));
#63086=CARTESIAN_POINT('Ctrl Pts',(3.19288461412186,-38.2742356128,-0.937814732681796));
#63087=CARTESIAN_POINT('Ctrl Pts',(3.14325806188673,-38.2742356128,-0.990174807210689));
#63088=CARTESIAN_POINT('Ctrl Pts',(3.09224670761339,-38.2742356128,-1.04122585806989));
#63089=CARTESIAN_POINT('Ctrl Pts',(3.07805424639482,-38.2742356128,-1.05542936373657));
#63090=CARTESIAN_POINT('Ctrl Pts',(3.06375482962459,-38.2742356128,-1.06953173993419));
#63091=CARTESIAN_POINT('Ctrl Pts',(3.04934932888766,-38.2742356128,-1.08352889162963));
#63092=CARTESIAN_POINT('Ctrl Pts',(2.99733269917098,-38.2742356128,-1.13407101926035));
#63093=CARTESIAN_POINT('Ctrl Pts',(2.94390821224003,-38.2742356128,-1.18325961424795));
#63094=CARTESIAN_POINT('Ctrl Pts',(2.88913019863473,-38.2742356128,-1.2309284391068));
#63095=CARTESIAN_POINT('Ctrl Pts',(2.83542091306856,-38.2742356128,-1.27766723736619));
#63096=CARTESIAN_POINT('Ctrl Pts',(2.78041078264352,-38.2742356128,-1.32294475248435));
#63097=CARTESIAN_POINT('Ctrl Pts',(2.7241807257774,-38.2742356128,-1.36664371639806));
#63098=CARTESIAN_POINT('Ctrl Pts',(2.68656652166145,-38.2742356128,-1.39587544476389));
#63099=CARTESIAN_POINT('Ctrl Pts',(2.64840877536037,-38.2742356128,-1.4244005783711));
#63100=CARTESIAN_POINT('Ctrl Pts',(2.60972219620018,-38.2742356128,-1.45220579524711));
#63101=CARTESIAN_POINT('Ctrl Pts',(2.55332475186832,-38.2742356128,-1.49274034766661));
#63102=CARTESIAN_POINT('Ctrl Pts',(2.49581071755516,-38.2742356128,-1.53173612384503));
#63103=CARTESIAN_POINT('Ctrl Pts',(2.43730150766331,-38.2742356128,-1.56914474154156));
#63104=CARTESIAN_POINT('Ctrl Pts',(2.37879229777147,-38.2742356128,-1.60655335923809));
#63105=CARTESIAN_POINT('Ctrl Pts',(2.31928819316852,-38.2742356128,-1.64237451439411));
#63106=CARTESIAN_POINT('Ctrl Pts',(2.25892891673801,-38.2742356128,-1.6766100621915));
#63107=CARTESIAN_POINT('Ctrl Pts',(2.19511841977279,-38.2742356128,-1.71280312890831));
#63108=CARTESIAN_POINT('Ctrl Pts',(2.13031943918726,-38.2742356128252,-1.74724581047013));
#63109=CARTESIAN_POINT('Ctrl Pts',(2.06475207097091,-38.2742356127748,-1.77998075758362));
#63110=CARTESIAN_POINT('Ctrl Pts',(1.9952421880732,-38.2742356127214,-1.81468403152032));
#63111=CARTESIAN_POINT('Ctrl Pts',(1.92486912697262,-38.274235612856,-1.84746868240433));
#63112=CARTESIAN_POINT('Ctrl Pts',(1.8538610151458,-38.2742356108741,-1.87843249901246));
#63113=CARTESIAN_POINT('Ctrl Pts',(1.84076584838186,-38.2742356105085,-1.88414278100278));
#63114=CARTESIAN_POINT('Ctrl Pts',(1.82764898574597,-38.2742356100572,-1.88979124085339));
#63115=CARTESIAN_POINT('Ctrl Pts',(1.81451172471327,-38.2742356094821,-1.89537862184467));
#63116=CARTESIAN_POINT('Ctrl Pts',(1.73807179708742,-38.2742356061358,-1.92788912746134));
#63117=CARTESIAN_POINT('Ctrl Pts',(1.66096465259571,-38.2742356025828,-1.95834639660289));
#63118=CARTESIAN_POINT('Ctrl Pts',(1.58339648228159,-38.2742356015641,-1.98692473901088));
#63119=CARTESIAN_POINT('Ctrl Pts',(1.50608662566594,-38.2742356005489,-2.01540791123124));
#63120=CARTESIAN_POINT('Ctrl Pts',(1.42831878001412,-38.2742356016823,-2.04202631360568));
#63121=CARTESIAN_POINT('Ctrl Pts',(1.35024806210187,-38.2742356035753,-2.06695847219112));
#63122=CARTESIAN_POINT('Ctrl Pts',(1.27521671791387,-38.2742356053945,-2.09091999607869));
#63123=CARTESIAN_POINT('Ctrl Pts',(1.19990534194343,-38.2742356077503,-2.11332534295206));
#63124=CARTESIAN_POINT('Ctrl Pts',(1.12440899952419,-38.2742356094292,-2.13431684042754));
#63125=CARTESIAN_POINT('Ctrl Pts',(1.05063454131336,-38.2742356110698,-2.15482957394101));
#63126=CARTESIAN_POINT('Ctrl Pts',(0.976683314121403,-38.2742356120552,
-2.17399333744373));
#63127=CARTESIAN_POINT('Ctrl Pts',(0.902605394673177,-38.2742356124601,
-2.19190749111279));
#63128=CARTESIAN_POINT('Ctrl Pts',(0.834186928837262,-38.2742356128341,
-2.2084530274874));
#63129=CARTESIAN_POINT('Ctrl Pts',(0.765659995525827,-38.2742356127997,
-2.22393298752294));
#63130=CARTESIAN_POINT('Ctrl Pts',(0.697035032190242,-38.2742356128,-2.23838703956805));
#63131=CARTESIAN_POINT('Ctrl Pts',(0.691358497472616,-38.2742356128,-2.23958265300457));
#63132=CARTESIAN_POINT('Ctrl Pts',(0.68568127619484,-38.2742356128,-2.24077122154839));
#63133=CARTESIAN_POINT('Ctrl Pts',(0.680003365706886,-38.2742356128,-2.24195275347034));
#63134=CARTESIAN_POINT('Ctrl Pts',(0.675275609675362,-38.2742356128,-2.24293656515288));
#63135=CARTESIAN_POINT('Ctrl Pts',(0.670548709585667,-38.2742356128,-2.24391524728333));
#63136=CARTESIAN_POINT('Ctrl Pts',(0.665818566089,-38.2742356128,-2.24488964795));
#63137=CARTESIAN_POINT('',(-0.665819792855,-38.2742356128,-2.24488937901));
#63138=CARTESIAN_POINT('Origin',(0.000369776183994502,-38.2742356128,0.228538425659855));
#63139=CARTESIAN_POINT('',(-4.67790721121502,-38.2742356127993,1.7660251822171));
#63140=CARTESIAN_POINT('Ctrl Pts',(-0.665819792855,-38.2742356128,-2.24488937901));
#63141=CARTESIAN_POINT('Ctrl Pts',(-0.704646928243065,-38.2742356128,-2.23689100011484));
#63142=CARTESIAN_POINT('Ctrl Pts',(-0.743453331885261,-38.2742356128,-2.22856728027694));
#63143=CARTESIAN_POINT('Ctrl Pts',(-0.782230669443798,-38.2742356128,-2.21991217212279));
#63144=CARTESIAN_POINT('Ctrl Pts',(-0.861978408748563,-38.2742356128,-2.2021124635252));
#63145=CARTESIAN_POINT('Ctrl Pts',(-0.941609929902936,-38.2742356128618,
-2.18290567003262));
#63146=CARTESIAN_POINT('Ctrl Pts',(-1.02105429711175,-38.274235612313,-2.16219578205612));
#63147=CARTESIAN_POINT('Ctrl Pts',(-1.10290476162442,-38.2742356117475,
-2.14085866262982));
#63148=CARTESIAN_POINT('Ctrl Pts',(-1.18455818824905,-38.2742356103604,
-2.11792477960474));
#63149=CARTESIAN_POINT('Ctrl Pts',(-1.26591655734601,-38.2742356089745,
-2.09323731023742));
#63150=CARTESIAN_POINT('Ctrl Pts',(-1.3439080125386,-38.274235607646,-2.06957150077798));
#63151=CARTESIAN_POINT('Ctrl Pts',(-1.42162941951018,-38.2742356065559,
-2.0442927105919));
#63152=CARTESIAN_POINT('Ctrl Pts',(-1.49895641008838,-38.2742356071964,
-2.0172372185917));
#63153=CARTESIAN_POINT('Ctrl Pts',(-1.52916899268689,-38.2742356074466,
-2.00666631339175));
#63154=CARTESIAN_POINT('Ctrl Pts',(-1.55932085791326,-38.2742356079481,
-1.99582401911051));
#63155=CARTESIAN_POINT('Ctrl Pts',(-1.58940238356075,-38.2742356086409,
-1.98470018387681));
#63156=CARTESIAN_POINT('Ctrl Pts',(-1.65827743543357,-38.2742356102272,
-1.95923090623033));
#63157=CARTESIAN_POINT('Ctrl Pts',(-1.72679211337431,-38.2742356121567,
-1.93228407763729));
#63158=CARTESIAN_POINT('Ctrl Pts',(-1.79480399594728,-38.2742356125605,
-1.90371427925461));
#63159=CARTESIAN_POINT('Ctrl Pts',(-1.80225554318575,-38.2742356126047,
-1.90058410267092));
#63160=CARTESIAN_POINT('Ctrl Pts',(-1.80970100322648,-38.2742356126389,
-1.8974344502975));
#63161=CARTESIAN_POINT('Ctrl Pts',(-1.81714014934601,-38.2742356126655,
-1.8942651365982));
#63162=CARTESIAN_POINT('Ctrl Pts',(-1.88215012246053,-38.2742356128977,
-1.86656881297826));
#63163=CARTESIAN_POINT('Ctrl Pts',(-1.9466690398652,-38.2742356128,-1.83737781683262));
#63164=CARTESIAN_POINT('Ctrl Pts',(-2.01050469177384,-38.2742356128,-1.8066078872014));
#63165=CARTESIAN_POINT('Ctrl Pts',(-2.02064600006318,-38.2742356128,-1.80171959463914));
#63166=CARTESIAN_POINT('Ctrl Pts',(-2.03076996375684,-38.2742356128,-1.79679149040022));
#63167=CARTESIAN_POINT('Ctrl Pts',(-2.04087569583709,-38.2742356128,-1.79182328305228));
#63168=CARTESIAN_POINT('Ctrl Pts',(-2.10389818516883,-38.2742356128,-1.76083999632974));
#63169=CARTESIAN_POINT('Ctrl Pts',(-2.16623248706984,-38.2742356128,-1.72828190095184));
#63170=CARTESIAN_POINT('Ctrl Pts',(-2.22770535961108,-38.2742356128,-1.69410472600633));
#63171=CARTESIAN_POINT('Ctrl Pts',(-2.28968314957015,-38.2742356128,-1.65964683128625));
#63172=CARTESIAN_POINT('Ctrl Pts',(-2.3507852148703,-38.2742356128,-1.62354325629355));
#63173=CARTESIAN_POINT('Ctrl Pts',(-2.41085879928969,-38.2742356128,-1.58579533568302));
#63174=CARTESIAN_POINT('Ctrl Pts',(-2.45562897187998,-38.2742356128,-1.5576634880999));
#63175=CARTESIAN_POINT('Ctrl Pts',(-2.4998261921559,-38.2742356128,-1.52862112939009));
#63176=CARTESIAN_POINT('Ctrl Pts',(-2.54341537278903,-38.2742356128,-1.49867112182991));
#63177=CARTESIAN_POINT('Ctrl Pts',(-2.6033372665094,-38.2742356128,-1.45749895149135));
#63178=CARTESIAN_POINT('Ctrl Pts',(-2.66210134842506,-38.2742356128,-1.41461433672546));
#63179=CARTESIAN_POINT('Ctrl Pts',(-2.71958929396136,-38.2742356128,-1.37009585559334));
#63180=CARTESIAN_POINT('Ctrl Pts',(-2.76961721589123,-38.2742356128,-1.33135439287906));
#63181=CARTESIAN_POINT('Ctrl Pts',(-2.8186791267139,-38.2742356128,-1.29137639594389));
#63182=CARTESIAN_POINT('Ctrl Pts',(-2.8667147611275,-38.2742356128,-1.25024041056458));
#63183=CARTESIAN_POINT('Ctrl Pts',(-2.92283268399407,-38.2742356128,-1.20218304476235));
#63184=CARTESIAN_POINT('Ctrl Pts',(-2.97757449459017,-38.2742356128,-1.15252277207788));
#63185=CARTESIAN_POINT('Ctrl Pts',(-3.0308692710291,-38.2742356128,-1.10142066322325));
#63186=CARTESIAN_POINT('Ctrl Pts',(-3.08490320715715,-38.2742356128,-1.04960980538011));
#63187=CARTESIAN_POINT('Ctrl Pts',(-3.13744957757337,-38.2742356128,-0.996317007609141));
#63188=CARTESIAN_POINT('Ctrl Pts',(-3.18846749637239,-38.2742356128,-0.941752210541535));
#63189=CARTESIAN_POINT('Ctrl Pts',(-3.19984156223126,-38.2742356128,-0.929587394531143));
#63190=CARTESIAN_POINT('Ctrl Pts',(-3.21113979101621,-38.2742356128,-0.917359513398042));
#63191=CARTESIAN_POINT('Ctrl Pts',(-3.22236195773395,-38.2742356128,-0.90507115917739));
#63192=CARTESIAN_POINT('Ctrl Pts',(-3.26759437276338,-38.2742356128,-0.855541335559813));
#63193=CARTESIAN_POINT('Ctrl Pts',(-3.3115962220051,-38.2742356130343,-0.805026964631294));
#63194=CARTESIAN_POINT('Ctrl Pts',(-3.35442080548355,-38.2742356125657,
-0.753747455454356));
#63195=CARTESIAN_POINT('Ctrl Pts',(-3.39860538542766,-38.2742356120822,
-0.70083944354426));
#63196=CARTESIAN_POINT('Ctrl Pts',(-3.44153700222848,-38.2742356130572,
-0.647116843795417));
#63197=CARTESIAN_POINT('Ctrl Pts',(-3.48328433696875,-38.2742355963193,
-0.592765882196818));
#63198=CARTESIAN_POINT('Ctrl Pts',(-3.5004252969157,-38.2742355894469,-0.570450022714151));
#63199=CARTESIAN_POINT('Ctrl Pts',(-3.5173667001797,-38.2742355791753,-0.548027614240496));
#63200=CARTESIAN_POINT('Ctrl Pts',(-3.53411360439285,-38.2742355614603,
-0.525509056348052));
#63201=CARTESIAN_POINT('Ctrl Pts',(-3.5758719966679,-38.2742355172881,-0.469359050235111));
#63202=CARTESIAN_POINT('Ctrl Pts',(-3.61643933142103,-38.2742354330541,
-0.412633362231607));
#63203=CARTESIAN_POINT('Ctrl Pts',(-3.65591884381001,-38.2742353633462,
-0.355511048503402));
#63204=CARTESIAN_POINT('Ctrl Pts',(-3.66231665555709,-38.2742353520498,
-0.346254150743627));
#63205=CARTESIAN_POINT('Ctrl Pts',(-3.66868591455307,-38.2742353413087,
-0.336986727039308));
#63206=CARTESIAN_POINT('Ctrl Pts',(-3.67502707437779,-38.2742353315075,
-0.32770941450126));
#63207=CARTESIAN_POINT('Ctrl Pts',(-3.71582855026059,-38.274235268443,-0.268015595982058));
#63208=CARTESIAN_POINT('Ctrl Pts',(-3.75546633556578,-38.2742352456737,
-0.20791359818607));
#63209=CARTESIAN_POINT('Ctrl Pts',(-3.79406195827873,-38.2742352691212,
-0.147455189639169));
#63210=CARTESIAN_POINT('Ctrl Pts',(-3.79847911440783,-38.2742352718047,
-0.140535901619011));
#63211=CARTESIAN_POINT('Ctrl Pts',(-3.80288260521456,-38.2742352750323,
-0.133611891455309));
#63212=CARTESIAN_POINT('Ctrl Pts',(-3.80727260057058,-38.274235278769,-0.1266831960356));
#63213=CARTESIAN_POINT('Ctrl Pts',(-3.84951550837526,-38.2742353147257,
-0.0600115442261541));
#63214=CARTESIAN_POINT('Ctrl Pts',(-3.89050327927577,-38.274235371207,0.00711033372151271));
#63215=CARTESIAN_POINT('Ctrl Pts',(-3.93033830324993,-38.2742354234395,
0.074631574892402));
#63216=CARTESIAN_POINT('Ctrl Pts',(-3.96932598119582,-38.2742354745609,
0.140716545921541));
#63217=CARTESIAN_POINT('Ctrl Pts',(-4.00721011573223,-38.2742355208942,
0.207185040203976));
#63218=CARTESIAN_POINT('Ctrl Pts',(-4.04405961795798,-38.2742355520696,
0.274037052391819));
#63219=CARTESIAN_POINT('Ctrl Pts',(-4.08211043356015,-38.2742355842614,
0.343068475742127));
#63220=CARTESIAN_POINT('Ctrl Pts',(-4.11905913677954,-38.2742356005673,
0.412509522792078));
#63221=CARTESIAN_POINT('Ctrl Pts',(-4.15493864924535,-38.2742356072897,
0.482399519863388));
#63222=CARTESIAN_POINT('Ctrl Pts',(-4.18875568288618,-38.2742356136257,
0.548271997488862));
#63223=CARTESIAN_POINT('Ctrl Pts',(-4.22162316150445,-38.2742356127982,
0.614544288831008));
#63224=CARTESIAN_POINT('Ctrl Pts',(-4.25352261766768,-38.2742356127999,
0.681270513461267));
#63225=CARTESIAN_POINT('Ctrl Pts',(-4.25546814469304,-38.2742356128,0.685340102380078));
#63226=CARTESIAN_POINT('Ctrl Pts',(-4.2574100553188,-38.2742356128,0.689411384115315));
#63227=CARTESIAN_POINT('Ctrl Pts',(-4.25934833912097,-38.2742356128,0.693484372475847));
#63228=CARTESIAN_POINT('Ctrl Pts',(-4.28903323078085,-38.2742356128,0.755862347300288));
#63229=CARTESIAN_POINT('Ctrl Pts',(-4.31789233067801,-38.2742356128,0.818650643278417));
#63230=CARTESIAN_POINT('Ctrl Pts',(-4.34595980192137,-38.2742356128,0.881889756801076));
#63231=CARTESIAN_POINT('Ctrl Pts',(-4.37622528401063,-38.2742356128,0.950081231589276));
#63232=CARTESIAN_POINT('Ctrl Pts',(-4.40556985037429,-38.2742356127999,
1.01879649029968));
#63233=CARTESIAN_POINT('Ctrl Pts',(-4.43400163081888,-38.2742356127999,
1.08803594876579));
#63234=CARTESIAN_POINT('Ctrl Pts',(-4.46837585055085,-38.2742356127998,
1.17174693422715));
#63235=CARTESIAN_POINT('Ctrl Pts',(-4.50141511800001,-38.2742356127997,
1.25622383278628));
#63236=CARTESIAN_POINT('Ctrl Pts',(-4.53309301902471,-38.2742356127996,
1.34140008502369));
#63237=CARTESIAN_POINT('Ctrl Pts',(-4.5726759465089,-38.2742356127996,1.44783155007117));
#63238=CARTESIAN_POINT('Ctrl Pts',(-4.61012817527797,-38.2742356127997,
1.55535047338883));
#63239=CARTESIAN_POINT('Ctrl Pts',(-4.64538460757811,-38.2742356127999,
1.66376470978849));
#63240=CARTESIAN_POINT('Ctrl Pts',(-4.65528938830893,-38.2742356128,1.69422210917864));
#63241=CARTESIAN_POINT('Ctrl Pts',(-4.66502111917286,-38.2742356128,1.7247501570161));
#63242=CARTESIAN_POINT('Ctrl Pts',(-4.67457931908424,-38.2742356128,1.75534499646853));
#63243=CARTESIAN_POINT('Ctrl Pts',(-4.6756911332579,-38.2742356128,1.75890380214947));
#63244=CARTESIAN_POINT('Ctrl Pts',(-4.67680044999003,-38.2742356128,1.76246301601769));
#63245=CARTESIAN_POINT('Ctrl Pts',(-4.67790796861,-38.2742356128,1.76602494395));
#63246=CARTESIAN_POINT('',(-5.53988688529846,-38.2742356128,5.60698050627013));
#63247=CARTESIAN_POINT('Ctrl Pts',(-4.67800175055493,-38.2742356128,1.7663265757088));
#63248=CARTESIAN_POINT('Ctrl Pts',(-4.69251924365702,-38.2742356128,1.8130288213493));
#63249=CARTESIAN_POINT('Ctrl Pts',(-4.70639030202568,-38.274235612792,1.85910573504843));
#63250=CARTESIAN_POINT('Ctrl Pts',(-4.71985822559416,-38.2742356127938,
1.90464595121774));
#63251=CARTESIAN_POINT('Ctrl Pts',(-4.73322084691452,-38.2742356127955,
1.94983010008994));
#63252=CARTESIAN_POINT('Ctrl Pts',(-4.74618665047486,-38.2742356127992,
1.99448599975856));
#63253=CARTESIAN_POINT('Ctrl Pts',(-4.75894398307504,-38.2742356127998,
2.03868484514955));
#63254=CARTESIAN_POINT('Ctrl Pts',(-4.76431621360322,-38.2742356128,2.05729738696853));
#63255=CARTESIAN_POINT('Ctrl Pts',(-4.76965087070964,-38.2742356128,2.07582868278896));
#63256=CARTESIAN_POINT('Ctrl Pts',(-4.77495939222068,-38.2742356128,2.09428318197623));
#63257=CARTESIAN_POINT('Ctrl Pts',(-4.78796234557368,-38.2742356128,2.13948653880281));
#63258=CARTESIAN_POINT('Ctrl Pts',(-4.80084040354426,-38.2742356128176,
2.18432693740341));
#63259=CARTESIAN_POINT('Ctrl Pts',(-4.81375974350727,-38.2742356127822,
2.22898466812738));
#63260=CARTESIAN_POINT('Ctrl Pts',(-4.82734652173961,-38.274235612745,2.27594950421374));
#63261=CARTESIAN_POINT('Ctrl Pts',(-4.84097877771399,-38.2742356128325,
2.32271208442447));
#63262=CARTESIAN_POINT('Ctrl Pts',(-4.85479666640947,-38.2742356114848,
2.36946043386112));
#63263=CARTESIAN_POINT('Ctrl Pts',(-4.8587801405254,-38.2742356110963,2.38293722789582));
#63264=CARTESIAN_POINT('Ctrl Pts',(-4.86277872827033,-38.2742356105678,
2.39641271970806));
#63265=CARTESIAN_POINT('Ctrl Pts',(-4.86679505182229,-38.274235609794,2.40989114382001));
#63266=CARTESIAN_POINT('Ctrl Pts',(-4.88059037731783,-38.2742356071361,
2.45618702745232));
#63267=CARTESIAN_POINT('Ctrl Pts',(-4.89456039340916,-38.2742356002741,
2.50239264268077));
#63268=CARTESIAN_POINT('Ctrl Pts',(-4.90873520412703,-38.2742355926928,
2.54846227156529));
#63269=CARTESIAN_POINT('Ctrl Pts',(-4.91028381252858,-38.2742355918645,
2.55349541209652));
#63270=CARTESIAN_POINT('Ctrl Pts',(-4.91183481649938,-38.2742355910419,
2.55852691419768));
#63271=CARTESIAN_POINT('Ctrl Pts',(-4.91338821986879,-38.2742355902393,
2.56355670680289));
#63272=CARTESIAN_POINT('Ctrl Pts',(-4.92878136479561,-38.2742355822858,
2.61339844659059));
#63273=CARTESIAN_POINT('Ctrl Pts',(-4.94446242793141,-38.2742355777817,
2.66322253982865));
#63274=CARTESIAN_POINT('Ctrl Pts',(-4.96043781291716,-38.2742355779049,
2.71312250655352));
#63275=CARTESIAN_POINT('Ctrl Pts',(-4.97766141629314,-38.2742355780377,
2.76692134996855));
#63276=CARTESIAN_POINT('Ctrl Pts',(-4.99522708121126,-38.2742355830336,
2.82080823788669));
#63277=CARTESIAN_POINT('Ctrl Pts',(-5.01308247143858,-38.2742355888683,
2.87488233891121));
#63278=CARTESIAN_POINT('Ctrl Pts',(-5.03196312008577,-38.2742355950381,
2.93206138061001));
#63279=CARTESIAN_POINT('Ctrl Pts',(-5.05116721886563,-38.2742356017569,
2.98944941342246));
#63280=CARTESIAN_POINT('Ctrl Pts',(-5.07057244294407,-38.2742356059748,
3.04714821864261));
#63281=CARTESIAN_POINT('Ctrl Pts',(-5.0926331575463,-38.2742356107698,3.11274276522994));
#63282=CARTESIAN_POINT('Ctrl Pts',(-5.11495343239751,-38.2742356123442,
3.17873841755785));
#63283=CARTESIAN_POINT('Ctrl Pts',(-5.1372834033019,-38.2742356126751,3.24527209500931));
#63284=CARTESIAN_POINT('Ctrl Pts',(-5.14793271821097,-38.2742356128329,
3.27700245803906));
#63285=CARTESIAN_POINT('Ctrl Pts',(-5.15858332970118,-38.2742356128,3.30885507470597));
#63286=CARTESIAN_POINT('Ctrl Pts',(-5.1692042386179,-38.2742356128,3.34084464185392));
#63287=CARTESIAN_POINT('Ctrl Pts',(-5.18615827832582,-38.2742356128,3.39190923490501));
#63288=CARTESIAN_POINT('Ctrl Pts',(-5.2030376480001,-38.2742356128,3.44329909325076));
#63289=CARTESIAN_POINT('Ctrl Pts',(-5.21971989492434,-38.2742356128,3.49509480363394));
#63290=CARTESIAN_POINT('Ctrl Pts',(-5.23206581250308,-38.2742356128,3.53342690447306));
#63291=CARTESIAN_POINT('Ctrl Pts',(-5.24430626641809,-38.2742356128,3.57198986757135));
#63292=CARTESIAN_POINT('Ctrl Pts',(-5.2563876606808,-38.2742356128,3.61080945089639));
#63293=CARTESIAN_POINT('Ctrl Pts',(-5.26204241065736,-38.2742356128,3.62897912842896));
#63294=CARTESIAN_POINT('Ctrl Pts',(-5.2676622425971,-38.2742356128,3.64720481174824));
#63295=CARTESIAN_POINT('Ctrl Pts',(-5.2732416422671,-38.2742356128,3.66548897551996));
#63296=CARTESIAN_POINT('Ctrl Pts',(-5.29415732881792,-38.2742356128,3.73403144620004));
#63297=CARTESIAN_POINT('Ctrl Pts',(-5.31450074962474,-38.2742356128,3.80338813483685));
#63298=CARTESIAN_POINT('Ctrl Pts',(-5.33397236668635,-38.2742356128,3.87353289876993));
#63299=CARTESIAN_POINT('Ctrl Pts',(-5.35283131746884,-38.2742356128,3.94147058707169));
#63300=CARTESIAN_POINT('Ctrl Pts',(-5.37087127259599,-38.2742356128,4.01014719863215));
#63301=CARTESIAN_POINT('Ctrl Pts',(-5.38783722079999,-38.2742356128,4.07949471936758));
#63302=CARTESIAN_POINT('Ctrl Pts',(-5.40408962754407,-38.2742356128,4.14592567271799));
#63303=CARTESIAN_POINT('Ctrl Pts',(-5.41935563770956,-38.2742356128,4.21297193948276));
#63304=CARTESIAN_POINT('Ctrl Pts',(-5.43344131574358,-38.2742356128,4.28053748855896));
#63305=CARTESIAN_POINT('Ctrl Pts',(-5.4454597515054,-38.2742356128,4.33818698255723));
#63306=CARTESIAN_POINT('Ctrl Pts',(-5.45661884192655,-38.2742356128,4.39621219347407));
#63307=CARTESIAN_POINT('Ctrl Pts',(-5.46682548455427,-38.2742356128,4.45454748070309));
#63308=CARTESIAN_POINT('Ctrl Pts',(-5.47770583464895,-38.2742356128,4.51673329155941));
#63309=CARTESIAN_POINT('Ctrl Pts',(-5.48750209793833,-38.2742356128,4.57926820462705));
#63310=CARTESIAN_POINT('Ctrl Pts',(-5.49613554366455,-38.2742356128,4.6420318749869));
#63311=CARTESIAN_POINT('Ctrl Pts',(-5.50453362460369,-38.2742356128,4.70308448369432));
#63312=CARTESIAN_POINT('Ctrl Pts',(-5.51183107041303,-38.2742356128,4.76435340279378));
#63313=CARTESIAN_POINT('Ctrl Pts',(-5.51799936991938,-38.2742356128,4.82570765700624));
#63314=CARTESIAN_POINT('Ctrl Pts',(-5.5239505945413,-38.2742356128,4.88490273142708));
#63315=CARTESIAN_POINT('Ctrl Pts',(-5.52885055510356,-38.2742356128,4.94417709295067));
#63316=CARTESIAN_POINT('Ctrl Pts',(-5.53271894510559,-38.2742356128,5.003396179467));
#63317=CARTESIAN_POINT('Ctrl Pts',(-5.53470010105145,-38.2742356128,5.03372462238493));
#63318=CARTESIAN_POINT('Ctrl Pts',(-5.53641144935291,-38.2742356128,5.06403830324197));
#63319=CARTESIAN_POINT('Ctrl Pts',(-5.53786073495758,-38.2742356128,5.09431751427075));
#63320=CARTESIAN_POINT('Ctrl Pts',(-5.54057010536452,-38.2742356128,5.15092305705868));
#63321=CARTESIAN_POINT('Ctrl Pts',(-5.54236123784421,-38.2742356128,5.20742199664858));
#63322=CARTESIAN_POINT('Ctrl Pts',(-5.54331935811328,-38.2742356128,5.26367049854319));
#63323=CARTESIAN_POINT('Ctrl Pts',(-5.54427311748046,-38.2742356128,5.31966298435481));
#63324=CARTESIAN_POINT('Ctrl Pts',(-5.5444011346495,-38.2742356128,5.3754072468512));
#63325=CARTESIAN_POINT('Ctrl Pts',(-5.5438384561933,-38.2742356128,5.43074893164346));
#63326=CARTESIAN_POINT('Ctrl Pts',(-5.54327577773709,-38.2742356128,5.48609061643572));
#63327=CARTESIAN_POINT('Ctrl Pts',(-5.54202208977835,-38.2742356128,5.54102966902184));
#63328=CARTESIAN_POINT('Ctrl Pts',(-5.54026815741874,-38.2742356128,5.59540007603281));
#63329=CARTESIAN_POINT('Ctrl Pts',(-5.54014355072925,-38.2742356128,5.59926277711513));
#63330=CARTESIAN_POINT('Ctrl Pts',(-5.54001645927,-38.2742356128,5.60312234544667));
#63331=CARTESIAN_POINT('Ctrl Pts',(-5.53988688857,-38.2742356128,5.60698050638));
#63332=CARTESIAN_POINT('Ctrl Pts',(-5.53988688120902,-38.2742356128,5.60698050613279));
#63333=CARTESIAN_POINT('Ctrl Pts',(-5.53835461888468,-38.2742356128,5.65260642340235));
#63334=CARTESIAN_POINT('Ctrl Pts',(-5.536259875995,-38.2742356128,5.69821935187167));
#63335=CARTESIAN_POINT('Ctrl Pts',(-5.5336031510825,-38.2742356128,5.743797561555));
#63336=CARTESIAN_POINT('Ctrl Pts',(-5.53094642617,-38.2742356128,5.78937577123833));
#63337=CARTESIAN_POINT('Ctrl Pts',(-5.52772748735596,-38.2742356128,5.83492380218515));
#63338=CARTESIAN_POINT('Ctrl Pts',(-5.52394721644107,-38.2742356128,5.88042392815046));
#63339=CARTESIAN_POINT('Ctrl Pts',(-5.51115082727157,-38.2742356128,6.03444392624604));
#63340=CARTESIAN_POINT('Ctrl Pts',(-5.49191715811991,-38.2742356128,6.18793486599567));
#63341=CARTESIAN_POINT('Ctrl Pts',(-5.46630422780706,-38.2742356127999,
6.34035255218782));
#63342=CARTESIAN_POINT('Ctrl Pts',(-5.44035409258864,-38.2742356127999,
6.49477688076138));
#63343=CARTESIAN_POINT('Ctrl Pts',(-5.40785568517866,-38.2742356127999,
6.64809930316969));
#63344=CARTESIAN_POINT('Ctrl Pts',(-5.36892159353684,-38.2742356127999,
6.79976605176687));
#63345=CARTESIAN_POINT('Ctrl Pts',(-5.32969944639958,-38.2742356127999,
6.95255491310809));
#63346=CARTESIAN_POINT('Ctrl Pts',(-5.28394615822592,-38.2742356127999,
7.10366330310781));
#63347=CARTESIAN_POINT('Ctrl Pts',(-5.23182799159665,-38.2742356127999,
7.25254050637488));
#63348=CARTESIAN_POINT('Ctrl Pts',(-5.17936032583359,-38.2742356127999,
7.40241606505134));
#63349=CARTESIAN_POINT('Ctrl Pts',(-5.12044226986684,-38.2742356127999,
7.55003019609581));
#63350=CARTESIAN_POINT('Ctrl Pts',(-5.05529310484516,-38.2742356127999,
7.69483982044707));
#63351=CARTESIAN_POINT('Ctrl Pts',(-4.98976338672371,-38.2742356127999,
7.84049531521595));
#63352=CARTESIAN_POINT('Ctrl Pts',(-4.91792970568151,-38.2742356127999,
7.98331322084872));
#63353=CARTESIAN_POINT('Ctrl Pts',(-4.84006305112756,-38.2742356127999,
8.12276314875079));
#63354=CARTESIAN_POINT('Ctrl Pts',(-4.76166290620733,-38.2742356128,8.26316849452125));
#63355=CARTESIAN_POINT('Ctrl Pts',(-4.67714699130435,-38.2742356128,8.40015931653317));
#63356=CARTESIAN_POINT('Ctrl Pts',(-4.58683794520934,-38.2742356128,8.53322024142848));
#63357=CARTESIAN_POINT('Ctrl Pts',(-4.49629467958833,-38.2742356128,8.66662626427471));
#63358=CARTESIAN_POINT('Ctrl Pts',(-4.39992838652888,-38.2742356128,8.79608175399285));
#63359=CARTESIAN_POINT('Ctrl Pts',(-4.2981076828134,-38.2742356128,8.92109681428887));
#63360=CARTESIAN_POINT('Ctrl Pts',(-4.19608210028847,-38.2742356128,9.04636342398282));
#63361=CARTESIAN_POINT('Ctrl Pts',(-4.08858033437217,-38.2742356128,9.16717149106921));
#63362=CARTESIAN_POINT('Ctrl Pts',(-3.9760138595325,-38.2742356128,9.28306111775555));
#63363=CARTESIAN_POINT('Ctrl Pts',(-3.90539029603414,-38.2742356128,9.3557696077455));
#63364=CARTESIAN_POINT('Ctrl Pts',(-3.83277394124446,-38.2742356128,9.42654275117891));
#63365=CARTESIAN_POINT('Ctrl Pts',(-3.75827401203565,-38.2742356128,9.49527417891981));
#63366=CARTESIAN_POINT('Ctrl Pts',(-3.63965885290044,-38.2742356128,9.60470501094418));
#63367=CARTESIAN_POINT('Ctrl Pts',(-3.51626710819725,-38.2742356128,9.70895831597016));
#63368=CARTESIAN_POINT('Ctrl Pts',(-3.38856684804589,-38.2742356128,9.80763610928524));
#63369=CARTESIAN_POINT('Ctrl Pts',(-3.26114695780359,-38.2742356128,9.90609725242353));
#63370=CARTESIAN_POINT('Ctrl Pts',(-3.12943768874386,-38.2742356128,9.99900714103251));
#63371=CARTESIAN_POINT('Ctrl Pts',(-2.9939361381078,-38.2742356128,10.0860110380169));
#63372=CARTESIAN_POINT('Ctrl Pts',(-2.85892760240792,-38.2742356128,10.1726983761093));
#63373=CARTESIAN_POINT('Ctrl Pts',(-2.72015457125465,-38.2742356128,10.2535224381057));
#63374=CARTESIAN_POINT('Ctrl Pts',(-2.57813705267921,-38.2742356128,10.3281755642702));
#63375=CARTESIAN_POINT('Ctrl Pts',(-2.43727514445134,-38.2742356128,10.4022212306936));
#63376=CARTESIAN_POINT('Ctrl Pts',(-2.29322158416204,-38.2742356128,10.4701958383899));
#63377=CARTESIAN_POINT('Ctrl Pts',(-2.14650802776576,-38.2742356127999,
10.5318441397132));
#63378=CARTESIAN_POINT('Ctrl Pts',(-2.00061624306781,-38.2742356127999,
10.5931471366862));
#63379=CARTESIAN_POINT('Ctrl Pts',(-1.85209440527852,-38.2742356127999,
10.6481943461997));
#63380=CARTESIAN_POINT('Ctrl Pts',(-1.70148582143208,-38.2742356127999,
10.6967816414531));
#63381=CARTESIAN_POINT('Ctrl Pts',(-1.55244458158058,-38.2742356127999,
10.7448633014797));
#63382=CARTESIAN_POINT('Ctrl Pts',(-1.4013600311476,-38.2742356127999,10.7866186970661));
#63383=CARTESIAN_POINT('Ctrl Pts',(-1.24877544147231,-38.2742356127999,
10.8218978649459));
#63384=CARTESIAN_POINT('Ctrl Pts',(-1.11051101261617,-38.2742356127998,
10.8538660604747));
#63385=CARTESIAN_POINT('Ctrl Pts',(-0.97101520004087,-38.2742356127998,
10.8805170667324));
#63386=CARTESIAN_POINT('Ctrl Pts',(-0.830701999895475,-38.2742356127998,
10.9017749796494));
#63387=CARTESIAN_POINT('Ctrl Pts',(-0.677686947127854,-38.2742356127998,
10.9249572651603));
#63388=CARTESIAN_POINT('Ctrl Pts',(-0.523701733229498,-38.2742356127999,
10.941724955098));
#63389=CARTESIAN_POINT('Ctrl Pts',(-0.369289497635685,-38.2742356128,10.9520282985498));
#63390=CARTESIAN_POINT('Ctrl Pts',(-0.248348049539687,-38.2742356128,10.9600982631643));
#63391=CARTESIAN_POINT('Ctrl Pts',(-0.127144870043233,-38.2742356128,10.9642035478476));
#63392=CARTESIAN_POINT('Ctrl Pts',(-0.00594433456959664,-38.2742356128,
10.9643423600255));
#63393=CARTESIAN_POINT('Ctrl Pts',(-0.00397084641091772,-38.2742356128,
10.9643446202811));
#63394=CARTESIAN_POINT('Ctrl Pts',(-0.00199736053559199,-38.2742356128,
10.9643458293));
#63395=CARTESIAN_POINT('Ctrl Pts',(-2.39294621618E-5,-38.2742356128,10.9643459873));
#63396=CARTESIAN_POINT('Ctrl Pts',(-2.08574170933,-36.2742356128,-9.31728158894));
#63397=CARTESIAN_POINT('Ctrl Pts',(-2.06766727163,-36.2742356128,-9.22478316375));
#63398=CARTESIAN_POINT('Ctrl Pts',(-2.04959283393,-36.3112466293,-9.13228473856));
#63399=CARTESIAN_POINT('Ctrl Pts',(-2.03530680234,-36.3857400536,-9.05917400362));
#63400=CARTESIAN_POINT('Ctrl Pts',(-2.02820898726,-36.4799878332,-9.02284995699));
#63401=CARTESIAN_POINT('Ctrl Pts',(-2.02820898726,-36.5742356128,-9.02284995699));
#63402=CARTESIAN_POINT('Ctrl Pts',(-2.08911689677,-36.2742356128,-9.31662206836));
#63403=CARTESIAN_POINT('Ctrl Pts',(-2.07116027711,-36.2742356128,-9.22410062121));
#63404=CARTESIAN_POINT('Ctrl Pts',(-2.05320365744,-36.3112466293,-9.13157917406));
#63405=CARTESIAN_POINT('Ctrl Pts',(-2.03901074921,-36.3857400536,-9.05845024258));
#63406=CARTESIAN_POINT('Ctrl Pts',(-2.03195920116,-36.4799878332,-9.02211715524));
#63407=CARTESIAN_POINT('Ctrl Pts',(-2.03195920116,-36.5742356128,-9.02211715524));
#63408=CARTESIAN_POINT('Ctrl Pts',(-2.0924931363,-36.2742356128,-9.31596792123));
#63409=CARTESIAN_POINT('Ctrl Pts',(-2.0746543701,-36.2742356128,-9.22342363995));
#63410=CARTESIAN_POINT('Ctrl Pts',(-2.0568156039,-36.3112466293,-9.13087935867));
#63411=CARTESIAN_POINT('Ctrl Pts',(-2.04271584702,-36.3857400536,-9.05773237909));
#63412=CARTESIAN_POINT('Ctrl Pts',(-2.03571057991,-36.4799878332,-9.02139032482));
#63413=CARTESIAN_POINT('Ctrl Pts',(-2.03571057991,-36.5742356128,-9.02139032482));
#63414=CARTESIAN_POINT('Ctrl Pts',(-2.09585558711,-36.2742356128,-9.31532184587));
#63415=CARTESIAN_POINT('Ctrl Pts',(-2.07813573018,-36.2742356128,-9.22275473257));
#63416=CARTESIAN_POINT('Ctrl Pts',(-2.06041587325,-36.3112466293,-9.13018761926));
#63417=CARTESIAN_POINT('Ctrl Pts',(-2.04640963715,-36.3857400536,-9.05702267764));
#63418=CARTESIAN_POINT('Ctrl Pts',(-2.03945153068,-36.4799878332,-9.02067157287));
#63419=CARTESIAN_POINT('Ctrl Pts',(-2.03945153068,-36.5742356128,-9.02067157287));
#63420=CARTESIAN_POINT('Ctrl Pts',(-2.10264192286,-36.2742356128,-9.31402965523));
#63421=CARTESIAN_POINT('Ctrl Pts',(-2.08515587597,-36.2742356128,-9.22141799595));
#63422=CARTESIAN_POINT('Ctrl Pts',(-2.06766982907,-36.3112466293,-9.12880633666));
#63423=CARTESIAN_POINT('Ctrl Pts',(-2.05384932652,-36.3857400536,-9.05560601714));
#63424=CARTESIAN_POINT('Ctrl Pts',(-2.04698210689,-36.4799878332,-9.01923758796));
#63425=CARTESIAN_POINT('Ctrl Pts',(-2.04698210689,-36.5742356128,-9.01923758796));
#63426=CARTESIAN_POINT('Ctrl Pts',(-2.10937295423,-36.2742356128,-9.31276977998));
#63427=CARTESIAN_POINT('Ctrl Pts',(-2.09212493888,-36.2742356128,-9.22011358344));
#63428=CARTESIAN_POINT('Ctrl Pts',(-2.07487692352,-36.3112466293,-9.1274573869));
#63429=CARTESIAN_POINT('Ctrl Pts',(-2.06124363091,-36.3857400536,-9.0542220339));
#63430=CARTESIAN_POINT('Ctrl Pts',(-2.05447081618,-36.4799878332,-9.01783594623));
#63431=CARTESIAN_POINT('Ctrl Pts',(-2.05447081618,-36.5742356128,-9.01783594623));
#63432=CARTESIAN_POINT('Ctrl Pts',(-2.11282966913,-36.2742356128,-9.31212882607));
#63433=CARTESIAN_POINT('Ctrl Pts',(-2.09569451045,-36.2742356128,-9.21945167612));
#63434=CARTESIAN_POINT('Ctrl Pts',(-2.07855935176,-36.3112466293,-9.12677452618));
#63435=CARTESIAN_POINT('Ctrl Pts',(-2.06501758638,-36.3857400536,-9.05352218973));
#63436=CARTESIAN_POINT('Ctrl Pts',(-2.05828676503,-36.4799878332,-9.01712829556));
#63437=CARTESIAN_POINT('Ctrl Pts',(-2.05828676503,-36.5742356128,-9.01712829556));
#63438=CARTESIAN_POINT('Ctrl Pts',(-2.11610882906,-36.2742356128,-9.31152571954));
#63439=CARTESIAN_POINT('Ctrl Pts',(-2.09909881001,-36.2742356128,-9.21882557494));
#63440=CARTESIAN_POINT('Ctrl Pts',(-2.08208879095,-36.3112466293,-9.12612543034));
#63441=CARTESIAN_POINT('Ctrl Pts',(-2.06864283545,-36.3857400536,-9.05285548143));
#63442=CARTESIAN_POINT('Ctrl Pts',(-2.06196425677,-36.4799878332,-9.01645199477));
#63443=CARTESIAN_POINT('Ctrl Pts',(-2.06196425677,-36.5742356128,-9.01645199477));
#63444=CARTESIAN_POINT('Ctrl Pts',(-2.11953809664,-36.2742356128,-9.31090088679));
#63445=CARTESIAN_POINT('Ctrl Pts',(-2.10264304655,-36.2742356128,-9.21817979292));
#63446=CARTESIAN_POINT('Ctrl Pts',(-2.08574799646,-36.3112466293,-9.12545869905));
#63447=CARTESIAN_POINT('Ctrl Pts',(-2.07239415258,-36.3857400536,-9.05217196684));
#63448=CARTESIAN_POINT('Ctrl Pts',(-2.06575948192,-36.4799878332,-9.01576047842));
#63449=CARTESIAN_POINT('Ctrl Pts',(-2.06575948192,-36.5742356128,-9.01576047842));
#63450=CARTESIAN_POINT('',(-2.02820898726,-36.5742356128,-9.02284995699));
#63451=CARTESIAN_POINT('Origin',(-2.08533438268287,-36.5721143203773,-9.31519977054305));
#63452=CARTESIAN_POINT('',(-2.06575948151871,-36.5742356128,-9.01576047619305));
#63453=CARTESIAN_POINT('Origin',(-2.11915857361596,-36.5721143085717,-9.308813819988));
#63454=CARTESIAN_POINT('Origin',(-2.46533767222342,-36.5742356128,-11.2351029262791));
#63455=CARTESIAN_POINT('Ctrl Pts',(-2.06575948222,-37.9742356128,-9.01576048002));
#63456=CARTESIAN_POINT('Ctrl Pts',(-2.0657594822,-38.0684833925,-9.01576048002));
#63457=CARTESIAN_POINT('Ctrl Pts',(-2.07239441316,-38.1627311721,-9.05217192117));
#63458=CARTESIAN_POINT('Ctrl Pts',(-2.08574878097,-38.2372245964,-9.12545855823));
#63459=CARTESIAN_POINT('Ctrl Pts',(-2.10264449395,-38.2742356129,-9.21817953172));
#63460=CARTESIAN_POINT('Ctrl Pts',(-2.11954020693,-38.2742356128,-9.31090050519));
#63461=CARTESIAN_POINT('Ctrl Pts',(-2.05815374966,-37.9742356128,-9.01714631048));
#63462=CARTESIAN_POINT('Ctrl Pts',(-2.05815374989,-38.0684833923,-9.01714631044));
#63463=CARTESIAN_POINT('Ctrl Pts',(-2.06487519089,-38.1627311717,-9.05354198334));
#63464=CARTESIAN_POINT('Ctrl Pts',(-2.07840770897,-38.2372245959,-9.12679615488));
#63465=CARTESIAN_POINT('Ctrl Pts',(-2.09552712261,-38.2742356126,-9.21947635948));
#63466=CARTESIAN_POINT('Ctrl Pts',(-2.11264653618,-38.2742356128,-9.3121565642));
#63467=CARTESIAN_POINT('Ctrl Pts',(-2.05152801719,-37.9742356128,-9.01837808851));
#63468=CARTESIAN_POINT('Ctrl Pts',(-2.05152801591,-38.0684833934,-9.01837808874));
#63469=CARTESIAN_POINT('Ctrl Pts',(-2.05839882311,-38.162731174,-9.05474628549));
#63470=CARTESIAN_POINT('Ctrl Pts',(-2.07226541572,-38.2372245982,-9.12793903416));
#63471=CARTESIAN_POINT('Ctrl Pts',(-2.08975388938,-38.2742356144,-9.22055135079));
#63472=CARTESIAN_POINT('Ctrl Pts',(-2.10724236369,-38.2742356128,-9.3131636663));
#63473=CARTESIAN_POINT('Ctrl Pts',(-2.04377025976,-37.9742356128,-9.01983403466));
#63474=CARTESIAN_POINT('Ctrl Pts',(-2.04377013041,-38.0684833525,-9.01983405993));
#63475=CARTESIAN_POINT('Ctrl Pts',(-2.05055250717,-38.1627310922,-9.05621942074));
#63476=CARTESIAN_POINT('Ctrl Pts',(-2.06436433537,-38.2372244929,-9.12942216681));
#63477=CARTESIAN_POINT('Ctrl Pts',(-2.08149565721,-38.2742355501,-9.22210406029));
#63478=CARTESIAN_POINT('Ctrl Pts',(-2.09862701806,-38.2742356128,-9.31478596379));
#63479=CARTESIAN_POINT('Ctrl Pts',(-2.03570878929,-37.9742356128,-9.02138447577));
#63480=CARTESIAN_POINT('Ctrl Pts',(-2.03570878929,-38.0684833924,-9.02138447577));
#63481=CARTESIAN_POINT('Ctrl Pts',(-2.04272147106,-38.1627311721,-9.05772515867));
#63482=CARTESIAN_POINT('Ctrl Pts',(-2.05681387623,-38.2372245951,-9.13087372673));
#63483=CARTESIAN_POINT('Ctrl Pts',(-2.07465269973,-38.2742356128,-9.22341819256));
#63484=CARTESIAN_POINT('Ctrl Pts',(-2.09249152102,-38.2742356128,-9.31596265782));
#63485=CARTESIAN_POINT('Ctrl Pts',(-2.02820898726,-37.9742356128,-9.02284995699));
#63486=CARTESIAN_POINT('Ctrl Pts',(-2.02820898726,-38.0684833924,-9.02284995699));
#63487=CARTESIAN_POINT('Ctrl Pts',(-2.03530680234,-38.1627311721,-9.05917400362));
#63488=CARTESIAN_POINT('Ctrl Pts',(-2.04959283393,-38.2372245963,-9.13228473856));
#63489=CARTESIAN_POINT('Ctrl Pts',(-2.06766727163,-38.2742356128,-9.22478316375));
#63490=CARTESIAN_POINT('Ctrl Pts',(-2.08574170933,-38.2742356128,-9.31728158894));
#63491=CARTESIAN_POINT('',(-2.02820898726,-37.9742356128,-9.02284995699));
#63492=CARTESIAN_POINT('Origin',(-2.08533572939304,-37.9763569039443,-9.3151995089407));
#63493=CARTESIAN_POINT('',(-2.06576130603488,-37.9742356128,-9.01576016653796));
#63494=CARTESIAN_POINT('Origin',(-2.46533597282467,-37.9742356128,-11.2350939774593));
#63495=CARTESIAN_POINT('Origin',(-2.11915381796855,-37.9763566360376,-9.30881475751182));
#63496=CARTESIAN_POINT('Origin',(-2.60353950403013,-37.9742356128,-11.9671837342904));
#63497=CARTESIAN_POINT('',(-2.02820898725,-37.2742356128,-9.02284995699));
#63498=CARTESIAN_POINT('',(-2.06575948168,-37.2742356128,-9.01576047707));
#63499=CARTESIAN_POINT('Ctrl Pts',(-2.11953749589,-36.2742356128,-9.31090098978));
#63500=CARTESIAN_POINT('Ctrl Pts',(-2.10264256193,-36.2742356128,-9.21817987482));
#63501=CARTESIAN_POINT('Ctrl Pts',(-2.08574762796,-36.3112466293,-9.12545875985));
#63502=CARTESIAN_POINT('Ctrl Pts',(-2.07239387587,-36.3857400536,-9.05217201097));
#63503=CARTESIAN_POINT('Ctrl Pts',(-2.06575925082,-36.4799878332,-9.01576051427));
#63504=CARTESIAN_POINT('Ctrl Pts',(-2.06575925082,-36.5742356128,-9.01576051427));
#63505=CARTESIAN_POINT('Ctrl Pts',(-2.61883842747,-36.2742356128,-9.21992235908));
#63506=CARTESIAN_POINT('Ctrl Pts',(-2.59793617609,-36.2742356128,-9.12793143196));
#63507=CARTESIAN_POINT('Ctrl Pts',(-2.57703392472,-36.3112466293,-9.03594050483));
#63508=CARTESIAN_POINT('Ctrl Pts',(-2.56051279612,-36.3857400536,-8.96323089513));
#63509=CARTESIAN_POINT('Ctrl Pts',(-2.5523044949,-36.4799878332,-8.92710614364));
#63510=CARTESIAN_POINT('Ctrl Pts',(-2.5523044949,-36.5742356128,-8.92710614364));
#63511=CARTESIAN_POINT('Ctrl Pts',(-3.11244995705,-36.2742356128,-9.10225947341));
#63512=CARTESIAN_POINT('Ctrl Pts',(-3.08747265848,-36.2742356128,-9.0112321755));
#63513=CARTESIAN_POINT('Ctrl Pts',(-3.06249535992,-36.3112466293,-8.92020487759));
#63514=CARTESIAN_POINT('Ctrl Pts',(-3.0427532992,-36.3857400536,-8.84825692301));
#63515=CARTESIAN_POINT('Ctrl Pts',(-3.03294474641,-36.4799878332,-8.81251058504));
#63516=CARTESIAN_POINT('Ctrl Pts',(-3.03294474641,-36.5742356128,-8.81251058504));
#63517=CARTESIAN_POINT('Ctrl Pts',(-3.59670238728,-36.2742356128,-8.9571409937));
#63518=CARTESIAN_POINT('Ctrl Pts',(-3.56742906565,-36.2742356128,-8.86737676632));
#63519=CARTESIAN_POINT('Ctrl Pts',(-3.53815574401,-36.3112466293,-8.77761253894));
#63520=CARTESIAN_POINT('Ctrl Pts',(-3.5150181194,-36.3857400536,-8.70666291293));
#63521=CARTESIAN_POINT('Ctrl Pts',(-3.50352251051,-36.4799878332,-8.6714125837));
#63522=CARTESIAN_POINT('Ctrl Pts',(-3.50352251051,-36.5742356128,-8.6714125837));
#63523=CARTESIAN_POINT('Ctrl Pts',(-4.71225848168,-36.2742356128,-8.54787678002));
#63524=CARTESIAN_POINT('Ctrl Pts',(-4.67300397879,-36.2742356128,-8.46179505057));
#63525=CARTESIAN_POINT('Ctrl Pts',(-4.6337494759,-36.3112466293,-8.37571332112));
#63526=CARTESIAN_POINT('Ctrl Pts',(-4.60272272226,-36.3857400536,-8.30767434165));
#63527=CARTESIAN_POINT('Ctrl Pts',(-4.58730751821,-36.4799878332,-8.27387012499));
#63528=CARTESIAN_POINT('Ctrl Pts',(-4.58730751821,-36.5742356128,-8.27387012499));
#63529=CARTESIAN_POINT('Ctrl Pts',(-5.76024912723,-36.2742356128,-7.98940147532));
#63530=CARTESIAN_POINT('Ctrl Pts',(-5.71191143403,-36.2742356128,-7.90816087535));
#63531=CARTESIAN_POINT('Ctrl Pts',(-5.66357374084,-36.3112466293,-7.82692027539));
#63532=CARTESIAN_POINT('Ctrl Pts',(-5.62536764306,-36.3857400536,-7.76270772231));
#63533=CARTESIAN_POINT('Ctrl Pts',(-5.60638547104,-36.4799878332,-7.73080461404));
#63534=CARTESIAN_POINT('Ctrl Pts',(-5.60638547104,-36.5742356128,-7.73080461404));
#63535=CARTESIAN_POINT('Ctrl Pts',(-6.33821543401,-36.2742356128,-7.61896694326));
#63536=CARTESIAN_POINT('Ctrl Pts',(-6.28525641384,-36.2742356128,-7.54080551103));
#63537=CARTESIAN_POINT('Ctrl Pts',(-6.23229739367,-36.3112466293,-7.46264407879));
#63538=CARTESIAN_POINT('Ctrl Pts',(-6.1904385957,-36.3857400536,-7.40086530005));
#63539=CARTESIAN_POINT('Ctrl Pts',(-6.16964163719,-36.4799878332,-7.37017137728));
#63540=CARTESIAN_POINT('Ctrl Pts',(-6.16964163719,-36.5742356128,-7.37017137728));
#63541=CARTESIAN_POINT('Ctrl Pts',(-7.2863768604,-36.2742356128,-6.92663027622));
#63542=CARTESIAN_POINT('Ctrl Pts',(-7.2271227297,-36.2742356128,-6.8530659898));
#63543=CARTESIAN_POINT('Ctrl Pts',(-7.167868599,-36.3112466293,-6.77950170338));
#63544=CARTESIAN_POINT('Ctrl Pts',(-7.12103414712,-36.3857400536,-6.72135650754));
#63545=CARTESIAN_POINT('Ctrl Pts',(-7.0977651044,-36.4799878332,-6.69246787984));
#63546=CARTESIAN_POINT('Ctrl Pts',(-7.0977651044,-36.5742356128,-6.69246787984));
#63547=CARTESIAN_POINT('Ctrl Pts',(-8.17808008644,-36.2742356128,-6.11829341209));
#63548=CARTESIAN_POINT('Ctrl Pts',(-8.11276510867,-36.2742356128,-6.05021218498));
#63549=CARTESIAN_POINT('Ctrl Pts',(-8.0474501309,-36.3112466293,-5.98213095786));
#63550=CARTESIAN_POINT('Ctrl Pts',(-7.99582518686,-36.3857400536,-5.9283195709));
#63551=CARTESIAN_POINT('Ctrl Pts',(-7.97017605504,-36.4799878332,-5.90158413555));
#63552=CARTESIAN_POINT('Ctrl Pts',(-7.97017605504,-36.5742356128,-5.90158413555));
#63553=CARTESIAN_POINT('Ctrl Pts',(-8.53884026615,-36.2742356128,-5.7594573392));
#63554=CARTESIAN_POINT('Ctrl Pts',(-8.47082512858,-36.2742356128,-5.69401108691));
#63555=CARTESIAN_POINT('Ctrl Pts',(-8.402809991,-36.3112466293,-5.62856483461));
#63556=CARTESIAN_POINT('Ctrl Pts',(-8.34905084127,-36.3857400536,-5.57683613125));
#63557=CARTESIAN_POINT('Ctrl Pts',(-8.32234135915,-36.4799878332,-5.55113544801));
#63558=CARTESIAN_POINT('Ctrl Pts',(-8.32234135915,-36.5742356128,-5.55113544801));
#63559=CARTESIAN_POINT('Ctrl Pts',(-9.14391387257,-36.2742356128,-5.08624796937));
#63560=CARTESIAN_POINT('Ctrl Pts',(-9.07021258959,-36.2742356128,-5.02690763905));
#63561=CARTESIAN_POINT('Ctrl Pts',(-8.99651130661,-36.3112466293,-4.96756730873));
#63562=CARTESIAN_POINT('Ctrl Pts',(-8.93825782872,-36.3857400536,-4.92066472472));
#63563=CARTESIAN_POINT('Ctrl Pts',(-8.9093154026,-36.4799878332,-4.89736183147));
#63564=CARTESIAN_POINT('Ctrl Pts',(-8.9093154026,-36.5742356128,-4.89736183147));
#63565=CARTESIAN_POINT('Ctrl Pts',(-9.65506365996,-36.2742356128,-4.33036740431));
#63566=CARTESIAN_POINT('Ctrl Pts',(-9.57455339335,-36.2742356128,-4.28091564854));
#63567=CARTESIAN_POINT('Ctrl Pts',(-9.49404312674,-36.3112466293,-4.23146389278));
#63568=CARTESIAN_POINT('Ctrl Pts',(-9.43040782971,-36.3857400536,-4.19237723581));
#63569=CARTESIAN_POINT('Ctrl Pts',(-9.39879152194,-36.4799878332,-4.17295757681));
#63570=CARTESIAN_POINT('Ctrl Pts',(-9.39879152194,-36.5742356128,-4.17295757681));
#63571=CARTESIAN_POINT('Ctrl Pts',(-9.85393064124,-36.2742356128,-3.98362416377));
#63572=CARTESIAN_POINT('Ctrl Pts',(-9.77024228393,-36.2742356128,-3.93958894582));
#63573=CARTESIAN_POINT('Ctrl Pts',(-9.68655392663,-36.3112466293,-3.89555372787));
#63574=CARTESIAN_POINT('Ctrl Pts',(-9.62040666759,-36.3857400536,-3.86074830211));
#63575=CARTESIAN_POINT('Ctrl Pts',(-9.58754232635,-36.4799878332,-3.84345571163));
#63576=CARTESIAN_POINT('Ctrl Pts',(-9.58754232635,-36.5742356128,-3.84345571163));
#63577=CARTESIAN_POINT('Ctrl Pts',(-10.363444524,-36.2742356128,-2.88078522158));
#63578=CARTESIAN_POINT('Ctrl Pts',(-10.2712984823,-36.2742356128,-2.85484986236));
#63579=CARTESIAN_POINT('Ctrl Pts',(-10.1791524407,-36.3112466293,-2.82891450314));
#63580=CARTESIAN_POINT('Ctrl Pts',(-10.1063202294,-36.3857400536,-2.80841519904));
#63581=CARTESIAN_POINT('Ctrl Pts',(-10.0701345637,-36.4799878332,-2.79823040916));
#63582=CARTESIAN_POINT('Ctrl Pts',(-10.0701345637,-36.5742356128,-2.79823040916));
#63583=CARTESIAN_POINT('Ctrl Pts',(-10.5676336782,-36.2742356128,-1.65939737822));
#63584=CARTESIAN_POINT('Ctrl Pts',(-10.4719619497,-36.2742356128,-1.65453645426));
#63585=CARTESIAN_POINT('Ctrl Pts',(-10.3762902212,-36.3112466293,-1.64967553031));
#63586=CARTESIAN_POINT('Ctrl Pts',(-10.3006713084,-36.3857400536,-1.64583346123));
#63587=CARTESIAN_POINT('Ctrl Pts',(-10.2631011081,-36.4799878332,-1.64392457671));
#63588=CARTESIAN_POINT('Ctrl Pts',(-10.2631011081,-36.5742356128,-1.64392457671));
#63589=CARTESIAN_POINT('Ctrl Pts',(-10.5419165386,-36.2742356128,-0.848067876402));
#63590=CARTESIAN_POINT('Ctrl Pts',(-10.4477463127,-36.2742356128,-0.852679034501));
#63591=CARTESIAN_POINT('Ctrl Pts',(-10.3535760868,-36.3112466293,-0.8572901926));
#63592=CARTESIAN_POINT('Ctrl Pts',(-10.2791439585,-36.3857400536,-0.860934836052));
#63593=CARTESIAN_POINT('Ctrl Pts',(-10.2421633997,-36.4799878332,-0.862745648498));
#63594=CARTESIAN_POINT('Ctrl Pts',(-10.2421633997,-36.5742356128,-0.862745648498));
#63595=CARTESIAN_POINT('Ctrl Pts',(-10.473089026,-36.2742356128,-0.0706759998857));
#63596=CARTESIAN_POINT('Ctrl Pts',(-10.3792034004,-36.2742356128,-0.080327881531));
#63597=CARTESIAN_POINT('Ctrl Pts',(-10.2853177749,-36.3112466293,-0.0899797631762));
#63598=CARTESIAN_POINT('Ctrl Pts',(-10.2111105988,-36.3857400536,-0.0976086182963));
#63599=CARTESIAN_POINT('Ctrl Pts',(-10.1742417982,-36.4799878332,-0.101398893365));
#63600=CARTESIAN_POINT('Ctrl Pts',(-10.1742417982,-36.5742356128,-0.101398893365));
#63601=CARTESIAN_POINT('Ctrl Pts',(-10.3535104648,-36.2742356128,0.692257829523));
#63602=CARTESIAN_POINT('Ctrl Pts',(-10.2603995032,-36.2742356128,0.67766355641));
#63603=CARTESIAN_POINT('Ctrl Pts',(-10.1672885415,-36.3112466293,0.663069283296));
#63604=CARTESIAN_POINT('Ctrl Pts',(-10.0936936579,-36.3857400536,0.651533973036));
#63605=CARTESIAN_POINT('Ctrl Pts',(-10.0571290687,-36.4799878332,0.645802815386));
#63606=CARTESIAN_POINT('Ctrl Pts',(-10.0571290687,-36.5742356128,0.645802815386));
#63607=CARTESIAN_POINT('',(-10.0571285787,-36.5742356128,0.645805825719));
#63608=CARTESIAN_POINT('Origin',(-10.3514149258478,-36.5721143559387,0.691928460092334));
#63609=CARTESIAN_POINT('Ctrl Pts',(-2.06575948168,-36.5742356128,-9.01576047707));
#63610=CARTESIAN_POINT('Ctrl Pts',(-2.88684751198,-36.5742356128,-8.86614972783));
#63611=CARTESIAN_POINT('Ctrl Pts',(-3.69023581935,-36.5742356128,-8.64282630111));
#63612=CARTESIAN_POINT('Ctrl Pts',(-4.45617471096,-36.5742356128,-8.3426574972));
#63613=CARTESIAN_POINT('Ctrl Pts',(-5.4347519266,-36.5742356128,-7.8381799988));
#63614=CARTESIAN_POINT('Ctrl Pts',(-6.34892734604,-36.5742356128,-7.22182745264));
#63615=CARTESIAN_POINT('Ctrl Pts',(-6.57301164304,-36.5742356128,-7.06148474597));
#63616=CARTESIAN_POINT('Ctrl Pts',(-7.23577044161,-36.5742356128,-6.56118503754));
#63617=CARTESIAN_POINT('Ctrl Pts',(-7.87223833418,-36.5742356128,-6.00004951347));
#63618=CARTESIAN_POINT('Ctrl Pts',(-8.28331893233,-36.5742356128,-5.59939000156));
#63619=CARTESIAN_POINT('Ctrl Pts',(-8.90941365274,-36.5742356128,-4.90631405862));
#63620=CARTESIAN_POINT('Ctrl Pts',(-9.42196991537,-36.5742356128,-4.13127436126));
#63621=CARTESIAN_POINT('Ctrl Pts',(-9.59767693443,-36.5742356128,-3.81973064431));
#63622=CARTESIAN_POINT('Ctrl Pts',(-9.84427307953,-36.5742356128,-3.28258152507));
#63623=CARTESIAN_POINT('Ctrl Pts',(-10.0147288891,-36.5742356128,-2.71679407199));
#63624=CARTESIAN_POINT('Ctrl Pts',(-10.0694270847,-36.5742356128,-2.49123410795));
#63625=CARTESIAN_POINT('Ctrl Pts',(-10.154755688,-36.5742356128,-2.03576280704));
#63626=CARTESIAN_POINT('Ctrl Pts',(-10.1959693718,-36.5742356128,-1.57549366979));
#63627=CARTESIAN_POINT('Ctrl Pts',(-10.2066163947,-36.5742356128,-1.34483444272));
#63628=CARTESIAN_POINT('Ctrl Pts',(-10.2113958308,-36.5742356128,-0.80319628916));
#63629=CARTESIAN_POINT('Ctrl Pts',(-10.1751569467,-36.5742356128,-0.265526349602));
#63630=CARTESIAN_POINT('Ctrl Pts',(-10.1436911823,-36.5742356128,0.0415756246997));
#63631=CARTESIAN_POINT('Ctrl Pts',(-10.1043144812,-36.5742356128,0.344751093937));
#63632=CARTESIAN_POINT('Ctrl Pts',(-10.0571285787,-36.5742356128,0.645805825719));
#63633=CARTESIAN_POINT('Ctrl Pts',(-10.0571285552,-37.9742356128,0.645805969836));
#63634=CARTESIAN_POINT('Ctrl Pts',(-10.0571285554,-38.0684833925,0.645805968571));
#63635=CARTESIAN_POINT('Ctrl Pts',(-10.0936931762,-38.1627311721,0.651536924187));
#63636=CARTESIAN_POINT('Ctrl Pts',(-10.1672881231,-38.2372245963,0.663071829355));
#63637=CARTESIAN_POINT('Ctrl Pts',(-10.2603991649,-38.2742356128,0.67766559072));
#63638=CARTESIAN_POINT('Ctrl Pts',(-10.3535102065,-38.2742356128,0.692259352582));
#63639=CARTESIAN_POINT('Ctrl Pts',(-10.166801105,-37.9742356128,-0.0539288837089));
#63640=CARTESIAN_POINT('Ctrl Pts',(-10.1668011785,-38.0684833943,-0.0539293520197));
#63641=CARTESIAN_POINT('Ctrl Pts',(-10.2036480968,-38.1627311757,-0.0499995227518));
#63642=CARTESIAN_POINT('Ctrl Pts',(-10.2778111132,-38.2372246007,-0.0420890384201));
#63643=CARTESIAN_POINT('Ctrl Pts',(-10.3716408342,-38.2742356157,-0.0320806300088));
#63644=CARTESIAN_POINT('Ctrl Pts',(-10.4654705253,-38.2742356128,-0.0220720388979));
#63645=CARTESIAN_POINT('Ctrl Pts',(-10.233499836,-37.9742356128,-0.766569459386));
#63646=CARTESIAN_POINT('Ctrl Pts',(-10.2334997254,-38.0684833762,-0.766568752312));
#63647=CARTESIAN_POINT('Ctrl Pts',(-10.2704792366,-38.1627311396,-0.764558608417));
#63648=CARTESIAN_POINT('Ctrl Pts',(-10.3449094314,-38.2372245581,-0.760513883966));
#63649=CARTESIAN_POINT('Ctrl Pts',(-10.4390772685,-38.2742355874,-0.755396874269));
#63650=CARTESIAN_POINT('Ctrl Pts',(-10.5332451587,-38.2742356128,-0.750280139627));
#63651=CARTESIAN_POINT('Ctrl Pts',(-10.2589747967,-37.9742356128,-1.49377249196));
#63652=CARTESIAN_POINT('Ctrl Pts',(-10.2589748319,-38.0684834037,-1.49377265296));
#63653=CARTESIAN_POINT('Ctrl Pts',(-10.2963782615,-38.1627311946,-1.49497949399));
#63654=CARTESIAN_POINT('Ctrl Pts',(-10.3716614552,-38.2372246229,-1.49740827406));
#63655=CARTESIAN_POINT('Ctrl Pts',(-10.4669084166,-38.2742356306,-1.50048105645));
#63656=CARTESIAN_POINT('Ctrl Pts',(-10.5621553577,-38.2742356128,-1.5035537741));
#63657=CARTESIAN_POINT('Ctrl Pts',(-10.07136584,-37.9742356128,-2.91801448478));
#63658=CARTESIAN_POINT('Ctrl Pts',(-10.0713658062,-38.0684833816,-2.91801433022));
#63659=CARTESIAN_POINT('Ctrl Pts',(-10.1076744141,-38.1627311504,-2.92880207761));
#63660=CARTESIAN_POINT('Ctrl Pts',(-10.1807541274,-38.2372245708,-2.95051523186));
#63661=CARTESIAN_POINT('Ctrl Pts',(-10.2732133244,-38.2742355958,-2.97798640082));
#63662=CARTESIAN_POINT('Ctrl Pts',(-10.3656725408,-38.2742356128,-3.00545763192));
#63663=CARTESIAN_POINT('Ctrl Pts',(-9.43888580477,-37.9742356128,-4.19731493645));
#63664=CARTESIAN_POINT('Ctrl Pts',(-9.43888583723,-38.0684834029,-4.19731508481));
#63665=CARTESIAN_POINT('Ctrl Pts',(-9.47062176951,-38.1627311929,-4.21722149235));
#63666=CARTESIAN_POINT('Ctrl Pts',(-9.53449778852,-38.2372246208,-4.2572875957));
#63667=CARTESIAN_POINT('Ctrl Pts',(-9.61531259337,-38.2742356292,-4.30797846695));
#63668=CARTESIAN_POINT('Ctrl Pts',(-9.6961273796,-38.2742356128,-4.35866927856));
#63669=CARTESIAN_POINT('Ctrl Pts',(-9.02777291595,-37.9742356128,-4.76329520136));
#63670=CARTESIAN_POINT('Ctrl Pts',(-9.02777292761,-38.0684834,-4.76329519358));
#63671=CARTESIAN_POINT('Ctrl Pts',(-9.057065221,-38.1627311872,-4.78613151867));
#63672=CARTESIAN_POINT('Ctrl Pts',(-9.11602287492,-38.2372246142,-4.83209503424));
#63673=CARTESIAN_POINT('Ctrl Pts',(-9.19061506035,-38.2742356247,-4.89024727341));
#63674=CARTESIAN_POINT('Ctrl Pts',(-9.26520723838,-38.2742356128,-4.94839951173));
#63675=CARTESIAN_POINT('Ctrl Pts',(-8.30376468439,-37.9742356128,-5.59440760207));
#63676=CARTESIAN_POINT('Ctrl Pts',(-8.30376467773,-38.0684833881,-5.59440760651));
#63677=CARTESIAN_POINT('Ctrl Pts',(-8.33036893671,-38.1627311634,-5.62029070861));
#63678=CARTESIAN_POINT('Ctrl Pts',(-8.38391630832,-38.2372245861,-5.67238656763));
#63679=CARTESIAN_POINT('Ctrl Pts',(-8.45166351292,-38.274235606,-5.7382973376));
#63680=CARTESIAN_POINT('Ctrl Pts',(-8.51941072175,-38.2742356128,-5.80420810805));
#63681=CARTESIAN_POINT('Ctrl Pts',(-7.49360195673,-37.9742356128,-6.33060530722));
#63682=CARTESIAN_POINT('Ctrl Pts',(-7.49360196054,-38.0684833949,-6.33060530468));
#63683=CARTESIAN_POINT('Ctrl Pts',(-7.51791854842,-38.162731177,-6.35853121169));
#63684=CARTESIAN_POINT('Ctrl Pts',(-7.5668614281,-38.2372246022,-6.41473870745));
#63685=CARTESIAN_POINT('Ctrl Pts',(-7.62878310191,-38.2742356167,-6.48585145033));
#63686=CARTESIAN_POINT('Ctrl Pts',(-7.6907047733,-38.2742356128,-6.55696419293));
#63687=CARTESIAN_POINT('Ctrl Pts',(-7.19158531474,-37.9742356128,-6.58638782253));
#63688=CARTESIAN_POINT('Ctrl Pts',(-7.19158531103,-38.0684833899,-6.58638782576));
#63689=CARTESIAN_POINT('Ctrl Pts',(-7.21512703478,-38.162731167,-6.61497407193));
#63690=CARTESIAN_POINT('Ctrl Pts',(-7.26251032621,-38.2372245904,-6.67251064937));
#63691=CARTESIAN_POINT('Ctrl Pts',(-7.32245884208,-38.2742356089,-6.74530492126));
#63692=CARTESIAN_POINT('Ctrl Pts',(-7.38240736043,-38.2742356128,-6.81809919304));
#63693=CARTESIAN_POINT('Ctrl Pts',(-6.57881164637,-37.9742356128,-7.06987433056));
#63694=CARTESIAN_POINT('Ctrl Pts',(-6.57881165007,-38.068483395,-7.06987432735));
#63695=CARTESIAN_POINT('Ctrl Pts',(-6.60071832324,-38.1627311771,-7.09975694193));
#63696=CARTESIAN_POINT('Ctrl Pts',(-6.64481067968,-38.2372246022,-7.15990277537));
#63697=CARTESIAN_POINT('Ctrl Pts',(-6.7005955562,-38.2742356168,-7.23599823476));
#63698=CARTESIAN_POINT('Ctrl Pts',(-6.75638043023,-38.2742356128,-7.31209369426));
#63699=CARTESIAN_POINT('Ctrl Pts',(-5.9353899124,-37.9742356128,-7.5039276571));
#63700=CARTESIAN_POINT('Ctrl Pts',(-5.93538990872,-38.06848339,-7.5039276603));
#63701=CARTESIAN_POINT('Ctrl Pts',(-5.95536133185,-38.1627311671,-7.53512169599));
#63702=CARTESIAN_POINT('Ctrl Pts',(-5.99555854896,-38.2372245905,-7.5979070666));
#63703=CARTESIAN_POINT('Ctrl Pts',(-6.046415369,-38.2742356089,-7.67734202));
#63704=CARTESIAN_POINT('Ctrl Pts',(-6.09727219151,-38.2742356128,-7.75677697329));
#63705=CARTESIAN_POINT('Ctrl Pts',(-5.60614917144,-37.9742356128,-7.70722191498));
#63706=CARTESIAN_POINT('Ctrl Pts',(-5.60614918073,-38.0684833903,-7.707221912));
#63707=CARTESIAN_POINT('Ctrl Pts',(-5.6250617684,-38.1627311678,-7.73907597951));
#63708=CARTESIAN_POINT('Ctrl Pts',(-5.6631278099,-38.2372245913,-7.80318982834));
#63709=CARTESIAN_POINT('Ctrl Pts',(-5.71128829675,-38.2742356095,-7.88430555277));
#63710=CARTESIAN_POINT('Ctrl Pts',(-5.75944878038,-38.2742356128,-7.96542127963));
#63711=CARTESIAN_POINT('Ctrl Pts',(-4.74244689379,-37.9742356128,-8.18975922749));
#63712=CARTESIAN_POINT('Ctrl Pts',(-4.74244687927,-38.0684833958,-8.18975923215));
#63713=CARTESIAN_POINT('Ctrl Pts',(-4.75843542755,-38.1627311787,-8.22325041568));
#63714=CARTESIAN_POINT('Ctrl Pts',(-4.79061618477,-38.2372246042,-8.29065933715));
#63715=CARTESIAN_POINT('Ctrl Pts',(-4.83133072336,-38.2742356181,-8.37594392375));
#63716=CARTESIAN_POINT('Ctrl Pts',(-4.87204526698,-38.2742356128,-8.46122850655));
#63717=CARTESIAN_POINT('Ctrl Pts',(-3.8297049454,-37.9742356128,-8.56858316919));
#63718=CARTESIAN_POINT('Ctrl Pts',(-3.8297049681,-38.0684833872,-8.5685831619));
#63719=CARTESIAN_POINT('Ctrl Pts',(-3.84237809363,-38.1627311616,-8.60346422097));
#63720=CARTESIAN_POINT('Ctrl Pts',(-3.86788572113,-38.237224584,-8.67367061231));
#63721=CARTESIAN_POINT('Ctrl Pts',(-3.90015751593,-38.2742356046,-8.76249451857));
#63722=CARTESIAN_POINT('Ctrl Pts',(-3.93242930286,-38.2742356128,-8.85131843076));
#63723=CARTESIAN_POINT('Ctrl Pts',(-3.25582231846,-37.9742356128,-8.75788647545));
#63724=CARTESIAN_POINT('Ctrl Pts',(-3.25582230332,-38.0684834022,-8.75788647812));
#63725=CARTESIAN_POINT('Ctrl Pts',(-3.2663841251,-38.1627311915,-8.79345058999));
#63726=CARTESIAN_POINT('Ctrl Pts',(-3.28764233655,-38.2372246192,-8.86503176831));
#63727=CARTESIAN_POINT('Ctrl Pts',(-3.31453785051,-38.2742356281,-8.95559502193));
#63728=CARTESIAN_POINT('Ctrl Pts',(-3.34143336856,-38.2742356128,-9.04615826881));
#63729=CARTESIAN_POINT('Ctrl Pts',(-2.66537560342,-37.9742356128,-8.90650444612));
#63730=CARTESIAN_POINT('Ctrl Pts',(-2.66537564264,-38.0684833929,-8.90650443911));
#63731=CARTESIAN_POINT('Ctrl Pts',(-2.67394959074,-38.1627311729,-8.94256257595));
#63732=CARTESIAN_POINT('Ctrl Pts',(-2.69120662213,-38.2372245974,-9.0151381165));
#63733=CARTESIAN_POINT('Ctrl Pts',(-2.71303990103,-38.2742356135,-9.10695942575));
#63734=CARTESIAN_POINT('Ctrl Pts',(-2.73487316451,-38.2742356128,-9.19878073748));
#63735=CARTESIAN_POINT('Ctrl Pts',(-2.0657631474,-37.9742356128,-9.01575989378));
#63736=CARTESIAN_POINT('Ctrl Pts',(-2.06576314406,-38.0684833924,-9.01575989438));
#63737=CARTESIAN_POINT('Ctrl Pts',(-2.07239767256,-38.162731172,-9.05217140948));
#63738=CARTESIAN_POINT('Ctrl Pts',(-2.08575123441,-38.2372245963,-9.12545819469));
#63739=CARTESIAN_POINT('Ctrl Pts',(-2.10264592972,-38.2742356128,-9.21817935525));
#63740=CARTESIAN_POINT('Ctrl Pts',(-2.11954062634,-38.2742356128,-9.3109005156));
#63741=CARTESIAN_POINT('',(-10.0571285787,-37.9742356128,0.645805825719));
#63742=CARTESIAN_POINT('Ctrl Pts',(-2.0657631474,-37.9742356128,-9.01575989378));
#63743=CARTESIAN_POINT('Ctrl Pts',(-2.21055756124637,-37.9742356128,-8.98937688864956));
#63744=CARTESIAN_POINT('Ctrl Pts',(-2.35470583880119,-37.9742356128,-8.96023914137939));
#63745=CARTESIAN_POINT('Ctrl Pts',(-2.49801140128497,-37.9742356128,-8.92830835678781));
#63746=CARTESIAN_POINT('Ctrl Pts',(-2.64661454196291,-37.9742356128,-8.89519718655563));
#63747=CARTESIAN_POINT('Ctrl Pts',(-2.7943118638327,-37.9742356128,-8.85908222926721));
#63748=CARTESIAN_POINT('Ctrl Pts',(-2.94094133902924,-37.9742356128,-8.81992924536183));
#63749=CARTESIAN_POINT('Ctrl Pts',(-3.09326087237576,-37.9742356128,-8.77925690284954));
#63750=CARTESIAN_POINT('Ctrl Pts',(-3.24442857386082,-37.9742356128,-8.73530560793822));
#63751=CARTESIAN_POINT('Ctrl Pts',(-3.39431677839277,-37.9742356128,-8.6880537429529));
#63752=CARTESIAN_POINT('Ctrl Pts',(-3.55149447503361,-37.9742356128,-8.6385038846197));
#63753=CARTESIAN_POINT('Ctrl Pts',(-3.70726586213417,-37.9742356128,-8.58532381792461));
#63754=CARTESIAN_POINT('Ctrl Pts',(-3.86153295951299,-37.9742356128,-8.52851746693305));
#63755=CARTESIAN_POINT('Ctrl Pts',(-4.0172550578266,-37.9742356128,-8.47117533549836));
#63756=CARTESIAN_POINT('Ctrl Pts',(-4.17144546130456,-37.9742356128,-8.41013749149708));
#63757=CARTESIAN_POINT('Ctrl Pts',(-4.32403828257966,-37.9742356128,-8.34544797793615));
#63758=CARTESIAN_POINT('Ctrl Pts',(-4.47348519624443,-37.9742356128,-8.28209212628224));
#63759=CARTESIAN_POINT('Ctrl Pts',(-4.62140087163535,-37.9742356128,-8.21523318084772));
#63760=CARTESIAN_POINT('Ctrl Pts',(-4.76773975955357,-37.9742356128,-8.1449588479227));
#63761=CARTESIAN_POINT('Ctrl Pts',(-4.82030561847545,-37.9742356128,-8.11971586075151));
#63762=CARTESIAN_POINT('Ctrl Pts',(-4.87266809902291,-37.9742356128,-8.0940326613706));
#63763=CARTESIAN_POINT('Ctrl Pts',(-4.92482519221318,-37.9742356128,-8.06791498369728));
#63764=CARTESIAN_POINT('Ctrl Pts',(-5.06040908297022,-37.9742356128,-8.00002131593537));
#63765=CARTESIAN_POINT('Ctrl Pts',(-5.19460591643175,-37.9742356128,-7.92918756170566));
#63766=CARTESIAN_POINT('Ctrl Pts',(-5.32737904492262,-37.9742356128,-7.85553870103708));
#63767=CARTESIAN_POINT('Ctrl Pts',(-5.48706475962,-37.9742356128,-7.76696150860226));
#63768=CARTESIAN_POINT('Ctrl Pts',(-5.64468815179341,-37.9742356128,-7.67431398917331));
#63769=CARTESIAN_POINT('Ctrl Pts',(-5.80019139110691,-37.9742356128,-7.57788422162767));
#63770=CARTESIAN_POINT('Ctrl Pts',(-5.9314757506791,-37.9742356128,-7.49647292542694));
#63771=CARTESIAN_POINT('Ctrl Pts',(-6.06124785245264,-37.9742356128,-7.41236864383582));
#63772=CARTESIAN_POINT('Ctrl Pts',(-6.18950386976392,-37.9742356128,-7.32575186448882));
#63773=CARTESIAN_POINT('Ctrl Pts',(-6.3059579274687,-37.9742356128,-7.24710545372591));
#63774=CARTESIAN_POINT('Ctrl Pts',(-6.42116159360231,-37.9742356128,-7.16638882252908));
#63775=CARTESIAN_POINT('Ctrl Pts',(-6.53514946295618,-37.9742356128,-7.08371932032296));
#63776=CARTESIAN_POINT('Ctrl Pts',(-6.54670148833218,-37.9742356128,-7.07534123419221));
#63777=CARTESIAN_POINT('Ctrl Pts',(-6.55824106452687,-37.9742356128,-7.06694306644521));
#63778=CARTESIAN_POINT('Ctrl Pts',(-6.56976825429465,-37.9742356128,-7.05852492131865));
#63779=CARTESIAN_POINT('Ctrl Pts',(-6.64878179524979,-37.9742356128,-7.00082243978382));
#63780=CARTESIAN_POINT('Ctrl Pts',(-6.72721753878092,-37.9742356128,-6.94217924661947));
#63781=CARTESIAN_POINT('Ctrl Pts',(-6.80514089959812,-37.9742356128,-6.88257070926825));
#63782=CARTESIAN_POINT('Ctrl Pts',(-6.88589195492991,-37.9742356128,-6.82079908844215));
#63783=CARTESIAN_POINT('Ctrl Pts',(-6.96609266210244,-37.9742356128,-6.75799124102026));
#63784=CARTESIAN_POINT('Ctrl Pts',(-7.0457631144731,-37.9742356128,-6.69414250228203));
#63785=CARTESIAN_POINT('Ctrl Pts',(-7.12865126771334,-37.9742356128,-6.62771506421366));
#63786=CARTESIAN_POINT('Ctrl Pts',(-7.21096532137975,-37.9742356128,-6.56016156130215));
#63787=CARTESIAN_POINT('Ctrl Pts',(-7.29267376299196,-37.9742356128,-6.49149273615506));
#63788=CARTESIAN_POINT('Ctrl Pts',(-7.37939561494801,-37.9742356128,-6.41861057647975));
#63789=CARTESIAN_POINT('Ctrl Pts',(-7.46543516586726,-37.9742356128,-6.34447289356002));
#63790=CARTESIAN_POINT('Ctrl Pts',(-7.55069654496993,-37.9742356128,-6.26909869682082));
#63791=CARTESIAN_POINT('Ctrl Pts',(-7.6393847665147,-37.9742356128,-6.19069504525525));
#63792=CARTESIAN_POINT('Ctrl Pts',(-7.72723055271955,-37.9742356128,-6.11095470869088));
#63793=CARTESIAN_POINT('Ctrl Pts',(-7.814069401565,-37.9742356128,-6.02988909397397));
#63794=CARTESIAN_POINT('Ctrl Pts',(-7.90090825041046,-37.9742356128,-5.94882347925705));
#63795=CARTESIAN_POINT('Ctrl Pts',(-7.98673929450905,-37.9742356128,-5.86643381460967));
#63796=CARTESIAN_POINT('Ctrl Pts',(-8.0713531761618,-37.9742356128,-5.78270311231078));
#63797=CARTESIAN_POINT('Ctrl Pts',(-8.1467028994669,-37.9742356128,-5.70813987130199));
#63798=CARTESIAN_POINT('Ctrl Pts',(-8.22108885952716,-37.9742356128,-5.63251312569528));
#63799=CARTESIAN_POINT('Ctrl Pts',(-8.29437508920965,-37.9742356128,-5.55581755269425));
#63800=CARTESIAN_POINT('Ctrl Pts',(-8.37310090860936,-37.9742356128,-5.47342933522153));
#63801=CARTESIAN_POINT('Ctrl Pts',(-8.45055738224527,-37.9742356128,-5.38980730088329));
#63802=CARTESIAN_POINT('Ctrl Pts',(-8.52652404805359,-37.9742356128,-5.30491282776207));
#63803=CARTESIAN_POINT('Ctrl Pts',(-8.61219204089014,-37.9742356128,-5.20917690151302));
#63804=CARTESIAN_POINT('Ctrl Pts',(-8.69596499022727,-37.9742356128,-5.11182198372865));
#63805=CARTESIAN_POINT('Ctrl Pts',(-8.77746802781235,-37.9742356128,-5.0127629061177));
#63806=CARTESIAN_POINT('Ctrl Pts',(-8.88365772022927,-37.9742356128,-4.88369958167865));
#63807=CARTESIAN_POINT('Ctrl Pts',(-8.98599271413021,-37.9742356128,-4.7517397333071));
#63808=CARTESIAN_POINT('Ctrl Pts',(-9.08355926863292,-37.9742356128,-4.61668045648252));
#63809=CARTESIAN_POINT('Ctrl Pts',(-9.16215290844201,-37.9742356128,-4.5078849762103));
#63810=CARTESIAN_POINT('Ctrl Pts',(-9.23764895184771,-37.9742356128,-4.39707658418915));
#63811=CARTESIAN_POINT('Ctrl Pts',(-9.30956694400941,-37.9742356128,-4.28417925211255));
#63812=CARTESIAN_POINT('Ctrl Pts',(-9.37213796405824,-37.9742356128,-4.18595485768087));
#63813=CARTESIAN_POINT('Ctrl Pts',(-9.43199962616356,-37.9742356128,-4.08614884411721));
#63814=CARTESIAN_POINT('Ctrl Pts',(-9.4888561786539,-37.9742356128,-3.984747468796));
#63815=CARTESIAN_POINT('Ctrl Pts',(-9.53965553238558,-37.9742356128,-3.89414886391758));
#63816=CARTESIAN_POINT('Ctrl Pts',(-9.58805567524611,-37.9742356128,-3.80227667672272));
#63817=CARTESIAN_POINT('Ctrl Pts',(-9.63387055719901,-37.9742356128,-3.70915455341205));
#63818=CARTESIAN_POINT('Ctrl Pts',(-9.67774260674016,-37.9742356128,-3.61998138013043));
#63819=CARTESIAN_POINT('Ctrl Pts',(-9.71924365336037,-37.9742356128,-3.5296617836214));
#63820=CARTESIAN_POINT('Ctrl Pts',(-9.75823923133626,-37.9742356128,-3.43825143381026));
#63821=CARTESIAN_POINT('Ctrl Pts',(-9.79512552212818,-37.9742356128,-3.3517855081966));
#63822=CARTESIAN_POINT('Ctrl Pts',(-9.82976990344546,-37.9742356128,-3.26434356911638));
#63823=CARTESIAN_POINT('Ctrl Pts',(-9.86208840966277,-37.9742356128,-3.17600670010489));
#63824=CARTESIAN_POINT('Ctrl Pts',(-9.89428974958264,-37.9742356128,-3.08799008425733));
#63825=CARTESIAN_POINT('Ctrl Pts',(-9.92418167132371,-37.9742356128,-2.99908468371943));
#63826=CARTESIAN_POINT('Ctrl Pts',(-9.95171582590476,-37.9742356128,-2.90940871914275));
#63827=CARTESIAN_POINT('Ctrl Pts',(-9.97851922512363,-37.9742356128,-2.82211275108205));
#63828=CARTESIAN_POINT('Ctrl Pts',(-10.0030868945867,-37.9742356128,-2.73409104825337));
#63829=CARTESIAN_POINT('Ctrl Pts',(-10.0254224159267,-37.9742356128,-2.64549978022437));
#63830=CARTESIAN_POINT('Ctrl Pts',(-10.0486642310802,-37.9742356128,-2.55331380236448));
#63831=CARTESIAN_POINT('Ctrl Pts',(-10.0694893669665,-37.9742356128,-2.46051118720013));
#63832=CARTESIAN_POINT('Ctrl Pts',(-10.087957545448,-37.9742356128,-2.36725121569743));
#63833=CARTESIAN_POINT('Ctrl Pts',(-10.1073441963928,-37.9742356128,-2.26935317358935));
#63834=CARTESIAN_POINT('Ctrl Pts',(-10.1241340090463,-37.9742356128,-2.17095128248165));
#63835=CARTESIAN_POINT('Ctrl Pts',(-10.1384510808335,-37.9742356128,-2.07221001847922));
#63836=CARTESIAN_POINT('Ctrl Pts',(-10.153674187722,-37.9742356128,-1.96722005694614));
#63837=CARTESIAN_POINT('Ctrl Pts',(-10.1661022453971,-37.9742356128,-1.86184661853482));
#63838=CARTESIAN_POINT('Ctrl Pts',(-10.1759378701588,-37.9742356128,-1.75626284034153));
#63839=CARTESIAN_POINT('Ctrl Pts',(-10.1870815562795,-37.9742356128,-1.63663724337702));
#63840=CARTESIAN_POINT('Ctrl Pts',(-10.194898157712,-37.9742356128,-1.51674233002038));
#63841=CARTESIAN_POINT('Ctrl Pts',(-10.199739349461,-37.9742356128,-1.39679152753606));
#63842=CARTESIAN_POINT('Ctrl Pts',(-10.2049385442023,-37.9742356128,-1.26797044094861));
#63843=CARTESIAN_POINT('Ctrl Pts',(-10.2067084649352,-37.9742356128,-1.13908538627714));
#63844=CARTESIAN_POINT('Ctrl Pts',(-10.2055200313416,-37.9742356128,-1.01034972448036));
#63845=CARTESIAN_POINT('Ctrl Pts',(-10.2043825812601,-37.9742356128,-0.887136791259177));
#63846=CARTESIAN_POINT('Ctrl Pts',(-10.2005378334161,-37.9742356128,-0.764060290648597));
#63847=CARTESIAN_POINT('Ctrl Pts',(-10.19439037226,-37.9742356128,-0.641263249215135));
#63848=CARTESIAN_POINT('Ctrl Pts',(-10.1889620856855,-37.9742356128,-0.53283189609585));
#63849=CARTESIAN_POINT('Ctrl Pts',(-10.1817393597794,-37.9742356128,-0.424617787571569));
#63850=CARTESIAN_POINT('Ctrl Pts',(-10.1729711247451,-37.9742356128,-0.31669226407076));
#63851=CARTESIAN_POINT('Ctrl Pts',(-10.1647993631123,-37.9742356128,-0.216108549253679));
#63852=CARTESIAN_POINT('Ctrl Pts',(-10.155285824146,-37.9742356128,-0.115775221617667));
#63853=CARTESIAN_POINT('Ctrl Pts',(-10.144593847242,-37.9742356128,-0.0157306628922133));
#63854=CARTESIAN_POINT('Ctrl Pts',(-10.134369024781,-37.9742356128,0.0799427434699424));
#63855=CARTESIAN_POINT('Ctrl Pts',(-10.1230669838381,-37.9742356128,0.175352208840096));
#63856=CARTESIAN_POINT('Ctrl Pts',(-10.1107865597769,-37.9742356128,0.27047974645221));
#63857=CARTESIAN_POINT('Ctrl Pts',(-10.099126263622,-37.9742356128,0.360803602983524));
#63858=CARTESIAN_POINT('Ctrl Pts',(-10.0865841425898,-37.9742356128,0.450873416758909));
#63859=CARTESIAN_POINT('Ctrl Pts',(-10.0731992305874,-37.9742356128,0.540686188874415));
#63860=CARTESIAN_POINT('Ctrl Pts',(-10.067971383564,-37.9742356128,0.575765047314226));
#63861=CARTESIAN_POINT('Ctrl Pts',(-10.0626144400519,-37.9742356128,0.61080482232795));
#63862=CARTESIAN_POINT('Ctrl Pts',(-10.05712857781,-37.9742356128,0.6458058255795));
#63863=CARTESIAN_POINT('Origin',(-10.3514144928172,-37.9763569061288,0.691930920254248));
#63864=CARTESIAN_POINT('Ctrl Pts',(-2.06575948168,-37.9742356128,-9.01576047707));
#63865=CARTESIAN_POINT('Ctrl Pts',(-2.06575948168,-36.2942356128,-9.01576047707));
#63866=CARTESIAN_POINT('Ctrl Pts',(-2.88684751198,-37.9742356128,-8.86614972783));
#63867=CARTESIAN_POINT('Ctrl Pts',(-2.88684751198,-36.2942356128,-8.86614972783));
#63868=CARTESIAN_POINT('Ctrl Pts',(-3.69023581935,-37.9742356128,-8.64282630111));
#63869=CARTESIAN_POINT('Ctrl Pts',(-3.69023581935,-36.2942356128,-8.64282630111));
#63870=CARTESIAN_POINT('Ctrl Pts',(-4.45617471096,-37.9742356128,-8.3426574972));
#63871=CARTESIAN_POINT('Ctrl Pts',(-4.45617471096,-36.2942356128,-8.3426574972));
#63872=CARTESIAN_POINT('Ctrl Pts',(-5.4347519266,-37.9742356128,-7.8381799988));
#63873=CARTESIAN_POINT('Ctrl Pts',(-5.4347519266,-36.2942356128,-7.8381799988));
#63874=CARTESIAN_POINT('Ctrl Pts',(-6.34892734604,-37.9742356128,-7.22182745264));
#63875=CARTESIAN_POINT('Ctrl Pts',(-6.34892734604,-36.2942356128,-7.22182745264));
#63876=CARTESIAN_POINT('Ctrl Pts',(-6.57301164304,-37.9742356128,-7.06148474597));
#63877=CARTESIAN_POINT('Ctrl Pts',(-6.57301164304,-36.2942356128,-7.06148474597));
#63878=CARTESIAN_POINT('Ctrl Pts',(-7.23577044161,-37.9742356128,-6.56118503754));
#63879=CARTESIAN_POINT('Ctrl Pts',(-7.23577044161,-36.2942356128,-6.56118503754));
#63880=CARTESIAN_POINT('Ctrl Pts',(-7.87223833418,-37.9742356128,-6.00004951347));
#63881=CARTESIAN_POINT('Ctrl Pts',(-7.87223833418,-36.2942356128,-6.00004951347));
#63882=CARTESIAN_POINT('Ctrl Pts',(-8.28331893233,-37.9742356128,-5.59939000156));
#63883=CARTESIAN_POINT('Ctrl Pts',(-8.28331893233,-36.2942356128,-5.59939000156));
#63884=CARTESIAN_POINT('Ctrl Pts',(-8.90941365274,-37.9742356128,-4.90631405862));
#63885=CARTESIAN_POINT('Ctrl Pts',(-8.90941365274,-36.2942356128,-4.90631405862));
#63886=CARTESIAN_POINT('Ctrl Pts',(-9.42196991537,-37.9742356128,-4.13127436126));
#63887=CARTESIAN_POINT('Ctrl Pts',(-9.42196991537,-36.2942356128,-4.13127436126));
#63888=CARTESIAN_POINT('Ctrl Pts',(-9.59767693443,-37.9742356128,-3.81973064431));
#63889=CARTESIAN_POINT('Ctrl Pts',(-9.59767693443,-36.2942356128,-3.81973064431));
#63890=CARTESIAN_POINT('Ctrl Pts',(-9.84427307953,-37.9742356128,-3.28258152507));
#63891=CARTESIAN_POINT('Ctrl Pts',(-9.84427307953,-36.2942356128,-3.28258152507));
#63892=CARTESIAN_POINT('Ctrl Pts',(-10.0147288891,-37.9742356128,-2.71679407199));
#63893=CARTESIAN_POINT('Ctrl Pts',(-10.0147288891,-36.2942356128,-2.71679407199));
#63894=CARTESIAN_POINT('Ctrl Pts',(-10.0694270847,-37.9742356128,-2.49123410795));
#63895=CARTESIAN_POINT('Ctrl Pts',(-10.0694270847,-36.2942356128,-2.49123410795));
#63896=CARTESIAN_POINT('Ctrl Pts',(-10.154755688,-37.9742356128,-2.03576280704));
#63897=CARTESIAN_POINT('Ctrl Pts',(-10.154755688,-36.2942356128,-2.03576280704));
#63898=CARTESIAN_POINT('Ctrl Pts',(-10.1959693718,-37.9742356128,-1.57549366979));
#63899=CARTESIAN_POINT('Ctrl Pts',(-10.1959693718,-36.2942356128,-1.57549366979));
#63900=CARTESIAN_POINT('Ctrl Pts',(-10.2066163947,-37.9742356128,-1.34483444272));
#63901=CARTESIAN_POINT('Ctrl Pts',(-10.2066163947,-36.2942356128,-1.34483444272));
#63902=CARTESIAN_POINT('Ctrl Pts',(-10.2113958308,-37.9742356128,-0.80319628916));
#63903=CARTESIAN_POINT('Ctrl Pts',(-10.2113958308,-36.2942356128,-0.80319628916));
#63904=CARTESIAN_POINT('Ctrl Pts',(-10.1751569467,-37.9742356128,-0.265526349602));
#63905=CARTESIAN_POINT('Ctrl Pts',(-10.1751569467,-36.2942356128,-0.265526349602));
#63906=CARTESIAN_POINT('Ctrl Pts',(-10.1436911823,-37.9742356128,0.0415756246997));
#63907=CARTESIAN_POINT('Ctrl Pts',(-10.1436911823,-36.2942356128,0.0415756246997));
#63908=CARTESIAN_POINT('Ctrl Pts',(-10.1043144812,-37.9742356128,0.344751093937));
#63909=CARTESIAN_POINT('Ctrl Pts',(-10.1043144812,-36.2942356128,0.344751093937));
#63910=CARTESIAN_POINT('Ctrl Pts',(-10.0571285787,-37.9742356128,0.645805825719));
#63911=CARTESIAN_POINT('Ctrl Pts',(-10.0571285787,-36.2942356128,0.645805825719));
#63912=CARTESIAN_POINT('',(-10.0571285787,-37.2742356128,0.645805825719));
#63913=CARTESIAN_POINT('Ctrl Pts',(-10.3535102174,-36.2742356128,0.692259289483));
#63914=CARTESIAN_POINT('Ctrl Pts',(-10.2603991795,-36.2742356128,0.677665503434));
#63915=CARTESIAN_POINT('Ctrl Pts',(-10.1672881417,-36.3112466293,0.663071717384));
#63916=CARTESIAN_POINT('Ctrl Pts',(-10.0936931978,-36.3857400536,0.651536792099));
#63917=CARTESIAN_POINT('Ctrl Pts',(-10.0571285787,-36.4799878332,0.645805825719));
#63918=CARTESIAN_POINT('Ctrl Pts',(-10.0571285787,-36.5742356128,0.645805825719));
#63919=CARTESIAN_POINT('Ctrl Pts',(-10.3243887019,-36.2742356128,0.878059911334));
#63920=CARTESIAN_POINT('Ctrl Pts',(-10.2314618653,-36.2742356128,0.862290887462));
#63921=CARTESIAN_POINT('Ctrl Pts',(-10.1385350287,-36.3112466293,0.846521863591));
#63922=CARTESIAN_POINT('Ctrl Pts',(-10.0650856774,-36.3857400536,0.83405803183));
#63923=CARTESIAN_POINT('Ctrl Pts',(-10.0285933941,-36.4799878332,0.827865549396));
#63924=CARTESIAN_POINT('Ctrl Pts',(-10.0285933941,-36.5742356128,0.827865549396));
#63925=CARTESIAN_POINT('Ctrl Pts',(-10.2932212121,-36.2742356128,1.05777080235));
#63926=CARTESIAN_POINT('Ctrl Pts',(-10.2003615355,-36.2742356128,1.04171956338));
#63927=CARTESIAN_POINT('Ctrl Pts',(-10.1075018589,-36.3112466293,1.02566832442));
#63928=CARTESIAN_POINT('Ctrl Pts',(-10.0341055912,-36.3857400536,1.01298142707));
#63929=CARTESIAN_POINT('Ctrl Pts',(-9.99763968115,-36.4799878332,1.00667812186));
#63930=CARTESIAN_POINT('Ctrl Pts',(-9.99763968115,-36.5742356128,1.00667812186));
#63931=CARTESIAN_POINT('Ctrl Pts',(-10.2607745073,-36.2742356128,1.24596085714));
#63932=CARTESIAN_POINT('Ctrl Pts',(-10.1681333202,-36.2742356128,1.22834540563));
#63933=CARTESIAN_POINT('Ctrl Pts',(-10.0754921331,-36.3112466293,1.21072995412));
#63934=CARTESIAN_POINT('Ctrl Pts',(-10.0022685812,-36.3857400536,1.19680667032));
#63935=CARTESIAN_POINT('Ctrl Pts',(-9.96588844999,-36.4799878332,1.18988913349));
#63936=CARTESIAN_POINT('Ctrl Pts',(-9.96588844999,-36.5742356128,1.18988913349));
#63937=CARTESIAN_POINT('Ctrl Pts',(-10.1749701856,-36.2742356128,1.65068933105));
#63938=CARTESIAN_POINT('Ctrl Pts',(-10.0835898455,-36.2742356128,1.62659066301));
#63939=CARTESIAN_POINT('Ctrl Pts',(-9.99220950546,-36.3112466293,1.60249199497));
#63940=CARTESIAN_POINT('Ctrl Pts',(-9.91998248138,-36.3857400536,1.5834444508));
#63941=CARTESIAN_POINT('Ctrl Pts',(-9.88409752911,-36.4799878332,1.57398088825));
#63942=CARTESIAN_POINT('Ctrl Pts',(-9.88409752911,-36.5742356128,1.57398088825));
#63943=CARTESIAN_POINT('Ctrl Pts',(-10.0369131944,-36.2742356128,2.06011773698));
#63944=CARTESIAN_POINT('Ctrl Pts',(-9.94892100813,-36.2742356128,2.02559357059));
#63945=CARTESIAN_POINT('Ctrl Pts',(-9.8609288219,-36.3112466293,1.99106940419));
#63946=CARTESIAN_POINT('Ctrl Pts',(-9.79137984198,-36.3857400536,1.96378146973));
#63947=CARTESIAN_POINT('Ctrl Pts',(-9.75682536651,-36.4799878332,1.95022390222));
#63948=CARTESIAN_POINT('Ctrl Pts',(-9.75682536651,-36.5742356128,1.95022390222));
#63949=CARTESIAN_POINT('Ctrl Pts',(-9.94917208334,-36.2742356128,2.2667545433));
#63950=CARTESIAN_POINT('Ctrl Pts',(-9.86363693513,-36.2742356128,2.22630952643));
#63951=CARTESIAN_POINT('Ctrl Pts',(-9.77810178691,-36.3112466293,2.18586450956));
#63952=CARTESIAN_POINT('Ctrl Pts',(-9.71049472475,-36.3857400536,2.15389693954));
#63953=CARTESIAN_POINT('Ctrl Pts',(-9.67690525041,-36.4799878332,2.13801405614));
#63954=CARTESIAN_POINT('Ctrl Pts',(-9.67690525041,-36.5742356128,2.13801405614));
#63955=CARTESIAN_POINT('Ctrl Pts',(-9.83902583182,-36.2742356128,2.46711999934));
#63956=CARTESIAN_POINT('Ctrl Pts',(-9.75664708714,-36.2742356128,2.42118386819));
#63957=CARTESIAN_POINT('Ctrl Pts',(-9.67426834245,-36.3112466293,2.37524773705));
#63958=CARTESIAN_POINT('Ctrl Pts',(-9.60915626728,-36.3857400536,2.33893972063));
#63959=CARTESIAN_POINT('Ctrl Pts',(-9.57680614337,-36.4799878332,2.32090075257));
#63960=CARTESIAN_POINT('Ctrl Pts',(-9.57680614337,-36.5742356128,2.32090075257));
#63961=CARTESIAN_POINT('Ctrl Pts',(-9.72829200824,-36.2742356128,2.64855052214));
#63962=CARTESIAN_POINT('Ctrl Pts',(-9.64784465104,-36.2742356128,2.59944994453));
#63963=CARTESIAN_POINT('Ctrl Pts',(-9.56739729384,-36.3112466293,2.55034936692));
#63964=CARTESIAN_POINT('Ctrl Pts',(-9.5038117204,-36.3857400536,2.51154028118));
#63965=CARTESIAN_POINT('Ctrl Pts',(-9.4722201171,-36.4799878332,2.49225852944));
#63966=CARTESIAN_POINT('Ctrl Pts',(-9.4722201171,-36.5742356128,2.49225852944));
#63967=CARTESIAN_POINT('',(-9.47221988254214,-36.5742356128,2.49225890563289));
#63968=CARTESIAN_POINT('Origin',(-9.7264810754177,-36.5721143332941,2.64744582231073));
#63969=CARTESIAN_POINT('Ctrl Pts',(-10.0571285787,-36.5742356128,0.645805825719));
#63970=CARTESIAN_POINT('Ctrl Pts',(-10.0512202390646,-36.5742356128,0.683502118786429));
#63971=CARTESIAN_POINT('Ctrl Pts',(-10.045191880218,-36.5742356128,0.721027397434276));
#63972=CARTESIAN_POINT('Ctrl Pts',(-10.039052830587,-36.5742356128,0.758520627395506));
#63973=CARTESIAN_POINT('Ctrl Pts',(-10.0327166412668,-36.5742356128,0.797217855392582));
#63974=CARTESIAN_POINT('Ctrl Pts',(-10.0262621747024,-36.5742356128,0.835880865268867));
#63975=CARTESIAN_POINT('Ctrl Pts',(-10.0196616405614,-36.5742356128,0.874617705186171));
#63976=CARTESIAN_POINT('Ctrl Pts',(-10.0128144444338,-36.5742356128,0.914802140962507));
#63977=CARTESIAN_POINT('Ctrl Pts',(-10.0058096288593,-36.5742356128,0.955065985035107));
#63978=CARTESIAN_POINT('Ctrl Pts',(-9.99858199734885,-36.5742356128,0.995483360467456));
#63979=CARTESIAN_POINT('Ctrl Pts',(-9.99106528890846,-36.5742356128,1.03751727249131));
#63980=CARTESIAN_POINT('Ctrl Pts',(-9.9833070137521,-36.5742356128,1.0797172147409));
#63981=CARTESIAN_POINT('Ctrl Pts',(-9.97520532678219,-36.5742356128,1.12211771621868));
#63982=CARTESIAN_POINT('Ctrl Pts',(-9.96662488168625,-36.5742356128,1.1670238174198));
#63983=CARTESIAN_POINT('Ctrl Pts',(-9.95765844421231,-36.5742356128,1.21215499974358));
#63984=CARTESIAN_POINT('Ctrl Pts',(-9.94816426041759,-36.5742356128,1.25749762852443));
#63985=CARTESIAN_POINT('Ctrl Pts',(-9.93844008755608,-36.5742356128,1.30393864649854));
#63986=CARTESIAN_POINT('Ctrl Pts',(-9.92816108637949,-36.5742356128,1.35060127886798));
#63987=CARTESIAN_POINT('Ctrl Pts',(-9.91716946674835,-36.5742356128,1.39741623621432));
#63988=CARTESIAN_POINT('Ctrl Pts',(-9.90621039827007,-36.5742356128,1.44409255331622));
#63989=CARTESIAN_POINT('Ctrl Pts',(-9.89454156630661,-36.5742356128,1.49091987282535));
#63990=CARTESIAN_POINT('Ctrl Pts',(-9.88202055604576,-36.5742356128,1.53778090756651));
#63991=CARTESIAN_POINT('Ctrl Pts',(-9.8800220437476,-36.5742356128,1.54526052400987));
#63992=CARTESIAN_POINT('Ctrl Pts',(-9.87800187545779,-36.5742356128,1.55274090613695));
#63993=CARTESIAN_POINT('Ctrl Pts',(-9.87595954226258,-36.5742356128,1.56022147294422));
#63994=CARTESIAN_POINT('Ctrl Pts',(-9.87217026083382,-36.5742356128,1.57410068371447));
#63995=CARTESIAN_POINT('Ctrl Pts',(-9.86830430955095,-36.5742356128,1.58798172214129));
#63996=CARTESIAN_POINT('Ctrl Pts',(-9.8643642042847,-36.5742356128,1.60184532111123));
#63997=CARTESIAN_POINT('Ctrl Pts',(-9.84832680476092,-36.5742356128,1.65827428950022));
#63998=CARTESIAN_POINT('Ctrl Pts',(-9.83104562941538,-36.5742356128,1.71447457739543));
#63999=CARTESIAN_POINT('Ctrl Pts',(-9.81234709545891,-36.5742356128,1.77036490831683));
#64000=CARTESIAN_POINT('Ctrl Pts',(-9.80179728711155,-36.5742356128,1.80189851844177));
#64001=CARTESIAN_POINT('Ctrl Pts',(-9.79079560997722,-36.5742356128,1.83333468885662));
#64002=CARTESIAN_POINT('Ctrl Pts',(-9.77931157200682,-36.5742356128,1.86466494021047));
#64003=CARTESIAN_POINT('Ctrl Pts',(-9.77215186764178,-36.5742356128,1.8841977332885));
#64004=CARTESIAN_POINT('Ctrl Pts',(-9.76480472005903,-36.5742356128,1.90368942396184));
#64005=CARTESIAN_POINT('Ctrl Pts',(-9.75726381835173,-36.5742356128,1.92313827869078));
#64006=CARTESIAN_POINT('Ctrl Pts',(-9.75220095002517,-36.5742356128,1.93619599969247));
#64007=CARTESIAN_POINT('Ctrl Pts',(-9.7470500063913,-36.5742356128,1.94923629340378));
#64008=CARTESIAN_POINT('Ctrl Pts',(-9.74181183174468,-36.5742356128,1.96225262541807));
#64009=CARTESIAN_POINT('Ctrl Pts',(-9.72550464318401,-36.5742356128,2.00277433285331));
#64010=CARTESIAN_POINT('Ctrl Pts',(-9.70837226896001,-36.5742356128,2.0430049326535));
#64011=CARTESIAN_POINT('Ctrl Pts',(-9.69043140056761,-36.5742356128,2.08287240096882));
#64012=CARTESIAN_POINT('Ctrl Pts',(-9.67400285885705,-36.5742356128,2.11937923841878));
#64013=CARTESIAN_POINT('Ctrl Pts',(-9.65689624141328,-36.5742356128,2.1555819110846));
#64014=CARTESIAN_POINT('Ctrl Pts',(-9.63916750428284,-36.5742356128,2.19141965241515));
#64015=CARTESIAN_POINT('Ctrl Pts',(-9.62199168890653,-36.5742356128,2.2261396905131));
#64016=CARTESIAN_POINT('Ctrl Pts',(-9.6042316575573,-36.5742356128,2.2605174515297));
#64017=CARTESIAN_POINT('Ctrl Pts',(-9.58598418264596,-36.5742356128,2.29448826760494));
#64018=CARTESIAN_POINT('Ctrl Pts',(-9.56778747896572,-36.5742356128,2.32836456429256));
#64019=CARTESIAN_POINT('Ctrl Pts',(-9.54910565419454,-36.5742356128,2.36183641627422));
#64020=CARTESIAN_POINT('Ctrl Pts',(-9.53008640475237,-36.5742356128,2.39482653491171));
#64021=CARTESIAN_POINT('Ctrl Pts',(-9.51106715531021,-36.5742356128,2.4278166535492));
#64022=CARTESIAN_POINT('Ctrl Pts',(-9.49171019387024,-36.5742356128,2.46032523638466));
#64023=CARTESIAN_POINT('Ctrl Pts',(-9.4722201171,-36.5742356128,2.49225852944));
#64024=CARTESIAN_POINT('Ctrl Pts',(-9.47221976653,-37.9742356128,2.49225909299));
#64025=CARTESIAN_POINT('Ctrl Pts',(-9.47221976653,-38.0684833924,2.49225909299));
#64026=CARTESIAN_POINT('Ctrl Pts',(-9.50381146403,-38.1627311721,2.51154069023));
#64027=CARTESIAN_POINT('Ctrl Pts',(-9.56739722707,-38.2372245963,2.55034946501));
#64028=CARTESIAN_POINT('Ctrl Pts',(-9.64784482414,-38.2742356128,2.59944964919));
#64029=CARTESIAN_POINT('Ctrl Pts',(-9.72829242121,-38.2742356128,2.64854983337));
#64030=CARTESIAN_POINT('Ctrl Pts',(-9.57590405793,-37.9742356128,2.32237883269));
#64031=CARTESIAN_POINT('Ctrl Pts',(-9.57590405797,-38.0684833925,2.32237883264));
#64032=CARTESIAN_POINT('Ctrl Pts',(-9.60823780617,-38.1627311721,2.3404446279));
#64033=CARTESIAN_POINT('Ctrl Pts',(-9.67331602956,-38.2372245964,2.37680809748));
#64034=CARTESIAN_POINT('Ctrl Pts',(-9.75565231855,-38.2742356129,2.42281377752));
#64035=CARTESIAN_POINT('Ctrl Pts',(-9.83798860831,-38.2742356128,2.4688194563));
#64036=CARTESIAN_POINT('Ctrl Pts',(-9.67510718944,-37.9742356128,2.14132026528));
#64037=CARTESIAN_POINT('Ctrl Pts',(-9.67510717979,-38.0684833832,2.14132028047));
#64038=CARTESIAN_POINT('Ctrl Pts',(-9.70868867607,-38.1627311536,2.15721813848));
#64039=CARTESIAN_POINT('Ctrl Pts',(-9.7762810279,-38.2372245746,2.18921365099));
#64040=CARTESIAN_POINT('Ctrl Pts',(-9.86179701536,-38.2742355984,2.22969492403));
#64041=CARTESIAN_POINT('Ctrl Pts',(-9.94731301056,-38.2742356128,2.27017619541));
#64042=CARTESIAN_POINT('Ctrl Pts',(-9.75470839831,-37.9742356128,1.95515325352));
#64043=CARTESIAN_POINT('Ctrl Pts',(-9.75470839104,-38.0684833997,1.95515330638));
#64044=CARTESIAN_POINT('Ctrl Pts',(-9.78923398698,-38.1627311865,1.96877814974));
#64045=CARTESIAN_POINT('Ctrl Pts',(-9.85872451082,-38.2372246133,1.99620198352));
#64046=CARTESIAN_POINT('Ctrl Pts',(-9.94664288255,-38.2742356242,2.03089782227));
#64047=CARTESIAN_POINT('Ctrl Pts',(-10.0345612532,-38.2742356128,2.06559363831));
#64048=CARTESIAN_POINT('Ctrl Pts',(-9.88272651401,-37.9742356128,1.57928798862));
#64049=CARTESIAN_POINT('Ctrl Pts',(-9.88272652097,-38.0684833856,1.57928793803));
#64050=CARTESIAN_POINT('Ctrl Pts',(-9.9186033632,-38.1627311583,1.58879684875));
#64051=CARTESIAN_POINT('Ctrl Pts',(-9.9908143753,-38.2372245801,1.60793521244));
#64052=CARTESIAN_POINT('Ctrl Pts',(-10.0821743219,-38.274235602,1.63214903103));
#64053=CARTESIAN_POINT('Ctrl Pts',(-10.1735342695,-38.2742356128,1.65636287136));
#64054=CARTESIAN_POINT('Ctrl Pts',(-9.96501416235,-37.9742356128,1.19500960441));
#64055=CARTESIAN_POINT('Ctrl Pts',(-9.96501415569,-38.068483399,1.19500965283));
#64056=CARTESIAN_POINT('Ctrl Pts',(-10.0013888155,-38.1627311853,1.20195148351));
#64057=CARTESIAN_POINT('Ctrl Pts',(-10.0746010604,-38.2372246119,1.21592408453));
#64058=CARTESIAN_POINT('Ctrl Pts',(-10.1672280703,-38.2742356232,1.23360170088));
#64059=CARTESIAN_POINT('Ctrl Pts',(-10.2598550792,-38.2742356128,1.25127929642));
#64060=CARTESIAN_POINT('Ctrl Pts',(-9.9970648974,-37.9742356128,1.00998816846));
#64061=CARTESIAN_POINT('Ctrl Pts',(-9.99706491924,-38.0684833994,1.00998803024));
#64062=CARTESIAN_POINT('Ctrl Pts',(-10.0335312152,-38.162731186,1.01628939441));
#64063=CARTESIAN_POINT('Ctrl Pts',(-10.1069282296,-38.2372246127,1.02897258238));
#64064=CARTESIAN_POINT('Ctrl Pts',(-10.1997888365,-38.2742356238,1.04501919899));
#64065=CARTESIAN_POINT('Ctrl Pts',(-10.2926494305,-38.2742356128,1.06106586964));
#64066=CARTESIAN_POINT('Ctrl Pts',(-10.0283268609,-37.9742356128,0.829566080345));
#64067=CARTESIAN_POINT('Ctrl Pts',(-10.0283268609,-38.0684833924,0.829566080345));
#64068=CARTESIAN_POINT('Ctrl Pts',(-10.0648184673,-38.1627311721,0.835762881167));
#64069=CARTESIAN_POINT('Ctrl Pts',(-10.13826646,-38.2372245963,0.848235381488));
#64070=CARTESIAN_POINT('Ctrl Pts',(-10.231191576,-38.2742356128,0.864015382991));
#64071=CARTESIAN_POINT('Ctrl Pts',(-10.3241166921,-38.2742356128,0.879795384186));
#64072=CARTESIAN_POINT('Ctrl Pts',(-10.0571285787,-37.9742356128,0.645805825719));
#64073=CARTESIAN_POINT('Ctrl Pts',(-10.0571285787,-38.0684833924,0.645805825719));
#64074=CARTESIAN_POINT('Ctrl Pts',(-10.0936931978,-38.1627311721,0.651536792099));
#64075=CARTESIAN_POINT('Ctrl Pts',(-10.1672881417,-38.2372245963,0.663071717384));
#64076=CARTESIAN_POINT('Ctrl Pts',(-10.2603991795,-38.2742356128,0.677665503434));
#64077=CARTESIAN_POINT('Ctrl Pts',(-10.3535102174,-38.2742356128,0.692259289483));
#64078=CARTESIAN_POINT('',(-9.47221976654,-37.9742356128,2.49225909299));
#64079=CARTESIAN_POINT('Ctrl Pts',(-10.0571285787,-37.9742356128,0.645805825719));
#64080=CARTESIAN_POINT('Ctrl Pts',(-10.0283268609,-37.9742356128,0.829566080345));
#64081=CARTESIAN_POINT('Ctrl Pts',(-9.9970648974,-37.9742356128,1.00998816846));
#64082=CARTESIAN_POINT('Ctrl Pts',(-9.96501416235,-37.9742356128,1.19500960441));
#64083=CARTESIAN_POINT('Ctrl Pts',(-9.88272651401,-37.9742356128,1.57928798862));
#64084=CARTESIAN_POINT('Ctrl Pts',(-9.75470839830999,-37.9742356128,1.95515325352));
#64085=CARTESIAN_POINT('Ctrl Pts',(-9.67510718944,-37.9742356128,2.14132026528));
#64086=CARTESIAN_POINT('Ctrl Pts',(-9.57590405793,-37.9742356128,2.32237883269));
#64087=CARTESIAN_POINT('Ctrl Pts',(-9.47221976654,-37.9742356128,2.49225909299));
#64088=CARTESIAN_POINT('Origin',(-9.72648173905357,-37.9763569039206,2.64744470617795));
#64089=CARTESIAN_POINT('Ctrl Pts',(-10.0571285787,-37.9742356128,0.645805825719));
#64090=CARTESIAN_POINT('Ctrl Pts',(-10.0571285787,-36.2942356128,0.645805825719));
#64091=CARTESIAN_POINT('Ctrl Pts',(-10.0282717836,-37.9742356128,0.829917483843));
#64092=CARTESIAN_POINT('Ctrl Pts',(-10.0282717836,-36.2942356128,0.829917483843));
#64093=CARTESIAN_POINT('Ctrl Pts',(-9.9971133399,-37.9742356128,1.00951164248));
#64094=CARTESIAN_POINT('Ctrl Pts',(-9.9971133399,-36.2942356128,1.00951164248));
#64095=CARTESIAN_POINT('Ctrl Pts',(-9.9650475466,-37.9742356128,1.19577528245));
#64096=CARTESIAN_POINT('Ctrl Pts',(-9.9650475466,-36.2942356128,1.19577528245));
#64097=CARTESIAN_POINT('Ctrl Pts',(-9.90758702482,-37.9742356128,1.46388856511));
#64098=CARTESIAN_POINT('Ctrl Pts',(-9.90758702482,-36.2942356128,1.46388856511));
#64099=CARTESIAN_POINT('Ctrl Pts',(-9.82673775568,-37.9742356128,1.73070069002));
#64100=CARTESIAN_POINT('Ctrl Pts',(-9.82673775568,-36.2942356128,1.73070069002));
#64101=CARTESIAN_POINT('Ctrl Pts',(-9.80156823449,-37.9742356128,1.80635994999));
#64102=CARTESIAN_POINT('Ctrl Pts',(-9.80156823449,-36.2942356128,1.80635994999));
#64103=CARTESIAN_POINT('Ctrl Pts',(-9.7321123512,-37.9742356128,1.99616841131));
#64104=CARTESIAN_POINT('Ctrl Pts',(-9.7321123512,-36.2942356128,1.99616841131));
#64105=CARTESIAN_POINT('Ctrl Pts',(-9.64855478712,-37.9742356128,2.17984420246));
#64106=CARTESIAN_POINT('Ctrl Pts',(-9.64855478712,-36.2942356128,2.17984420246));
#64107=CARTESIAN_POINT('Ctrl Pts',(-9.59357915013,-37.9742356128,2.28708022821));
#64108=CARTESIAN_POINT('Ctrl Pts',(-9.59357915013,-36.2942356128,2.28708022821));
#64109=CARTESIAN_POINT('Ctrl Pts',(-9.53312961496,-37.9742356128,2.39246209578));
#64110=CARTESIAN_POINT('Ctrl Pts',(-9.53312961496,-36.2942356128,2.39246209578));
#64111=CARTESIAN_POINT('Ctrl Pts',(-9.47221976654,-37.9742356128,2.49225909299));
#64112=CARTESIAN_POINT('Ctrl Pts',(-9.47221976654,-36.2942356128,2.49225909299));
#64113=CARTESIAN_POINT('',(-9.47221976654,-37.2742356128,2.49225909299));
#64114=CARTESIAN_POINT('Ctrl Pts',(-9.72829242121,-36.2742356128,2.64854983337));
#64115=CARTESIAN_POINT('Ctrl Pts',(-9.64784482414,-36.2742356128,2.59944964919));
#64116=CARTESIAN_POINT('Ctrl Pts',(-9.56739722707,-36.3112466293,2.55034946501));
#64117=CARTESIAN_POINT('Ctrl Pts',(-9.50381146403,-36.3857400536,2.51154069022));
#64118=CARTESIAN_POINT('Ctrl Pts',(-9.47221976654,-36.4799878332,2.49225909299));
#64119=CARTESIAN_POINT('Ctrl Pts',(-9.47221976654,-36.5742356128,2.49225909299));
#64120=CARTESIAN_POINT('Ctrl Pts',(-9.62204834183,-36.2742356128,2.82262414757));
#64121=CARTESIAN_POINT('Ctrl Pts',(-9.54341206422,-36.2742356128,2.77055622916));
#64122=CARTESIAN_POINT('Ctrl Pts',(-9.4647757866,-36.3112466293,2.71848831074));
#64123=CARTESIAN_POINT('Ctrl Pts',(-9.40262168945,-36.3857400536,2.67733384035));
#64124=CARTESIAN_POINT('Ctrl Pts',(-9.37174129605,-36.4799878332,2.65688681573));
#64125=CARTESIAN_POINT('Ctrl Pts',(-9.37174129605,-36.5742356128,2.65688681573));
#64126=CARTESIAN_POINT('Ctrl Pts',(-9.50506026008,-36.2742356128,2.99588690652));
#64127=CARTESIAN_POINT('Ctrl Pts',(-9.42877576551,-36.2742356128,2.94035855976));
#64128=CARTESIAN_POINT('Ctrl Pts',(-9.35249127094,-36.3112466293,2.884830213));
#64129=CARTESIAN_POINT('Ctrl Pts',(-9.29219602419,-36.3857400536,2.84094061937));
#64130=CARTESIAN_POINT('Ctrl Pts',(-9.26223917223,-36.4799878332,2.81913468915));
#64131=CARTESIAN_POINT('Ctrl Pts',(-9.26223917223,-36.5742356128,2.81913468915));
#64132=CARTESIAN_POINT('Ctrl Pts',(-9.3722775174,-36.2742356128,3.17398231372));
#64133=CARTESIAN_POINT('Ctrl Pts',(-9.2994440476,-36.2742356128,3.1133047435));
#64134=CARTESIAN_POINT('Ctrl Pts',(-9.22661057779,-36.3112466293,3.05262717327));
#64135=CARTESIAN_POINT('Ctrl Pts',(-9.1690430188,-36.3857400536,3.00466763756));
#64136=CARTESIAN_POINT('Ctrl Pts',(-9.14044138256,-36.4799878332,2.98083960899));
#64137=CARTESIAN_POINT('Ctrl Pts',(-9.14044138256,-36.5742356128,2.98083960899));
#64138=CARTESIAN_POINT('Ctrl Pts',(-9.06627193321,-36.2742356128,3.49560197264));
#64139=CARTESIAN_POINT('Ctrl Pts',(-9.00530329208,-36.2742356128,3.4216519532));
#64140=CARTESIAN_POINT('Ctrl Pts',(-8.94433465096,-36.3112466293,3.34770193375));
#64141=CARTESIAN_POINT('Ctrl Pts',(-8.896145051,-36.3857400536,3.28925185434));
#64142=CARTESIAN_POINT('Ctrl Pts',(-8.87220272103,-36.4799878332,3.26021174991));
#64143=CARTESIAN_POINT('Ctrl Pts',(-8.87220272103,-36.5742356128,3.26021174991));
#64144=CARTESIAN_POINT('Ctrl Pts',(-8.6627303904,-36.2742356128,3.72995773168));
#64145=CARTESIAN_POINT('Ctrl Pts',(-8.62340519663,-36.2742356128,3.64301562554));
#64146=CARTESIAN_POINT('Ctrl Pts',(-8.58408000286,-36.3112466293,3.55607351941));
#64147=CARTESIAN_POINT('Ctrl Pts',(-8.55299737767,-36.3857400536,3.48735449644));
#64148=CARTESIAN_POINT('Ctrl Pts',(-8.53755441086,-36.4799878332,3.45321241259));
#64149=CARTESIAN_POINT('Ctrl Pts',(-8.53755441086,-36.5742356128,3.45321241259));
#64150=CARTESIAN_POINT('Ctrl Pts',(-8.44964730021,-36.2742356128,3.81095134586));
#64151=CARTESIAN_POINT('Ctrl Pts',(-8.42281522522,-36.2742356128,3.71904827968));
#64152=CARTESIAN_POINT('Ctrl Pts',(-8.39598315023,-36.3112466293,3.62714521349));
#64153=CARTESIAN_POINT('Ctrl Pts',(-8.37477508233,-36.3857400536,3.5545050494));
#64154=CARTESIAN_POINT('Ctrl Pts',(-8.36423815285,-36.4799878332,3.51841480048));
#64155=CARTESIAN_POINT('Ctrl Pts',(-8.36423815285,-36.5742356128,3.51841480048));
#64156=CARTESIAN_POINT('Ctrl Pts',(-8.00109574604,-36.2742356128,3.88930872087));
#64157=CARTESIAN_POINT('Ctrl Pts',(-8.00108575718,-36.2742356128,3.79282946445));
#64158=CARTESIAN_POINT('Ctrl Pts',(-8.00107576832,-36.3112466293,3.69635020803));
#64159=CARTESIAN_POINT('Ctrl Pts',(-8.001067873,-36.3857400536,3.62009302536));
#64160=CARTESIAN_POINT('Ctrl Pts',(-8.00106395051,-36.4799878332,3.58220570956));
#64161=CARTESIAN_POINT('Ctrl Pts',(-8.00106395051,-36.5742356128,3.58220570956));
#64162=CARTESIAN_POINT('Ctrl Pts',(-7.55893216723,-36.2742356128,3.81476466023));
#64163=CARTESIAN_POINT('Ctrl Pts',(-7.58431240017,-36.2742356128,3.72263792299));
#64164=CARTESIAN_POINT('Ctrl Pts',(-7.60969263311,-36.3112466293,3.63051118575));
#64165=CARTESIAN_POINT('Ctrl Pts',(-7.62975316565,-36.3857400536,3.55769423287));
#64166=CARTESIAN_POINT('Ctrl Pts',(-7.63971995782,-36.4799878332,3.52151614777));
#64167=CARTESIAN_POINT('Ctrl Pts',(-7.63971995782,-36.5742356128,3.52151614777));
#64168=CARTESIAN_POINT('Ctrl Pts',(-7.3474262191,-36.2742356128,3.73898310239));
#64169=CARTESIAN_POINT('Ctrl Pts',(-7.38416955592,-36.2742356128,3.65120125317));
#64170=CARTESIAN_POINT('Ctrl Pts',(-7.42091289275,-36.3112466293,3.56341940395));
#64171=CARTESIAN_POINT('Ctrl Pts',(-7.44995483128,-36.3857400536,3.49403667229));
#64172=CARTESIAN_POINT('Ctrl Pts',(-7.46438389272,-36.4799878332,3.45956479805));
#64173=CARTESIAN_POINT('Ctrl Pts',(-7.46438389272,-36.5742356128,3.45956479805));
#64174=CARTESIAN_POINT('Ctrl Pts',(-6.95886520076,-36.2742356128,3.53476719039));
#64175=CARTESIAN_POINT('Ctrl Pts',(-7.01431452426,-36.2742356128,3.45705331726));
#64176=CARTESIAN_POINT('Ctrl Pts',(-7.06976384776,-36.3112466293,3.37933944414));
#64177=CARTESIAN_POINT('Ctrl Pts',(-7.11359096799,-36.3857400536,3.31791439199));
#64178=CARTESIAN_POINT('Ctrl Pts',(-7.13536587928,-36.4799878332,3.2873962493));
#64179=CARTESIAN_POINT('Ctrl Pts',(-7.13536587928,-36.5742356128,3.2873962493));
#64180=CARTESIAN_POINT('Ctrl Pts',(-6.64385972405,-36.2742356128,3.24906826835));
#64181=CARTESIAN_POINT('Ctrl Pts',(-6.71208744564,-36.2742356128,3.18320934231));
#64182=CARTESIAN_POINT('Ctrl Pts',(-6.78031516723,-36.3112466293,3.11735041628));
#64183=CARTESIAN_POINT('Ctrl Pts',(-6.83424235588,-36.3857400536,3.06529556086));
#64184=CARTESIAN_POINT('Ctrl Pts',(-6.86103530699,-36.4799878332,3.03943279584));
#64185=CARTESIAN_POINT('Ctrl Pts',(-6.86103530699,-36.5742356128,3.03943279584));
#64186=CARTESIAN_POINT('Ctrl Pts',(-6.50139236315,-36.2742356128,3.08803899971));
#64187=CARTESIAN_POINT('Ctrl Pts',(-6.57495070071,-36.2742356128,3.02825036242));
#64188=CARTESIAN_POINT('Ctrl Pts',(-6.64850903826,-36.3112466293,2.96846172512));
#64189=CARTESIAN_POINT('Ctrl Pts',(-6.7066494798,-36.3857400536,2.92120470051));
#64190=CARTESIAN_POINT('Ctrl Pts',(-6.73553582371,-36.4799878332,2.89772585638));
#64191=CARTESIAN_POINT('Ctrl Pts',(-6.73553582371,-36.5742356128,2.89772585638));
#64192=CARTESIAN_POINT('Ctrl Pts',(-6.37711509272,-36.2742356128,2.91269406835));
#64193=CARTESIAN_POINT('Ctrl Pts',(-6.45574912481,-36.2742356128,2.85992970991));
#64194=CARTESIAN_POINT('Ctrl Pts',(-6.5343831569,-36.3112466293,2.80716535147));
#64195=CARTESIAN_POINT('Ctrl Pts',(-6.59653551323,-36.3857400536,2.76546048015));
#64196=CARTESIAN_POINT('Ctrl Pts',(-6.62741499076,-36.4799878332,2.74473989905));
#64197=CARTESIAN_POINT('Ctrl Pts',(-6.62741499076,-36.5742356128,2.74473989905));
#64198=CARTESIAN_POINT('Ctrl Pts',(-6.27496307903,-36.2742356128,2.72284588841));
#64199=CARTESIAN_POINT('Ctrl Pts',(-6.35795892644,-36.2742356128,2.67818792885));
#64200=CARTESIAN_POINT('Ctrl Pts',(-6.44095477384,-36.3112466293,2.63352996929));
#64201=CARTESIAN_POINT('Ctrl Pts',(-6.50655467338,-36.3857400536,2.59823232788));
#64202=CARTESIAN_POINT('Ctrl Pts',(-6.53914706644,-36.4799878332,2.58069518817));
#64203=CARTESIAN_POINT('Ctrl Pts',(-6.53914706644,-36.5742356128,2.58069518817));
#64204=CARTESIAN_POINT('',(-6.53914703399611,-36.5742356128,2.5806951245344));
#64205=CARTESIAN_POINT('Origin',(-6.27683128588048,-36.5721143277297,2.72184106982266));
#64206=CARTESIAN_POINT('Ctrl Pts',(-9.47221976654,-36.5742356128,2.49225909299));
#64207=CARTESIAN_POINT('Ctrl Pts',(-9.45178452931047,-36.5742356128,2.52574095783471));
#64208=CARTESIAN_POINT('Ctrl Pts',(-9.43084330217428,-36.5742356128,2.55920754094306));
#64209=CARTESIAN_POINT('Ctrl Pts',(-9.40933378143277,-36.5742356128,2.59263503957777));
#64210=CARTESIAN_POINT('Ctrl Pts',(-9.38762982918854,-36.5742356128,2.62636470016531));
#64211=CARTESIAN_POINT('Ctrl Pts',(-9.3653466531979,-36.5742356128,2.66005418215412));
#64212=CARTESIAN_POINT('Ctrl Pts',(-9.34240607923193,-36.5742356128,2.69362043224762));
#64213=CARTESIAN_POINT('Ctrl Pts',(-9.33286416290745,-36.5742356128,2.70758199878009));
#64214=CARTESIAN_POINT('Ctrl Pts',(-9.32320839801377,-36.5742356128,2.72152158549076));
#64215=CARTESIAN_POINT('Ctrl Pts',(-9.31343285049753,-36.5742356128,2.73543055204732));
#64216=CARTESIAN_POINT('Ctrl Pts',(-9.3067521540374,-36.5742356128,2.74493606398759));
#64217=CARTESIAN_POINT('Ctrl Pts',(-9.30001551073448,-36.5742356128,2.75442724329928));
#64218=CARTESIAN_POINT('Ctrl Pts',(-9.29322102418923,-36.5742356128,2.76390095330808));
#64219=CARTESIAN_POINT('Ctrl Pts',(-9.28846887090744,-36.5742356128,2.77052699072964));
#64220=CARTESIAN_POINT('Ctrl Pts',(-9.28368898333415,-36.5742356128,2.77714375911308));
#64221=CARTESIAN_POINT('Ctrl Pts',(-9.27887112661667,-36.5742356128,2.78376311685622));
#64222=CARTESIAN_POINT('Ctrl Pts',(-9.25361775870907,-36.5742356128,2.81845926624413));
#64223=CARTESIAN_POINT('Ctrl Pts',(-9.22738194732705,-36.5742356128,2.85314293661054));
#64224=CARTESIAN_POINT('Ctrl Pts',(-9.2001122283292,-36.5742356128,2.88751310400007));
#64225=CARTESIAN_POINT('Ctrl Pts',(-9.17396931118659,-36.5742356128,2.92046307456312));
#64226=CARTESIAN_POINT('Ctrl Pts',(-9.14687516035206,-36.5742356128,2.95312341883169));
#64227=CARTESIAN_POINT('Ctrl Pts',(-9.11881276730823,-36.5742356128,2.98519628971722));
#64228=CARTESIAN_POINT('Ctrl Pts',(-9.10657791227766,-36.5742356128,2.99917966330499));
#64229=CARTESIAN_POINT('Ctrl Pts',(-9.09415946971097,-36.5742356128,3.01305106866214));
#64230=CARTESIAN_POINT('Ctrl Pts',(-9.08155851754365,-36.5742356128,3.02678491299355));
#64231=CARTESIAN_POINT('Ctrl Pts',(-9.07585005623246,-36.5742356128,3.03300659513144));
#64232=CARTESIAN_POINT('Ctrl Pts',(-9.07010538548969,-36.5742356128,3.03919874111963));
#64233=CARTESIAN_POINT('Ctrl Pts',(-9.06432087221495,-36.5742356128,3.04536306782802));
#64234=CARTESIAN_POINT('Ctrl Pts',(-9.03453905552488,-36.5742356128,3.07710037040262));
#64235=CARTESIAN_POINT('Ctrl Pts',(-9.00355542500468,-36.5742356128,3.10825234925048));
#64236=CARTESIAN_POINT('Ctrl Pts',(-8.97133952680228,-36.5742356128,3.13849784243435));
#64237=CARTESIAN_POINT('Ctrl Pts',(-8.94121606492088,-36.5742356128,3.1667788779431));
#64238=CARTESIAN_POINT('Ctrl Pts',(-8.91001482010756,-36.5742356128,3.19426625312343));
#64239=CARTESIAN_POINT('Ctrl Pts',(-8.8777556198925,-36.5742356128,3.22069087225574));
#64240=CARTESIAN_POINT('Ctrl Pts',(-8.86422662034783,-36.5742356128,3.23177294055954));
#64241=CARTESIAN_POINT('Ctrl Pts',(-8.85051214048935,-36.5742356128,3.24266809673354));
#64242=CARTESIAN_POINT('Ctrl Pts',(-8.83661643344406,-36.5742356128,3.25335680269378));
#64243=CARTESIAN_POINT('Ctrl Pts',(-8.81836242792662,-36.5742356128,3.26739795201684));
#64244=CARTESIAN_POINT('Ctrl Pts',(-8.79979723642711,-36.5742356128,3.28108152158642));
#64245=CARTESIAN_POINT('Ctrl Pts',(-8.78091542981201,-36.5742356128,3.29437421039659));
#64246=CARTESIAN_POINT('Ctrl Pts',(-8.7489680446299,-36.5742356128,3.31686499521297));
#64247=CARTESIAN_POINT('Ctrl Pts',(-8.71609229015667,-36.5742356128,3.33825047301422));
#64248=CARTESIAN_POINT('Ctrl Pts',(-8.68229792411548,-36.5742356128,3.35836411240285));
#64249=CARTESIAN_POINT('Ctrl Pts',(-8.6475947598128,-36.5742356128,3.37901864788303));
#64250=CARTESIAN_POINT('Ctrl Pts',(-8.61192315156315,-36.5742356128,3.39833127668768));
#64251=CARTESIAN_POINT('Ctrl Pts',(-8.57534988837971,-36.5742356128,3.41612220858467));
#64252=CARTESIAN_POINT('Ctrl Pts',(-8.5490844798751,-36.5742356128,3.42889892177015));
#64253=CARTESIAN_POINT('Ctrl Pts',(-8.5223552581089,-36.5742356128,3.44089078500327));
#64254=CARTESIAN_POINT('Ctrl Pts',(-8.49520280272183,-36.5742356128,3.45203482771473));
#64255=CARTESIAN_POINT('Ctrl Pts',(-8.47642666650715,-36.5742356128,3.45974102079929));
#64256=CARTESIAN_POINT('Ctrl Pts',(-8.45744605695094,-36.5742356128,3.46704270285512));
#64257=CARTESIAN_POINT('Ctrl Pts',(-8.43828543372318,-36.5742356128,3.47391782434403));
#64258=CARTESIAN_POINT('Ctrl Pts',(-8.4005107660617,-36.5742356128,3.48747194658153));
#64259=CARTESIAN_POINT('Ctrl Pts',(-8.36205258057802,-36.5742356128,3.49935947844771));
#64260=CARTESIAN_POINT('Ctrl Pts',(-8.32308624720095,-36.5742356128,3.50946141251245));
#64261=CARTESIAN_POINT('Ctrl Pts',(-8.28498059057218,-36.5742356128,3.5193402180709));
#64262=CARTESIAN_POINT('Ctrl Pts',(-8.24638977185156,-36.5742356128,3.52751083953927));
#64263=CARTESIAN_POINT('Ctrl Pts',(-8.20750090981374,-36.5742356128,3.53390471385943));
#64264=CARTESIAN_POINT('Ctrl Pts',(-8.17019437411012,-36.5742356128,3.54003843153873));
#64265=CARTESIAN_POINT('Ctrl Pts',(-8.1326142429901,-36.5742356128,3.54453677805079));
#64266=CARTESIAN_POINT('Ctrl Pts',(-8.09493654742072,-36.5742356128,3.54738491301163));
#64267=CARTESIAN_POINT('Ctrl Pts',(-8.06426248640137,-36.5742356128,3.54970362874676));
#64268=CARTESIAN_POINT('Ctrl Pts',(-8.03352409131106,-36.5742356128,3.55092933198329));
#64269=CARTESIAN_POINT('Ctrl Pts',(-8.00281747813575,-36.5742356128,3.55107964607802));
#64270=CARTESIAN_POINT('Ctrl Pts',(-7.96270277011772,-36.5742356128,3.55127601439733));
#64271=CARTESIAN_POINT('Ctrl Pts',(-7.92264137730165,-36.5742356128,3.54963567943145));
#64272=CARTESIAN_POINT('Ctrl Pts',(-7.88278787617713,-36.5742356128,3.54619249889203));
#64273=CARTESIAN_POINT('Ctrl Pts',(-7.8405011481773,-36.5742356128,3.54253909743881));
#64274=CARTESIAN_POINT('Ctrl Pts',(-7.79844929680864,-36.5742356128,3.53685642893967));
#64275=CARTESIAN_POINT('Ctrl Pts',(-7.75682042603883,-36.5742356128,3.52924798342734));
#64276=CARTESIAN_POINT('Ctrl Pts',(-7.73188548808965,-36.5742356128,3.52469066267299));
#64277=CARTESIAN_POINT('Ctrl Pts',(-7.70710231204621,-36.5742356128,3.51944358499482));
#64278=CARTESIAN_POINT('Ctrl Pts',(-7.68250988053131,-36.5742356128,3.51353757033189));
#64279=CARTESIAN_POINT('Ctrl Pts',(-7.66774913753318,-36.5742356128,3.50999269252955));
#64280=CARTESIAN_POINT('Ctrl Pts',(-7.65305760413022,-36.5742356128,3.50621083142867));
#64281=CARTESIAN_POINT('Ctrl Pts',(-7.63842877546141,-36.5742356128,3.50219506857823));
#64282=CARTESIAN_POINT('Ctrl Pts',(-7.59473414475351,-36.5742356128,3.49020044626549));
#64283=CARTESIAN_POINT('Ctrl Pts',(-7.55163483891475,-36.5742356128,3.47612347756162));
#64284=CARTESIAN_POINT('Ctrl Pts',(-7.50935266584155,-36.5742356128,3.4601746702419));
#64285=CARTESIAN_POINT('Ctrl Pts',(-7.46870308154542,-36.5742356128,3.44484167431373));
#64286=CARTESIAN_POINT('Ctrl Pts',(-7.4288095588,-36.5742356128,3.42778024800884));
#64287=CARTESIAN_POINT('Ctrl Pts',(-7.38982831413737,-36.5742356128,3.40920241830386));
#64288=CARTESIAN_POINT('Ctrl Pts',(-7.3633352747518,-36.5742356128,3.39657626492337));
#64289=CARTESIAN_POINT('Ctrl Pts',(-7.33726275758436,-36.5742356128,3.38325016153255));
#64290=CARTESIAN_POINT('Ctrl Pts',(-7.31164578606096,-36.5742356128,3.36929213910639));
#64291=CARTESIAN_POINT('Ctrl Pts',(-7.29176246227058,-36.5742356128,3.35845823240828));
#64292=CARTESIAN_POINT('Ctrl Pts',(-7.27214586950384,-36.5742356128,3.34723983933327));
#64293=CARTESIAN_POINT('Ctrl Pts',(-7.25279266780678,-36.5742356128,3.33565750429941));
#64294=CARTESIAN_POINT('Ctrl Pts',(-7.21928492757203,-36.5742356128,3.31560408473085));
#64295=CARTESIAN_POINT('Ctrl Pts',(-7.18657606175943,-36.5742356128,3.29446497149353));
#64296=CARTESIAN_POINT('Ctrl Pts',(-7.15465499843816,-36.5742356128,3.27234915626901));
#64297=CARTESIAN_POINT('Ctrl Pts',(-7.11154237878949,-36.5742356128,3.24247951438399));
#64298=CARTESIAN_POINT('Ctrl Pts',(-7.06985594727397,-36.5742356128,3.21082568782116));
#64299=CARTESIAN_POINT('Ctrl Pts',(-7.02958048187159,-36.5742356128,3.17758678921859));
#64300=CARTESIAN_POINT('Ctrl Pts',(-6.98830979588565,-36.5742356128,3.14352654601492));
#64301=CARTESIAN_POINT('Ctrl Pts',(-6.94852125819688,-36.5742356128,3.10780256054435));
#64302=CARTESIAN_POINT('Ctrl Pts',(-6.91024718858311,-36.5742356128,3.07060371749456));
#64303=CARTESIAN_POINT('Ctrl Pts',(-6.87168160917733,-36.5742356128,3.03312155398501));
#64304=CARTESIAN_POINT('Ctrl Pts',(-6.83465434719058,-36.5742356128,2.99414259605905));
#64305=CARTESIAN_POINT('Ctrl Pts',(-6.79923734995239,-36.5742356128,2.95382526881695));
#64306=CARTESIAN_POINT('Ctrl Pts',(-6.76426659337508,-36.5742356128,2.91401592452532));
#64307=CARTESIAN_POINT('Ctrl Pts',(-6.7308664945914,-36.5742356128,2.87290222361067));
#64308=CARTESIAN_POINT('Ctrl Pts',(-6.6991334408564,-36.5742356128,2.83059477854831));
#64309=CARTESIAN_POINT('Ctrl Pts',(-6.66863403289319,-36.5742356128,2.78993206648746));
#64310=CARTESIAN_POINT('Ctrl Pts',(-6.63967521531564,-36.5742356128,2.74816688282246));
#64311=CARTESIAN_POINT('Ctrl Pts',(-6.61235787702105,-36.5742356128,2.70535332001463));
#64312=CARTESIAN_POINT('Ctrl Pts',(-6.58644612667648,-36.5742356128,2.66474268881497));
#64313=CARTESIAN_POINT('Ctrl Pts',(-6.56201175880056,-36.5742356128,2.62318890122085));
#64314=CARTESIAN_POINT('Ctrl Pts',(-6.53914706644,-36.5742356128,2.58069518817));
#64315=CARTESIAN_POINT('Ctrl Pts',(-6.53914719008,-37.9742356128,2.58069542603));
#64316=CARTESIAN_POINT('Ctrl Pts',(-6.53914719078,-38.0684833925,2.58069542736));
#64317=CARTESIAN_POINT('Ctrl Pts',(-6.50655468231,-38.1627311721,2.59823235248));
#64318=CARTESIAN_POINT('Ctrl Pts',(-6.44095454962,-38.2372245964,2.63352956036));
#64319=CARTESIAN_POINT('Ctrl Pts',(-6.35795840683,-38.2742356129,2.67818697059));
#64320=CARTESIAN_POINT('Ctrl Pts',(-6.27496226376,-38.2742356128,2.7228443803));
#64321=CARTESIAN_POINT('Ctrl Pts',(-6.60862882414,-37.9742356128,2.70982607508));
#64322=CARTESIAN_POINT('Ctrl Pts',(-6.60862879596,-38.0684833921,2.70982602153));
#64323=CARTESIAN_POINT('Ctrl Pts',(-6.57738634684,-38.1627311713,2.72987203609));
#64324=CARTESIAN_POINT('Ctrl Pts',(-6.5145035418,-38.2372245954,2.7702194031));
#64325=CARTESIAN_POINT('Ctrl Pts',(-6.43494534104,-38.2742356122,2.8212662386));
#64326=CARTESIAN_POINT('Ctrl Pts',(-6.35538715106,-38.2742356128,2.8723130951));
#64327=CARTESIAN_POINT('Ctrl Pts',(-6.69040968596,-37.9742356128,2.83211943121));
#64328=CARTESIAN_POINT('Ctrl Pts',(-6.69040972795,-38.0684833969,2.83211950901));
#64329=CARTESIAN_POINT('Ctrl Pts',(-6.66068017578,-38.162731181,2.85439814262));
#64330=CARTESIAN_POINT('Ctrl Pts',(-6.60084240217,-38.2372246069,2.89923913281));
#64331=CARTESIAN_POINT('Ctrl Pts',(-6.52513665775,-38.2742356199,2.95597109413));
#64332=CARTESIAN_POINT('Ctrl Pts',(-6.44943089912,-38.2742356128,3.0127030234));
#64333=CARTESIAN_POINT('Ctrl Pts',(-6.78293784481,-37.9742356128,2.94714618869));
#64334=CARTESIAN_POINT('Ctrl Pts',(-6.78293783118,-38.0684833893,2.94714616566));
#64335=CARTESIAN_POINT('Ctrl Pts',(-6.75483332907,-38.1627311657,2.97143599883));
#64336=CARTESIAN_POINT('Ctrl Pts',(-6.69826638119,-38.2372245888,3.02032504454));
#64337=CARTESIAN_POINT('Ctrl Pts',(-6.62669887685,-38.2742356078,3.0821786334));
#64338=CARTESIAN_POINT('Ctrl Pts',(-6.55513137645,-38.2742356128,3.14403223264));
#64339=CARTESIAN_POINT('Ctrl Pts',(-7.02925067951,-37.9742356128,3.20337077768));
#64340=CARTESIAN_POINT('Ctrl Pts',(-7.02925069855,-38.0684833969,3.20337080984));
#64341=CARTESIAN_POINT('Ctrl Pts',(-7.0054973778,-38.1627311809,3.23224071513));
#64342=CARTESIAN_POINT('Ctrl Pts',(-6.95768819081,-38.2372246068,3.29034821166));
#64343=CARTESIAN_POINT('Ctrl Pts',(-6.89720082675,-38.2742356198,3.36386477088));
#64344=CARTESIAN_POINT('Ctrl Pts',(-6.8367134572,-38.2742356128,3.43738131562));
#64345=CARTESIAN_POINT('Ctrl Pts',(-7.32593788713,-37.9742356128,3.39828475585));
#64346=CARTESIAN_POINT('Ctrl Pts',(-7.32593786055,-38.0684833862,3.39828471095));
#64347=CARTESIAN_POINT('Ctrl Pts',(-7.30823659937,-38.1627311597,3.43122238484));
#64348=CARTESIAN_POINT('Ctrl Pts',(-7.27260863663,-38.2372245817,3.49751726565));
#64349=CARTESIAN_POINT('Ctrl Pts',(-7.22753278341,-38.2742356031,3.58139243425));
#64350=CARTESIAN_POINT('Ctrl Pts',(-7.18245693785,-38.2742356128,3.66526762307));
#64351=CARTESIAN_POINT('Ctrl Pts',(-7.51861181031,-37.9742356128,3.48826721235));
#64352=CARTESIAN_POINT('Ctrl Pts',(-7.51861177171,-38.0684833924,3.48826721752));
#64353=CARTESIAN_POINT('Ctrl Pts',(-7.50543345832,-38.1627311719,3.52352395259));
#64354=CARTESIAN_POINT('Ctrl Pts',(-7.4789090267,-38.2372245962,3.59448646302));
#64355=CARTESIAN_POINT('Ctrl Pts',(-7.44535080562,-38.2742356127,3.68426698954));
#64356=CARTESIAN_POINT('Ctrl Pts',(-7.4117926006,-38.2742356128,3.77404751415));
#64357=CARTESIAN_POINT('Ctrl Pts',(-7.91545972539,-37.9742356128,3.58665245723));
#64358=CARTESIAN_POINT('Ctrl Pts',(-7.91545976172,-38.0684833925,3.58665245236));
#64359=CARTESIAN_POINT('Ctrl Pts',(-7.91297425904,-38.1627311722,3.62465357638));
#64360=CARTESIAN_POINT('Ctrl Pts',(-7.90797155303,-38.2372245965,3.70113983127));
#64361=CARTESIAN_POINT('Ctrl Pts',(-7.90164219398,-38.2742356129,3.79790890862));
#64362=CARTESIAN_POINT('Ctrl Pts',(-7.89531281982,-38.2742356128,3.89467798777));
#64363=CARTESIAN_POINT('Ctrl Pts',(-8.32196834325,-37.9742356128,3.53349085056));
#64364=CARTESIAN_POINT('Ctrl Pts',(-8.32196830907,-38.0684833924,3.53349085514));
#64365=CARTESIAN_POINT('Ctrl Pts',(-8.33127827363,-38.1627311719,3.57001419685));
#64366=CARTESIAN_POINT('Ctrl Pts',(-8.35001682583,-38.2372245962,3.64352605744));
#64367=CARTESIAN_POINT('Ctrl Pts',(-8.37372453412,-38.2742356127,3.73653197592));
#64368=CARTESIAN_POINT('Ctrl Pts',(-8.39743225663,-38.2742356128,3.82953789272));
#64369=CARTESIAN_POINT('Ctrl Pts',(-8.51257873567,-37.9742356128,3.46755862103));
#64370=CARTESIAN_POINT('Ctrl Pts',(-8.51257875377,-38.0684833947,3.46755862147));
#64371=CARTESIAN_POINT('Ctrl Pts',(-8.52738481159,-38.1627311765,3.50208416494));
#64372=CARTESIAN_POINT('Ctrl Pts',(-8.55718585956,-38.2372246016,3.57157437773));
#64373=CARTESIAN_POINT('Ctrl Pts',(-8.59488945106,-38.2742356164,3.65949244318));
#64374=CARTESIAN_POINT('Ctrl Pts',(-8.63259303718,-38.2742356128,3.74741050329));
#64375=CARTESIAN_POINT('Ctrl Pts',(-8.86229619026,-37.9742356128,3.27052379371));
#64376=CARTESIAN_POINT('Ctrl Pts',(-8.86229617129,-38.0684833901,3.27052379325));
#64377=CARTESIAN_POINT('Ctrl Pts',(-8.88606803187,-38.1627311673,3.2997528949));
#64378=CARTESIAN_POINT('Ctrl Pts',(-8.9339141532,-38.2372245908,3.35858401846));
#64379=CARTESIAN_POINT('Ctrl Pts',(-8.99444841221,-38.2742356091,3.43301585235));
#64380=CARTESIAN_POINT('Ctrl Pts',(-9.05498267684,-38.2742356128,3.50744769184));
#64381=CARTESIAN_POINT('Ctrl Pts',(-9.14074177278,-37.9742356128,2.98053227682));
#64382=CARTESIAN_POINT('Ctrl Pts',(-9.14074179266,-38.0684833949,2.9805322773));
#64383=CARTESIAN_POINT('Ctrl Pts',(-9.16934690231,-38.162731177,3.00435821305));
#64384=CARTESIAN_POINT('Ctrl Pts',(-9.22692183769,-38.2372246021,3.05231286426));
#64385=CARTESIAN_POINT('Ctrl Pts',(-9.29976445069,-38.2742356167,3.11298454342));
#64386=CARTESIAN_POINT('Ctrl Pts',(-9.37260705779,-38.2742356128,3.1736562167));
#64387=CARTESIAN_POINT('Ctrl Pts',(-9.26235716204,-37.9742356128,2.81894517549));
#64388=CARTESIAN_POINT('Ctrl Pts',(-9.2623571652,-38.0684833948,2.81894517181));
#64389=CARTESIAN_POINT('Ctrl Pts',(-9.29231496964,-38.1627311767,2.84074916224));
#64390=CARTESIAN_POINT('Ctrl Pts',(-9.35261048666,-38.2372246019,2.88463754863));
#64391=CARTESIAN_POINT('Ctrl Pts',(-9.42889602942,-38.2742356165,2.94016320761));
#64392=CARTESIAN_POINT('Ctrl Pts',(-9.50518155925,-38.2742356128,2.99568888448));
#64393=CARTESIAN_POINT('Ctrl Pts',(-9.37180357922,-37.9742356128,2.65678476864));
#64394=CARTESIAN_POINT('Ctrl Pts',(-9.37180357922,-38.0684833924,2.65678476864));
#64395=CARTESIAN_POINT('Ctrl Pts',(-9.40268405231,-38.1627311721,2.67723166281));
#64396=CARTESIAN_POINT('Ctrl Pts',(-9.46483940501,-38.2372245963,2.71838407584));
#64397=CARTESIAN_POINT('Ctrl Pts',(-9.54347679851,-38.2742356128,2.77045016604));
#64398=CARTESIAN_POINT('Ctrl Pts',(-9.6221141989,-38.2742356128,2.82251624486));
#64399=CARTESIAN_POINT('Ctrl Pts',(-9.47221976654,-37.9742356128,2.49225909299));
#64400=CARTESIAN_POINT('Ctrl Pts',(-9.47221976654,-38.0684833924,2.49225909299));
#64401=CARTESIAN_POINT('Ctrl Pts',(-9.50381146403,-38.1627311721,2.51154069022));
#64402=CARTESIAN_POINT('Ctrl Pts',(-9.56739722707,-38.2372245963,2.55034946501));
#64403=CARTESIAN_POINT('Ctrl Pts',(-9.64784482414,-38.2742356128,2.59944964919));
#64404=CARTESIAN_POINT('Ctrl Pts',(-9.72829242121,-38.2742356128,2.64854983337));
#64405=CARTESIAN_POINT('',(-6.53914701908,-37.9742356128,2.5806950957));
#64406=CARTESIAN_POINT('Ctrl Pts',(-9.47221976654,-37.9742356128,2.49225909299));
#64407=CARTESIAN_POINT('Ctrl Pts',(-9.37180357922,-37.9742356128,2.65678476864));
#64408=CARTESIAN_POINT('Ctrl Pts',(-9.26235716204,-37.9742356128,2.81894517549));
#64409=CARTESIAN_POINT('Ctrl Pts',(-9.14074177278,-37.9742356128,2.98053227682));
#64410=CARTESIAN_POINT('Ctrl Pts',(-8.86229619026,-37.9742356128,3.27052379371));
#64411=CARTESIAN_POINT('Ctrl Pts',(-8.51257873567,-37.9742356128,3.46755862103));
#64412=CARTESIAN_POINT('Ctrl Pts',(-8.32196834325,-37.9742356128,3.53349085056));
#64413=CARTESIAN_POINT('Ctrl Pts',(-7.91545972539,-37.9742356128,3.58665245723));
#64414=CARTESIAN_POINT('Ctrl Pts',(-7.51861181031,-37.9742356128,3.48826721235));
#64415=CARTESIAN_POINT('Ctrl Pts',(-7.32593788713,-37.9742356128,3.39828475585));
#64416=CARTESIAN_POINT('Ctrl Pts',(-7.02925067951,-37.9742356128,3.20337077768));
#64417=CARTESIAN_POINT('Ctrl Pts',(-6.78293784481,-37.9742356128,2.94714618869));
#64418=CARTESIAN_POINT('Ctrl Pts',(-6.69040968596,-37.9742356128,2.83211943121));
#64419=CARTESIAN_POINT('Ctrl Pts',(-6.60862882414,-37.9742356128,2.70982607508));
#64420=CARTESIAN_POINT('Ctrl Pts',(-6.53914701908,-37.9742356128,2.5806950957));
#64421=CARTESIAN_POINT('Origin',(-6.2768299648437,-37.9763568910239,2.72183863295591));
#64422=CARTESIAN_POINT('Ctrl Pts',(-9.47221976654,-37.9742356128,2.49225909299));
#64423=CARTESIAN_POINT('Ctrl Pts',(-9.47221976654,-36.2942356128,2.49225909299));
#64424=CARTESIAN_POINT('Ctrl Pts',(-9.43799021757,-37.9742356128,2.54834207942));
#64425=CARTESIAN_POINT('Ctrl Pts',(-9.43799021757,-36.2942356128,2.54834207942));
#64426=CARTESIAN_POINT('Ctrl Pts',(-9.40258508843,-37.9742356128,2.60436998551));
#64427=CARTESIAN_POINT('Ctrl Pts',(-9.40258508843,-36.2942356128,2.60436998551));
#64428=CARTESIAN_POINT('Ctrl Pts',(-9.36584102959,-37.9742356128,2.66040353433));
#64429=CARTESIAN_POINT('Ctrl Pts',(-9.36584102959,-36.2942356128,2.66040353433));
#64430=CARTESIAN_POINT('Ctrl Pts',(-9.28925382834,-37.9742356128,2.77218463031));
#64431=CARTESIAN_POINT('Ctrl Pts',(-9.28925382834,-36.2942356128,2.77218463031));
#64432=CARTESIAN_POINT('Ctrl Pts',(-9.20593013024,-37.9742356128,2.88194354511));
#64433=CARTESIAN_POINT('Ctrl Pts',(-9.20593013024,-36.2942356128,2.88194354511));
#64434=CARTESIAN_POINT('Ctrl Pts',(-9.16069630404,-37.9742356128,2.93809779908));
#64435=CARTESIAN_POINT('Ctrl Pts',(-9.16069630404,-36.2942356128,2.93809779908));
#64436=CARTESIAN_POINT('Ctrl Pts',(-9.06741515882,-37.9742356128,3.0462171446));
#64437=CARTESIAN_POINT('Ctrl Pts',(-9.06741515882,-36.2942356128,3.0462171446));
#64438=CARTESIAN_POINT('Ctrl Pts',(-8.9630009386,-37.9742356128,3.14917335528));
#64439=CARTESIAN_POINT('Ctrl Pts',(-8.9630009386,-36.2942356128,3.14917335528));
#64440=CARTESIAN_POINT('Ctrl Pts',(-8.90717355699,-37.9742356128,3.19917508688));
#64441=CARTESIAN_POINT('Ctrl Pts',(-8.90717355699,-36.2942356128,3.19917508688));
#64442=CARTESIAN_POINT('Ctrl Pts',(-8.78922597568,-37.9742356128,3.29398598989));
#64443=CARTESIAN_POINT('Ctrl Pts',(-8.78922597568,-36.2942356128,3.29398598989));
#64444=CARTESIAN_POINT('Ctrl Pts',(-8.65978894936,-37.9742356128,3.37495922004));
#64445=CARTESIAN_POINT('Ctrl Pts',(-8.65978894936,-36.2942356128,3.37495922004));
#64446=CARTESIAN_POINT('Ctrl Pts',(-8.59150582736,-37.9742356128,3.41174862899));
#64447=CARTESIAN_POINT('Ctrl Pts',(-8.59150582736,-36.2942356128,3.41174862899));
#64448=CARTESIAN_POINT('Ctrl Pts',(-8.37641925249,-37.9742356128,3.50886242158));
#64449=CARTESIAN_POINT('Ctrl Pts',(-8.37641925249,-36.2942356128,3.50886242158));
#64450=CARTESIAN_POINT('Ctrl Pts',(-8.13973403839,-37.9742356128,3.5585372531));
#64451=CARTESIAN_POINT('Ctrl Pts',(-8.13973403839,-36.2942356128,3.5585372531));
#64452=CARTESIAN_POINT('Ctrl Pts',(-7.97806372235,-37.9742356128,3.56548871191));
#64453=CARTESIAN_POINT('Ctrl Pts',(-7.97806372235,-36.2942356128,3.56548871191));
#64454=CARTESIAN_POINT('Ctrl Pts',(-7.74013214217,-37.9742356128,3.53951961667));
#64455=CARTESIAN_POINT('Ctrl Pts',(-7.74013214217,-36.2942356128,3.53951961667));
#64456=CARTESIAN_POINT('Ctrl Pts',(-7.51591788103,-37.9742356128,3.46603879043));
#64457=CARTESIAN_POINT('Ctrl Pts',(-7.51591788103,-36.2942356128,3.46603879043));
#64458=CARTESIAN_POINT('Ctrl Pts',(-7.44307437439,-37.9742356128,3.43661441301));
#64459=CARTESIAN_POINT('Ctrl Pts',(-7.44307437439,-36.2942356128,3.43661441301));
#64460=CARTESIAN_POINT('Ctrl Pts',(-7.16744129772,-37.9742356128,3.30480694269));
#64461=CARTESIAN_POINT('Ctrl Pts',(-7.16744129772,-36.2942356128,3.30480694269));
#64462=CARTESIAN_POINT('Ctrl Pts',(-6.93248240874,-37.9742356128,3.11682904882));
#64463=CARTESIAN_POINT('Ctrl Pts',(-6.93248240874,-36.2942356128,3.11682904882));
#64464=CARTESIAN_POINT('Ctrl Pts',(-6.77645737492,-37.9742356128,2.95406352231));
#64465=CARTESIAN_POINT('Ctrl Pts',(-6.77645737492,-36.2942356128,2.95406352231));
#64466=CARTESIAN_POINT('Ctrl Pts',(-6.64407030457,-37.9742356128,2.77569349664));
#64467=CARTESIAN_POINT('Ctrl Pts',(-6.64407030457,-36.2942356128,2.77569349664));
#64468=CARTESIAN_POINT('Ctrl Pts',(-6.53914701908,-37.9742356128,2.5806950957));
#64469=CARTESIAN_POINT('Ctrl Pts',(-6.53914701908,-36.2942356128,2.5806950957));
#64470=CARTESIAN_POINT('',(-6.53914701908,-37.2742356128,2.5806950957));
#64471=CARTESIAN_POINT('Ctrl Pts',(-6.2749628032,-36.2742356128,2.72284536858));
#64472=CARTESIAN_POINT('Ctrl Pts',(-6.35795872238,-36.2742356128,2.67818754328));
#64473=CARTESIAN_POINT('Ctrl Pts',(-6.44095464156,-36.3112466293,2.63352971798));
#64474=CARTESIAN_POINT('Ctrl Pts',(-6.50655459783,-36.3857400536,2.59823218268));
#64475=CARTESIAN_POINT('Ctrl Pts',(-6.53914701908,-36.4799878332,2.5806950957));
#64476=CARTESIAN_POINT('Ctrl Pts',(-6.53914701908,-36.5742356128,2.5806950957));
#64477=CARTESIAN_POINT('Ctrl Pts',(-6.20857721065,-36.2742356128,2.59946870979));
#64478=CARTESIAN_POINT('Ctrl Pts',(-6.29440217543,-36.2742356128,2.56006862461));
#64479=CARTESIAN_POINT('Ctrl Pts',(-6.3802271402,-36.3112466293,2.52066853944));
#64480=CARTESIAN_POINT('Ctrl Pts',(-6.44806317297,-36.3857400536,2.48952672142));
#64481=CARTESIAN_POINT('Ctrl Pts',(-6.48176655835,-36.4799878332,2.4740543435));
#64482=CARTESIAN_POINT('Ctrl Pts',(-6.48176655835,-36.5742356128,2.4740543435));
#64483=CARTESIAN_POINT('Ctrl Pts',(-6.15321817523,-36.2742356128,2.47317175996));
#64484=CARTESIAN_POINT('Ctrl Pts',(-6.24090872024,-36.2742356128,2.43823633957));
#64485=CARTESIAN_POINT('Ctrl Pts',(-6.32859926526,-36.3112466293,2.40330091918));
#64486=CARTESIAN_POINT('Ctrl Pts',(-6.39790985368,-36.3857400536,2.37568796974));
#64487=CARTESIAN_POINT('Ctrl Pts',(-6.43234584926,-36.4799878332,2.36196886307));
#64488=CARTESIAN_POINT('Ctrl Pts',(-6.43234584926,-36.5742356128,2.36196886307));
#64489=CARTESIAN_POINT('Ctrl Pts',(-6.10591213658,-36.2742356128,2.34560093633));
#64490=CARTESIAN_POINT('Ctrl Pts',(-6.19476895256,-36.2742356128,2.31400987032));
#64491=CARTESIAN_POINT('Ctrl Pts',(-6.28362576853,-36.3112466293,2.2824188043));
#64492=CARTESIAN_POINT('Ctrl Pts',(-6.35385817691,-36.3857400536,2.2574492336));
#64493=CARTESIAN_POINT('Ctrl Pts',(-6.38875216637,-36.4799878332,2.24504345006));
#64494=CARTESIAN_POINT('Ctrl Pts',(-6.38875216637,-36.5742356128,2.24504345006));
#64495=CARTESIAN_POINT('Ctrl Pts',(-6.04521899885,-36.2742356128,2.16171106337));
#64496=CARTESIAN_POINT('Ctrl Pts',(-6.13521792579,-36.2742356128,2.13366813026));
#64497=CARTESIAN_POINT('Ctrl Pts',(-6.22521685274,-36.3112466293,2.10562519715));
#64498=CARTESIAN_POINT('Ctrl Pts',(-6.29635198481,-36.3857400536,2.08346006881));
#64499=CARTESIAN_POINT('Ctrl Pts',(-6.33169448077,-36.4799878332,2.0724476349));
#64500=CARTESIAN_POINT('Ctrl Pts',(-6.33169448077,-36.5742356128,2.0724476349));
#64501=CARTESIAN_POINT('Ctrl Pts',(-5.99141530911,-36.2742356128,1.9788243735));
#64502=CARTESIAN_POINT('Ctrl Pts',(-6.0819421462,-36.2742356128,1.95259666444));
#64503=CARTESIAN_POINT('Ctrl Pts',(-6.17246898329,-36.3112466293,1.92636895538));
#64504=CARTESIAN_POINT('Ctrl Pts',(-6.2440213753,-36.3857400536,1.90563857988));
#64505=CARTESIAN_POINT('Ctrl Pts',(-6.27957118122,-36.4799878332,1.89533898265));
#64506=CARTESIAN_POINT('Ctrl Pts',(-6.27957118122,-36.5742356128,1.89533898265));
#64507=CARTESIAN_POINT('Ctrl Pts',(-5.97520112534,-36.2742356128,1.92228832367));
#64508=CARTESIAN_POINT('Ctrl Pts',(-6.06583420961,-36.2742356128,1.89643429474));
#64509=CARTESIAN_POINT('Ctrl Pts',(-6.15646729387,-36.3112466293,1.87058026582));
#64510=CARTESIAN_POINT('Ctrl Pts',(-6.2281036639,-36.3857400536,1.85014524757));
#64511=CARTESIAN_POINT('Ctrl Pts',(-6.26369519271,-36.4799878332,1.83999239363));
#64512=CARTESIAN_POINT('Ctrl Pts',(-6.26369519271,-36.5742356128,1.83999239363));
#64513=CARTESIAN_POINT('Ctrl Pts',(-5.9347525703,-36.2742356128,1.77898877676));
#64514=CARTESIAN_POINT('Ctrl Pts',(-6.02559800101,-36.2742356128,1.75388963588));
#64515=CARTESIAN_POINT('Ctrl Pts',(-6.11644343173,-36.3112466293,1.728790495));
#64516=CARTESIAN_POINT('Ctrl Pts',(-6.18824763999,-36.3857400536,1.70895213871));
#64517=CARTESIAN_POINT('Ctrl Pts',(-6.22392255742,-36.4799878332,1.69909572999));
#64518=CARTESIAN_POINT('Ctrl Pts',(-6.22392255742,-36.5742356128,1.69909572999));
#64519=CARTESIAN_POINT('Ctrl Pts',(-5.89729646051,-36.2742356128,1.64334906184));
#64520=CARTESIAN_POINT('Ctrl Pts',(-5.9880924731,-36.2742356128,1.61807905477));
#64521=CARTESIAN_POINT('Ctrl Pts',(-6.0788884857,-36.3112466293,1.5928090477));
#64522=CARTESIAN_POINT('Ctrl Pts',(-6.15065363436,-36.3857400536,1.57283564109));
#64523=CARTESIAN_POINT('Ctrl Pts',(-6.18630914486,-36.4799878332,1.5629121311));
#64524=CARTESIAN_POINT('Ctrl Pts',(-6.18630914486,-36.5742356128,1.5629121311));
#64525=CARTESIAN_POINT('Ctrl Pts',(-5.87402738023,-36.2742356128,1.56021991543));
#64526=CARTESIAN_POINT('Ctrl Pts',(-5.96471053981,-36.2742356128,1.53453784372));
#64527=CARTESIAN_POINT('Ctrl Pts',(-6.0553936994,-36.3112466293,1.508855772));
#64528=CARTESIAN_POINT('Ctrl Pts',(-6.12706965104,-36.3857400536,1.48855667603));
#64529=CARTESIAN_POINT('Ctrl Pts',(-6.16268084229,-36.4799878332,1.47847134219));
#64530=CARTESIAN_POINT('Ctrl Pts',(-6.16268084229,-36.5742356128,1.47847134219));
#64531=CARTESIAN_POINT('Ctrl Pts',(-5.82268928074,-36.2742356128,1.38179028229));
#64532=CARTESIAN_POINT('Ctrl Pts',(-5.91303885618,-36.2742356128,1.35492687511));
#64533=CARTESIAN_POINT('Ctrl Pts',(-6.00338843162,-36.3112466293,1.32806346794));
#64534=CARTESIAN_POINT('Ctrl Pts',(-6.07480071619,-36.3857400536,1.30683063676));
#64535=CARTESIAN_POINT('Ctrl Pts',(-6.11028091149,-36.4799878332,1.29628140149));
#64536=CARTESIAN_POINT('Ctrl Pts',(-6.11028091149,-36.5742356128,1.29628140149));
#64537=CARTESIAN_POINT('Ctrl Pts',(-5.76820785146,-36.2742356128,1.20835208937));
#64538=CARTESIAN_POINT('Ctrl Pts',(-5.85784448561,-36.2742356128,1.17919014597));
#64539=CARTESIAN_POINT('Ctrl Pts',(-5.94748111977,-36.3112466293,1.15002820258));
#64540=CARTESIAN_POINT('Ctrl Pts',(-6.01832989343,-36.3857400536,1.12697860118));
#64541=CARTESIAN_POINT('Ctrl Pts',(-6.05353011961,-36.4799878332,1.11552674054));
#64542=CARTESIAN_POINT('Ctrl Pts',(-6.05353011961,-36.5742356128,1.11552674054));
#64543=CARTESIAN_POINT('Ctrl Pts',(-5.73947450501,-36.2742356128,1.12179370849));
#64544=CARTESIAN_POINT('Ctrl Pts',(-5.82870044481,-36.2742356128,1.09138518818));
#64545=CARTESIAN_POINT('Ctrl Pts',(-5.91792638462,-36.3112466293,1.06097666786));
#64546=CARTESIAN_POINT('Ctrl Pts',(-5.9884505474,-36.3857400536,1.03694177877));
#64547=CARTESIAN_POINT('Ctrl Pts',(-6.02348949244,-36.4799878332,1.02500038208));
#64548=CARTESIAN_POINT('Ctrl Pts',(-6.02348949244,-36.5742356128,1.02500038208));
#64549=CARTESIAN_POINT('Ctrl Pts',(-5.6492991896,-36.2742356128,0.867227348791));
#64550=CARTESIAN_POINT('Ctrl Pts',(-5.73699523894,-36.2742356128,0.832468736018));
#64551=CARTESIAN_POINT('Ctrl Pts',(-5.82469128829,-36.3112466293,0.797710123244));
#64552=CARTESIAN_POINT('Ctrl Pts',(-5.89400622723,-36.3857400536,0.770236926332));
#64553=CARTESIAN_POINT('Ctrl Pts',(-5.92844438446,-36.4799878332,0.756587248033));
#64554=CARTESIAN_POINT('Ctrl Pts',(-5.92844438446,-36.5742356128,0.756587248033));
#64555=CARTESIAN_POINT('Ctrl Pts',(-5.54369220774,-36.2742356128,0.622753928119));
#64556=CARTESIAN_POINT('Ctrl Pts',(-5.62907055641,-36.2742356128,0.582523808606));
#64557=CARTESIAN_POINT('Ctrl Pts',(-5.71444890507,-36.3112466293,0.542293689093));
#64558=CARTESIAN_POINT('Ctrl Pts',(-5.78193193149,-36.3857400536,0.510495804805));
#64559=CARTESIAN_POINT('Ctrl Pts',(-5.8154599322,-36.4799878332,0.494697480486));
#64560=CARTESIAN_POINT('Ctrl Pts',(-5.8154599322,-36.5742356128,0.494697480486));
#64561=CARTESIAN_POINT('Ctrl Pts',(-5.46501384857,-36.2742356128,0.465072251063));
#64562=CARTESIAN_POINT('Ctrl Pts',(-5.54848443428,-36.2742356128,0.420970712728));
#64563=CARTESIAN_POINT('Ctrl Pts',(-5.63195502,-36.3112466293,0.376869174394));
#64564=CARTESIAN_POINT('Ctrl Pts',(-5.69793015283,-36.3857400536,0.342011328363));
#64565=CARTESIAN_POINT('Ctrl Pts',(-5.73070897496,-36.4799878332,0.324692694584));
#64566=CARTESIAN_POINT('Ctrl Pts',(-5.73070897496,-36.5742356128,0.324692694584));
#64567=CARTESIAN_POINT('Ctrl Pts',(-5.29016221704,-36.2742356128,0.160644480083));
#64568=CARTESIAN_POINT('Ctrl Pts',(-5.36921773106,-36.2742356128,0.108867903392));
#64569=CARTESIAN_POINT('Ctrl Pts',(-5.44827324508,-36.3112466293,0.0570913267005));
#64570=CARTESIAN_POINT('Ctrl Pts',(-5.51075870596,-36.3857400536,0.0161671319651));
#64571=CARTESIAN_POINT('Ctrl Pts',(-5.54180373374,-36.4799878332,-0.00416548225244));
#64572=CARTESIAN_POINT('Ctrl Pts',(-5.54180373374,-36.5742356128,-0.00416548225244));
#64573=CARTESIAN_POINT('Ctrl Pts',(-5.08056917549,-36.2742356128,-0.122448531423));
#64574=CARTESIAN_POINT('Ctrl Pts',(-5.15445489674,-36.2742356128,-0.181197969595));
#64575=CARTESIAN_POINT('Ctrl Pts',(-5.22834061799,-36.3112466293,-0.239947407767));
#64576=CARTESIAN_POINT('Ctrl Pts',(-5.28673987564,-36.3857400536,-0.286382951148));
#64577=CARTESIAN_POINT('Ctrl Pts',(-5.31575473071,-36.4799878332,-0.309453801202));
#64578=CARTESIAN_POINT('Ctrl Pts',(-5.31575473071,-36.5742356128,-0.309453801202));
#64579=CARTESIAN_POINT('Ctrl Pts',(-4.96743305836,-36.2742356128,-0.258380923711));
#64580=CARTESIAN_POINT('Ctrl Pts',(-5.03866455064,-36.2742356128,-0.320282770268));
#64581=CARTESIAN_POINT('Ctrl Pts',(-5.10989604293,-36.3112466293,-0.382184616825));
#64582=CARTESIAN_POINT('Ctrl Pts',(-5.1661974009,-36.3857400536,-0.431111821797));
#64583=CARTESIAN_POINT('Ctrl Pts',(-5.19416994037,-36.4799878332,-0.455420621033));
#64584=CARTESIAN_POINT('Ctrl Pts',(-5.19416994037,-36.5742356128,-0.455420621033));
#64585=CARTESIAN_POINT('Ctrl Pts',(-4.46114659269,-36.2742356128,-0.80567930031));
#64586=CARTESIAN_POINT('Ctrl Pts',(-4.52141506071,-36.2742356128,-0.879333647364));
#64587=CARTESIAN_POINT('Ctrl Pts',(-4.58168352872,-36.3112466293,-0.952987994419));
#64588=CARTESIAN_POINT('Ctrl Pts',(-4.62931970603,-36.3857400536,-1.0112043772));
#64589=CARTESIAN_POINT('Ctrl Pts',(-4.65298708463,-36.4799878332,-1.04012836859));
#64590=CARTESIAN_POINT('Ctrl Pts',(-4.65298708463,-36.5742356128,-1.04012836859));
#64591=CARTESIAN_POINT('Ctrl Pts',(-3.8375375961,-36.2742356128,-1.26315776015));
#64592=CARTESIAN_POINT('Ctrl Pts',(-3.88883264536,-36.2742356128,-1.34257410025));
#64593=CARTESIAN_POINT('Ctrl Pts',(-3.94012769463,-36.3112466293,-1.42199044035));
#64594=CARTESIAN_POINT('Ctrl Pts',(-3.98067131041,-36.3857400536,-1.48476108812));
#64595=CARTESIAN_POINT('Ctrl Pts',(-4.00081480904,-36.4799878332,-1.51594782192));
#64596=CARTESIAN_POINT('Ctrl Pts',(-4.00081480904,-36.5742356128,-1.51594782192));
#64597=CARTESIAN_POINT('Ctrl Pts',(-3.32820147129,-36.2742356128,-1.56569218035));
#64598=CARTESIAN_POINT('Ctrl Pts',(-3.37548175785,-36.2742356128,-1.64720794633));
#64599=CARTESIAN_POINT('Ctrl Pts',(-3.42276204441,-36.3112466293,-1.72872371231));
#64600=CARTESIAN_POINT('Ctrl Pts',(-3.46013228594,-36.3857400536,-1.79315379649));
#64601=CARTESIAN_POINT('Ctrl Pts',(-3.47869929762,-36.4799878332,-1.82516492226));
#64602=CARTESIAN_POINT('Ctrl Pts',(-3.47869929762,-36.5742356128,-1.82516492226));
#64603=CARTESIAN_POINT('Ctrl Pts',(-2.8169014355,-36.2742356128,-1.85179112224));
#64604=CARTESIAN_POINT('Ctrl Pts',(-2.8619505579,-36.2742356128,-1.93475206073));
#64605=CARTESIAN_POINT('Ctrl Pts',(-2.90699968031,-36.3112466293,-2.01771299922));
#64606=CARTESIAN_POINT('Ctrl Pts',(-2.94260655437,-36.3857400536,-2.08328527962));
#64607=CARTESIAN_POINT('Ctrl Pts',(-2.96029724575,-36.4799878332,-2.11586399113));
#64608=CARTESIAN_POINT('Ctrl Pts',(-2.96029724575,-36.5742356128,-2.11586399113));
#64609=CARTESIAN_POINT('Ctrl Pts',(-2.29653265536,-36.2742356128,-2.09683653367));
#64610=CARTESIAN_POINT('Ctrl Pts',(-2.33668543274,-36.2742356128,-2.18210316522));
#64611=CARTESIAN_POINT('Ctrl Pts',(-2.37683821013,-36.3112466293,-2.26736979677));
#64612=CARTESIAN_POINT('Ctrl Pts',(-2.40857495654,-36.3857400536,-2.3347645236));
#64613=CARTESIAN_POINT('Ctrl Pts',(-2.42434291535,-36.4799878332,-2.36824865151));
#64614=CARTESIAN_POINT('Ctrl Pts',(-2.42434291535,-36.5742356128,-2.36824865151));
#64615=CARTESIAN_POINT('',(-2.42434411094,-36.5742356128,-2.36824808793));
#64616=CARTESIAN_POINT('Origin',(-2.29743546385133,-36.5721143210983,-2.09875612122949));
#64617=CARTESIAN_POINT('Ctrl Pts',(-6.53914701908,-36.5742356128,2.5806950957));
#64618=CARTESIAN_POINT('Ctrl Pts',(-6.52032174685649,-36.5742356128,2.54570860091162));
#64619=CARTESIAN_POINT('Ctrl Pts',(-6.50258208588932,-36.5742356128,2.51012495658173));
#64620=CARTESIAN_POINT('Ctrl Pts',(-6.48575331803117,-36.5742356128,2.47402330026177));
#64621=CARTESIAN_POINT('Ctrl Pts',(-6.4630511932899,-36.5742356128,2.42532191510686));
#64622=CARTESIAN_POINT('Ctrl Pts',(-6.44200610676348,-36.5742356128,2.37568107869865));
#64623=CARTESIAN_POINT('Ctrl Pts',(-6.42224329823567,-36.5742356128,2.32538225843607));
#64624=CARTESIAN_POINT('Ctrl Pts',(-6.40593172984875,-36.5742356128,2.28386727612268));
#64625=CARTESIAN_POINT('Ctrl Pts',(-6.39049545136789,-36.5742356128,2.24190846192766));
#64626=CARTESIAN_POINT('Ctrl Pts',(-6.37573913119417,-36.5742356128,2.1996479726803));
#64627=CARTESIAN_POINT('Ctrl Pts',(-6.36347989451579,-36.5742356128,2.16453885782453));
#64628=CARTESIAN_POINT('Ctrl Pts',(-6.35169041632424,-36.5742356128,2.12922211872938));
#64629=CARTESIAN_POINT('Ctrl Pts',(-6.34025906051022,-36.5742356128,2.09374334947018));
#64630=CARTESIAN_POINT('Ctrl Pts',(-6.33082632142642,-36.5742356128,2.06446755936433));
#64631=CARTESIAN_POINT('Ctrl Pts',(-6.32163750734452,-36.5742356128,2.03508116248095));
#64632=CARTESIAN_POINT('Ctrl Pts',(-6.31262755192929,-36.5742356128,2.00558278534094));
#64633=CARTESIAN_POINT('Ctrl Pts',(-6.30858018488047,-36.5742356128,1.99233180305214));
#64634=CARTESIAN_POINT('Ctrl Pts',(-6.30456863126258,-36.5742356128,1.97905704388498));
#64635=CARTESIAN_POINT('Ctrl Pts',(-6.3005918933596,-36.5742356128,1.96577575871319));
#64636=CARTESIAN_POINT('Ctrl Pts',(-6.29838938787337,-36.5742356128,1.95841995499448));
#64637=CARTESIAN_POINT('Ctrl Pts',(-6.29619809600555,-36.5742356128,1.95106389512971));
#64638=CARTESIAN_POINT('Ctrl Pts',(-6.29402063675644,-36.5742356128,1.94371992905133));
#64639=CARTESIAN_POINT('Ctrl Pts',(-6.28642198061935,-36.5742356128,1.91809176956468));
#64640=CARTESIAN_POINT('Ctrl Pts',(-6.27898255033723,-36.5742356128,1.89258187965036));
#64641=CARTESIAN_POINT('Ctrl Pts',(-6.27170351106231,-36.5742356128,1.86733365133418));
#64642=CARTESIAN_POINT('Ctrl Pts',(-6.26599905047914,-36.5742356128,1.84754703969699));
#64643=CARTESIAN_POINT('Ctrl Pts',(-6.26039372562493,-36.5742356128,1.82792283460782));
#64644=CARTESIAN_POINT('Ctrl Pts',(-6.25488121131594,-36.5742356128,1.80849670939161));
#64645=CARTESIAN_POINT('Ctrl Pts',(-6.2500278231648,-36.5742356128,1.79139334771996));
#64646=CARTESIAN_POINT('Ctrl Pts',(-6.24524653645831,-36.5742356128,1.77444394963674));
#64647=CARTESIAN_POINT('Ctrl Pts',(-6.24052289064231,-36.5742356128,1.75763262190247));
#64648=CARTESIAN_POINT('Ctrl Pts',(-6.23822440223965,-36.5742356128,1.74945236382733));
#64649=CARTESIAN_POINT('Ctrl Pts',(-6.23593938575314,-36.5742356128,1.74130411709365));
#64650=CARTESIAN_POINT('Ctrl Pts',(-6.23366500246872,-36.5742356128,1.73318159032846));
#64651=CARTESIAN_POINT('Ctrl Pts',(-6.22636543920889,-36.5742356128,1.7071125902799));
#64652=CARTESIAN_POINT('Ctrl Pts',(-6.21917568075214,-36.5742356128,1.68131097734659));
#64653=CARTESIAN_POINT('Ctrl Pts',(-6.21200825626089,-36.5742356128,1.6555906033367));
#64654=CARTESIAN_POINT('Ctrl Pts',(-6.20391515965567,-36.5742356128,1.62654844574745));
#64655=CARTESIAN_POINT('Ctrl Pts',(-6.19584885745646,-36.5742356128,1.5976035761512));
#64656=CARTESIAN_POINT('Ctrl Pts',(-6.18768109822354,-36.5742356128,1.56845713212407));
#64657=CARTESIAN_POINT('Ctrl Pts',(-6.18155527879886,-36.5742356128,1.54659729910371));
#64658=CARTESIAN_POINT('Ctrl Pts',(-6.17537213047874,-36.5742356128,1.52462259154949));
#64659=CARTESIAN_POINT('Ctrl Pts',(-6.16908668276109,-36.5742356128,1.50243475193452));
#64660=CARTESIAN_POINT('Ctrl Pts',(-6.16347986492664,-36.5742356128,1.48264249839117));
#64661=CARTESIAN_POINT('Ctrl Pts',(-6.15779151472513,-36.5742356128,1.46268004755247));
#64662=CARTESIAN_POINT('Ctrl Pts',(-6.15200028273329,-36.5742356128,1.4425146091755));
#64663=CARTESIAN_POINT('Ctrl Pts',(-6.14655542305962,-36.5742356128,1.42355526125516));
#64664=CARTESIAN_POINT('Ctrl Pts',(-6.14101948977268,-36.5742356128,1.40441593963609));
#64665=CARTESIAN_POINT('Ctrl Pts',(-6.13538648341178,-36.5742356128,1.38511197583127));
#64666=CARTESIAN_POINT('Ctrl Pts',(-6.13112388099663,-36.5742356128,1.37050430144494));
#64667=CARTESIAN_POINT('Ctrl Pts',(-6.12680589496271,-36.5742356128,1.35580307774514));
#64668=CARTESIAN_POINT('Ctrl Pts',(-6.12243557585458,-36.5742356128,1.34103577276729));
#64669=CARTESIAN_POINT('Ctrl Pts',(-6.11956939397697,-36.5742356128,1.33135094635955));
#64670=CARTESIAN_POINT('Ctrl Pts',(-6.11668080562675,-36.5742356128,1.32163807644753));
#64671=CARTESIAN_POINT('Ctrl Pts',(-6.11377204094819,-36.5742356128,1.31191000022643));
#64672=CARTESIAN_POINT('Ctrl Pts',(-6.112245556784,-36.5742356128,1.30680482468269));
#64673=CARTESIAN_POINT('Ctrl Pts',(-6.11071368512088,-36.5742356128,1.30169604289404));
#64674=CARTESIAN_POINT('Ctrl Pts',(-6.10917821149739,-36.5742356128,1.29659039499181));
#64675=CARTESIAN_POINT('Ctrl Pts',(-6.09951672157609,-36.5742356128,1.26446469449489));
#64676=CARTESIAN_POINT('Ctrl Pts',(-6.08969773032946,-36.5742356128,1.23241427306604));
#64677=CARTESIAN_POINT('Ctrl Pts',(-6.0796753566568,-36.5742356128,1.20041384530431));
#64678=CARTESIAN_POINT('Ctrl Pts',(-6.06788110894677,-36.5742356128,1.16275600254416));
#64679=CARTESIAN_POINT('Ctrl Pts',(-6.05580535299258,-36.5742356128,1.12516843034084));
#64680=CARTESIAN_POINT('Ctrl Pts',(-6.043399902687,-36.5742356128,1.08767767748112));
#64681=CARTESIAN_POINT('Ctrl Pts',(-6.02909273273903,-36.5742356128,1.04443970067024));
#64682=CARTESIAN_POINT('Ctrl Pts',(-6.01434819002561,-36.5742356128,1.00133527281449));
#64683=CARTESIAN_POINT('Ctrl Pts',(-5.99911484370015,-36.5742356128,0.958441660976139));
#64684=CARTESIAN_POINT('Ctrl Pts',(-5.98578029087872,-36.5742356128,0.920894616450256));
#64685=CARTESIAN_POINT('Ctrl Pts',(-5.97207239113828,-36.5742356128,0.883512523022658));
#64686=CARTESIAN_POINT('Ctrl Pts',(-5.9579543699754,-36.5742356128,0.846312852561985));
#64687=CARTESIAN_POINT('Ctrl Pts',(-5.93414560884613,-36.5742356128,0.783578985126351));
#64688=CARTESIAN_POINT('Ctrl Pts',(-5.9091635512488,-36.5742356128,0.721350159380157));
#64689=CARTESIAN_POINT('Ctrl Pts',(-5.8828848071143,-36.5742356128,0.65973995614056));
#64690=CARTESIAN_POINT('Ctrl Pts',(-5.85568555938991,-36.5742356128,0.595971643176817));
#64691=CARTESIAN_POINT('Ctrl Pts',(-5.82709727613897,-36.5742356128,0.532866069549744));
#64692=CARTESIAN_POINT('Ctrl Pts',(-5.79703519303637,-36.5742356128,0.470527628371927));
#64693=CARTESIAN_POINT('Ctrl Pts',(-5.76636583046652,-36.5742356128,0.40692989803514));
#64694=CARTESIAN_POINT('Ctrl Pts',(-5.73416273827395,-36.5742356128,0.344130578955812));
#64695=CARTESIAN_POINT('Ctrl Pts',(-5.70038666343235,-36.5742356128,0.282218621126629));
#64696=CARTESIAN_POINT('Ctrl Pts',(-5.66556277133928,-36.5742356128,0.218386001474261));
#64697=CARTESIAN_POINT('Ctrl Pts',(-5.62906692815191,-36.5742356128,0.155496671561614));
#64698=CARTESIAN_POINT('Ctrl Pts',(-5.59090689045679,-36.5742356128,0.0936250953297072));
#64699=CARTESIAN_POINT('Ctrl Pts',(-5.57176245947455,-36.5742356128,0.0625848712503234));
#64700=CARTESIAN_POINT('Ctrl Pts',(-5.55219993689747,-36.5742356128,0.031800449018197));
#64701=CARTESIAN_POINT('Ctrl Pts',(-5.53222471364869,-36.5742356128,0.0012791285066921));
#64702=CARTESIAN_POINT('Ctrl Pts',(-5.48858293589753,-36.5742356128,-0.0654037150263174));
#64703=CARTESIAN_POINT('Ctrl Pts',(-5.44296905804018,-36.5742356128,-0.130827416139679));
#64704=CARTESIAN_POINT('Ctrl Pts',(-5.39547709946709,-36.5742356128,-0.194942398547811));
#64705=CARTESIAN_POINT('Ctrl Pts',(-5.34538435552397,-36.5742356128,-0.262568487114894));
#64706=CARTESIAN_POINT('Ctrl Pts',(-5.29320246599191,-36.5742356128,-0.328739090927756));
#64707=CARTESIAN_POINT('Ctrl Pts',(-5.23908298414192,-36.5742356128,-0.393442819708286));
#64708=CARTESIAN_POINT('Ctrl Pts',(-5.17794521020509,-36.5742356128,-0.46653742090972));
#64709=CARTESIAN_POINT('Ctrl Pts',(-5.11433476327847,-36.5742356128,-0.537760505216273));
#64710=CARTESIAN_POINT('Ctrl Pts',(-5.04851964288569,-36.5742356128,-0.607146788830764));
#64711=CARTESIAN_POINT('Ctrl Pts',(-5.00958808586998,-36.5742356128,-0.648190792708977));
#64712=CARTESIAN_POINT('Ctrl Pts',(-4.96988601884903,-36.5742356128,-0.688593005831337));
#64713=CARTESIAN_POINT('Ctrl Pts',(-4.92947512198836,-36.5742356128,-0.728365937491898));
#64714=CARTESIAN_POINT('Ctrl Pts',(-4.86990495862107,-36.5742356128,-0.786995669090893));
#64715=CARTESIAN_POINT('Ctrl Pts',(-4.80879601831302,-36.5742356128,-0.844256936244762));
#64716=CARTESIAN_POINT('Ctrl Pts',(-4.74633115403261,-36.5742356128,-0.900225234060358));
#64717=CARTESIAN_POINT('Ctrl Pts',(-4.69540993206243,-36.5742356128,-0.945850469129586));
#64718=CARTESIAN_POINT('Ctrl Pts',(-4.6435838315632,-36.5742356128,-0.990619526802198));
#64719=CARTESIAN_POINT('Ctrl Pts',(-4.59098076191512,-36.5742356128,-1.03455313729565));
#64720=CARTESIAN_POINT('Ctrl Pts',(-4.5059924451459,-36.5742356128,-1.10553461481043));
#64721=CARTESIAN_POINT('Ctrl Pts',(-4.41897174588524,-36.5742356128,-1.17433980339564));
#64722=CARTESIAN_POINT('Ctrl Pts',(-4.33038782770431,-36.5742356128,-1.24113580021237));
#64723=CARTESIAN_POINT('Ctrl Pts',(-4.24567268322767,-36.5742356128,-1.30501457908094));
#64724=CARTESIAN_POINT('Ctrl Pts',(-4.15952863925796,-36.5742356128,-1.36705753414624));
#64725=CARTESIAN_POINT('Ctrl Pts',(-4.0723260509289,-36.5742356128,-1.42743079196531));
#64726=CARTESIAN_POINT('Ctrl Pts',(-3.99046174632389,-36.5742356128,-1.4841081780705));
#64727=CARTESIAN_POINT('Ctrl Pts',(-3.9076648219601,-36.5742356128,-1.53931520624295));
#64728=CARTESIAN_POINT('Ctrl Pts',(-3.82419873102831,-36.5742356128,-1.59318740760338));
#64729=CARTESIAN_POINT('Ctrl Pts',(-3.74518523665179,-36.5742356128,-1.64418573317157));
#64730=CARTESIAN_POINT('Ctrl Pts',(-3.66557219084631,-36.5742356128,-1.693988594353));
#64731=CARTESIAN_POINT('Ctrl Pts',(-3.58554050425563,-36.5742356128,-1.74269603728047));
#64732=CARTESIAN_POINT('Ctrl Pts',(-3.50892602437149,-36.5742356128,-1.78932376144004));
#64733=CARTESIAN_POINT('Ctrl Pts',(-3.43192795463034,-36.5742356128,-1.83494812133376));
#64734=CARTESIAN_POINT('Ctrl Pts',(-3.35466350954136,-36.5742356128,-1.87963404280889));
#64735=CARTESIAN_POINT('Ctrl Pts',(-3.27816415521591,-36.5742356128,-1.92387747374725));
#64736=CARTESIAN_POINT('Ctrl Pts',(-3.20140389346523,-36.5742356128,-1.96720148429358));
#64737=CARTESIAN_POINT('Ctrl Pts',(-3.1244525163683,-36.5742356128,-2.0096384987399));
#64738=CARTESIAN_POINT('Ctrl Pts',(-3.0852866454685,-36.5742356128,-2.03123762655128));
#64739=CARTESIAN_POINT('Ctrl Pts',(-3.04607053863626,-36.5742356128,-2.05260643753161));
#64740=CARTESIAN_POINT('Ctrl Pts',(-3.00680870232973,-36.5742356128,-2.07374547713585));
#64741=CARTESIAN_POINT('Ctrl Pts',(-2.988900471926,-36.5742356128,-2.08338748136588));
#64742=CARTESIAN_POINT('Ctrl Pts',(-2.97097518539882,-36.5742356128,-2.09298568668701));
#64743=CARTESIAN_POINT('Ctrl Pts',(-2.95303040996166,-36.5742356128,-2.1025412036186));
#64744=CARTESIAN_POINT('Ctrl Pts',(-2.88078777831576,-36.5742356128,-2.14101009905238));
#64745=CARTESIAN_POINT('Ctrl Pts',(-2.80824941916113,-36.5742356128,-2.17878051698545));
#64746=CARTESIAN_POINT('Ctrl Pts',(-2.73544576469779,-36.5742356128,-2.21579026646871));
#64747=CARTESIAN_POINT('Ctrl Pts',(-2.66430005808082,-36.5742356128,-2.25195719789698));
#64748=CARTESIAN_POINT('Ctrl Pts',(-2.59290098389418,-36.5742356128,-2.28739789677643));
#64749=CARTESIAN_POINT('Ctrl Pts',(-2.52123973657706,-36.5742356128,-2.32202099352562));
#64750=CARTESIAN_POINT('Ctrl Pts',(-2.48899587984796,-36.5742356128,-2.33759959720465));
#64751=CARTESIAN_POINT('Ctrl Pts',(-2.45669843912861,-36.5742356128,-2.35301220297855));
#64752=CARTESIAN_POINT('Ctrl Pts',(-2.42434411115899,-36.5742356128,-2.36824808839505));
#64753=CARTESIAN_POINT('Ctrl Pts',(-2.42434398441,-37.9742356128,-2.3682481465));
#64754=CARTESIAN_POINT('Ctrl Pts',(-2.42434398591,-38.0684833924,-2.36824814579));
#64755=CARTESIAN_POINT('Ctrl Pts',(-2.40857608072,-38.1627311721,-2.33476399274));
#64756=CARTESIAN_POINT('Ctrl Pts',(-2.37683944038,-38.2372245963,-2.26736921615));
#64757=CARTESIAN_POINT('Ctrl Pts',(-2.33668679631,-38.2742356128,-2.18210252207));
#64758=CARTESIAN_POINT('Ctrl Pts',(-2.29653415164,-38.2742356128,-2.09683582826));
#64759=CARTESIAN_POINT('Ctrl Pts',(-3.10523376345,-37.9742356128,-2.04761278031));
#64760=CARTESIAN_POINT('Ctrl Pts',(-3.10523328188,-38.0684833917,-2.04761300582));
#64761=CARTESIAN_POINT('Ctrl Pts',(-3.087034044,-38.1627311705,-2.01527377228));
#64762=CARTESIAN_POINT('Ctrl Pts',(-3.05040417654,-38.2372245945,-1.9501832279));
#64763=CARTESIAN_POINT('Ctrl Pts',(-3.00406107947,-38.2742356116,-1.86783163316));
#64764=CARTESIAN_POINT('Ctrl Pts',(-2.95771817057,-38.2742356128,-1.78547994979));
#64765=CARTESIAN_POINT('Ctrl Pts',(-3.75558799721,-37.9742356128,-1.66539056819));
#64766=CARTESIAN_POINT('Ctrl Pts',(-3.75558871127,-38.0684833959,-1.66539023156));
#64767=CARTESIAN_POINT('Ctrl Pts',(-3.73654782615,-38.162731179,-1.63381112995));
#64768=CARTESIAN_POINT('Ctrl Pts',(-3.69822294792,-38.2372246046,-1.5702509984));
#64769=CARTESIAN_POINT('Ctrl Pts',(-3.6497344282,-38.2742356183,-1.48983609251));
#64770=CARTESIAN_POINT('Ctrl Pts',(-3.6012456292,-38.2742356128,-1.409421321));
#64771=CARTESIAN_POINT('Ctrl Pts',(-4.42784969665,-37.9742356128,-1.26351165773));
#64772=CARTESIAN_POINT('Ctrl Pts',(-4.42784946111,-38.0684834383,-1.26351181731));
#64773=CARTESIAN_POINT('Ctrl Pts',(-4.40636826728,-38.1627312638,-1.23261755234));
#64774=CARTESIAN_POINT('Ctrl Pts',(-4.36313251053,-38.2372247045,-1.17043536123));
#64775=CARTESIAN_POINT('Ctrl Pts',(-4.30843157333,-38.2742356849,-1.09176343887));
#64776=CARTESIAN_POINT('Ctrl Pts',(-4.2537307561,-38.2742356128,-1.01309146202));
#64777=CARTESIAN_POINT('Ctrl Pts',(-5.17355249507,-37.9742356128,-0.596349454932));
#64778=CARTESIAN_POINT('Ctrl Pts',(-5.17355255747,-38.0684833803,-0.596349412654));
#64779=CARTESIAN_POINT('Ctrl Pts',(-5.14592211519,-38.1627311477,-0.570516664483));
#64780=CARTESIAN_POINT('Ctrl Pts',(-5.09030925685,-38.2372245677,-0.51852219394));
#64781=CARTESIAN_POINT('Ctrl Pts',(-5.01994878926,-38.2742355937,-0.452739724933));
#64782=CARTESIAN_POINT('Ctrl Pts',(-4.94958828989,-38.2742356128,-0.386957270362));
#64783=CARTESIAN_POINT('Ctrl Pts',(-5.68047245792,-37.9742356128,0.230713175531));
#64784=CARTESIAN_POINT('Ctrl Pts',(-5.68047244139,-38.0684833957,0.23071316433));
#64785=CARTESIAN_POINT('Ctrl Pts',(-5.64814706462,-38.1627311785,0.248875697229));
#64786=CARTESIAN_POINT('Ctrl Pts',(-5.58308461353,-38.2372246039,0.285432101802));
#64787=CARTESIAN_POINT('Ctrl Pts',(-5.50076875003,-38.2742356179,0.331682633922));
#64788=CARTESIAN_POINT('Ctrl Pts',(-5.41845289496,-38.2742356128,0.377933169868));
#64789=CARTESIAN_POINT('Ctrl Pts',(-5.77561843229,-37.9742356128,0.410354854144));
#64790=CARTESIAN_POINT('Ctrl Pts',(-5.77561842674,-38.0684833594,0.410354840082));
#64791=CARTESIAN_POINT('Ctrl Pts',(-5.74243084804,-38.1627311059,0.426883018809));
#64792=CARTESIAN_POINT('Ctrl Pts',(-5.67563300366,-38.2372245184,0.460149908026));
#64793=CARTESIAN_POINT('Ctrl Pts',(-5.59112152855,-38.2742355609,0.50223860778));
#64794=CARTESIAN_POINT('Ctrl Pts',(-5.50661003688,-38.2742356128,0.544327321176));
#64795=CARTESIAN_POINT('Ctrl Pts',(-5.90159361138,-37.9742356128,0.688319077788));
#64796=CARTESIAN_POINT('Ctrl Pts',(-5.90159361416,-38.0684834091,0.688319084849));
#64797=CARTESIAN_POINT('Ctrl Pts',(-5.86735372253,-38.1627312053,0.702481569163));
#64798=CARTESIAN_POINT('Ctrl Pts',(-5.79843783889,-38.2372246355,0.730986909385));
#64799=CARTESIAN_POINT('Ctrl Pts',(-5.71124667074,-38.2742356389,0.767051361344));
#64800=CARTESIAN_POINT('Ctrl Pts',(-5.6240555109,-38.2742356128,0.803115806453));
#64801=CARTESIAN_POINT('Ctrl Pts',(-6.00622257558,-37.9742356128,0.974515968157));
#64802=CARTESIAN_POINT('Ctrl Pts',(-6.00622257418,-38.0684833841,0.974515964611));
#64803=CARTESIAN_POINT('Ctrl Pts',(-5.97128603775,-38.1627311554,0.986759517919));
#64804=CARTESIAN_POINT('Ctrl Pts',(-5.90096799706,-38.2372245767,1.01140256866));
#64805=CARTESIAN_POINT('Ctrl Pts',(-5.81200283764,-38.2742355997,1.04258052978));
#64806=CARTESIAN_POINT('Ctrl Pts',(-5.72303767403,-38.2742356128,1.07375849433));
#64807=CARTESIAN_POINT('Ctrl Pts',(-6.03928188172,-37.9742356128,1.07177315099));
#64808=CARTESIAN_POINT('Ctrl Pts',(-6.03928188245,-38.0684833854,1.07177315347));
#64809=CARTESIAN_POINT('Ctrl Pts',(-6.00415419262,-38.162731158,1.08344922785));
#64810=CARTESIAN_POINT('Ctrl Pts',(-5.93345140837,-38.2372245797,1.1069500878));
#64811=CARTESIAN_POINT('Ctrl Pts',(-5.84399947699,-38.2742356018,1.13668296404));
#64812=CARTESIAN_POINT('Ctrl Pts',(-5.75454754116,-38.2742356128,1.16641584059));
#64813=CARTESIAN_POINT('Ctrl Pts',(-6.11490875363,-37.9742356128,1.3080717033));
#64814=CARTESIAN_POINT('Ctrl Pts',(-6.11490875256,-38.0684834027,1.30807169968));
#64815=CARTESIAN_POINT('Ctrl Pts',(-6.07939173589,-38.1627311927,1.31851561198));
#64816=CARTESIAN_POINT('Ctrl Pts',(-6.00790534004,-38.2372246206,1.33953645854));
#64817=CARTESIAN_POINT('Ctrl Pts',(-5.91746200522,-38.274235629,1.36613166813));
#64818=CARTESIAN_POINT('Ctrl Pts',(-5.82701867689,-38.2742356128,1.39272687728));
#64819=CARTESIAN_POINT('Ctrl Pts',(-6.18342174186,-37.9742356128,1.55058013554));
#64820=CARTESIAN_POINT('Ctrl Pts',(-6.18342174342,-38.0684833774,1.55058014082));
#64821=CARTESIAN_POINT('Ctrl Pts',(-6.14774991166,-38.162731142,1.56044830715));
#64822=CARTESIAN_POINT('Ctrl Pts',(-6.07595191287,-38.2372245609,1.58031032001));
#64823=CARTESIAN_POINT('Ctrl Pts',(-5.9851143313,-38.2742355892,1.60543939017));
#64824=CARTESIAN_POINT('Ctrl Pts',(-5.89427674024,-38.2742356128,1.63056846098));
#64825=CARTESIAN_POINT('Ctrl Pts',(-6.21567787488,-37.9742356128,1.6694593188));
#64826=CARTESIAN_POINT('Ctrl Pts',(-6.21567765711,-38.0684833891,1.66945891565));
#64827=CARTESIAN_POINT('Ctrl Pts',(-6.17998213943,-38.1627311653,1.67922401337));
#64828=CARTESIAN_POINT('Ctrl Pts',(-6.1081367461,-38.2372245883,1.69887910028));
#64829=CARTESIAN_POINT('Ctrl Pts',(-6.01723933466,-38.2742356075,1.72374660724));
#64830=CARTESIAN_POINT('Ctrl Pts',(-5.92634200668,-38.2742356128,1.74861427291));
#64831=CARTESIAN_POINT('Ctrl Pts',(-6.29122760158,-37.9742356128,1.9445646743));
#64832=CARTESIAN_POINT('Ctrl Pts',(-6.29122780783,-38.0684833957,1.94456505612));
#64833=CARTESIAN_POINT('Ctrl Pts',(-6.25561493004,-38.1627311785,1.95469580701));
#64834=CARTESIAN_POINT('Ctrl Pts',(-6.18393533208,-38.2372246039,1.97508586283));
#64835=CARTESIAN_POINT('Ctrl Pts',(-6.09324743523,-38.2742356179,2.00088277762));
#64836=CARTESIAN_POINT('Ctrl Pts',(-6.00255945933,-38.2742356128,2.02667954206));
#64837=CARTESIAN_POINT('Ctrl Pts',(-6.37726427032,-37.9742356128,2.21399278029));
#64838=CARTESIAN_POINT('Ctrl Pts',(-6.37726407498,-38.0684833894,2.21399241868));
#64839=CARTESIAN_POINT('Ctrl Pts',(-6.34224466402,-38.162731166,2.22603592739));
#64840=CARTESIAN_POINT('Ctrl Pts',(-6.27176005687,-38.2372245892,2.25027677467));
#64841=CARTESIAN_POINT('Ctrl Pts',(-6.18258427948,-38.2742356081,2.28094609277));
#64842=CARTESIAN_POINT('Ctrl Pts',(-6.09340857698,-38.2742356128,2.31161555329));
#64843=CARTESIAN_POINT('Ctrl Pts',(-6.42332792062,-37.9742356128,2.34131663126));
#64844=CARTESIAN_POINT('Ctrl Pts',(-6.42332843985,-38.0684833825,2.34131759612));
#64845=CARTESIAN_POINT('Ctrl Pts',(-6.38877124366,-38.1627311522,2.35472949107));
#64846=CARTESIAN_POINT('Ctrl Pts',(-6.31921605307,-38.237224573,2.38172288062));
#64847=CARTESIAN_POINT('Ctrl Pts',(-6.2312157327,-38.2742355973,2.41587387978));
#64848=CARTESIAN_POINT('Ctrl Pts',(-6.14321520267,-38.2742356128,2.45002450227));
#64849=CARTESIAN_POINT('Ctrl Pts',(-6.47655499797,-37.9742356128,2.4643687343));
#64850=CARTESIAN_POINT('Ctrl Pts',(-6.47655499797,-38.0684833924,2.4643687343));
#64851=CARTESIAN_POINT('Ctrl Pts',(-6.44275070506,-38.1627311721,2.47965357706));
#64852=CARTESIAN_POINT('Ctrl Pts',(-6.37471158618,-38.2372245963,2.51041796246));
#64853=CARTESIAN_POINT('Ctrl Pts',(-6.28862967417,-38.2742356128,2.54934051494));
#64854=CARTESIAN_POINT('Ctrl Pts',(-6.20254776231,-38.2742356128,2.5882630677));
#64855=CARTESIAN_POINT('Ctrl Pts',(-6.53914701908,-37.9742356128,2.5806950957));
#64856=CARTESIAN_POINT('Ctrl Pts',(-6.53914701908,-38.0684833924,2.5806950957));
#64857=CARTESIAN_POINT('Ctrl Pts',(-6.50655459783,-38.1627311721,2.59823218268));
#64858=CARTESIAN_POINT('Ctrl Pts',(-6.44095464156,-38.2372245963,2.63352971798));
#64859=CARTESIAN_POINT('Ctrl Pts',(-6.35795872238,-38.2742356128,2.67818754328));
#64860=CARTESIAN_POINT('Ctrl Pts',(-6.2749628032,-38.2742356128,2.72284536858));
#64861=CARTESIAN_POINT('',(-2.42434411094,-37.9742356128,-2.36824808793));
#64862=CARTESIAN_POINT('Ctrl Pts',(-6.53914701908,-37.9742356128,2.5806950957));
#64863=CARTESIAN_POINT('Ctrl Pts',(-6.47656235486,-37.9742356128,2.46438240697));
#64864=CARTESIAN_POINT('Ctrl Pts',(-6.42402346497,-37.9742356128,2.34266436496));
#64865=CARTESIAN_POINT('Ctrl Pts',(-6.3783983006,-37.9742356128,2.21678838042));
#64866=CARTESIAN_POINT('Ctrl Pts',(-6.29416488484,-37.9742356128,1.9543061278));
#64867=CARTESIAN_POINT('Ctrl Pts',(-6.22058475422,-37.9742356128,1.68729407213));
#64868=CARTESIAN_POINT('Ctrl Pts',(-6.19138019874,-37.9742356128,1.57972238661));
#64869=CARTESIAN_POINT('Ctrl Pts',(-6.00694923806,-37.9742356128,0.922077056884));
#64870=CARTESIAN_POINT('Ctrl Pts',(-5.76642241656,-37.9742356128,0.278662479729));
#64871=CARTESIAN_POINT('Ctrl Pts',(-5.47236260901,-37.9742356128,-0.180892800215));
#64872=CARTESIAN_POINT('Ctrl Pts',(-4.83098837638,-37.9742356128,-0.890342468217));
#64873=CARTESIAN_POINT('Ctrl Pts',(-4.05512009519,-37.9742356128,-1.45762154474));
#64874=CARTESIAN_POINT('Ctrl Pts',(-3.70906725492,-37.9742356128,-1.67871445411));
#64875=CARTESIAN_POINT('Ctrl Pts',(-3.24315352431,-37.9742356128,-1.95213056689));
#64876=CARTESIAN_POINT('Ctrl Pts',(-2.77407974243,-37.9742356128,-2.19713947482));
#64877=CARTESIAN_POINT('Ctrl Pts',(-2.65752099961,-37.9742356128,-2.2562168661));
#64878=CARTESIAN_POINT('Ctrl Pts',(-2.54136162566,-37.9742356128,-2.31314371737));
#64879=CARTESIAN_POINT('Ctrl Pts',(-2.42434411094,-37.9742356128,-2.36824808793));
#64880=CARTESIAN_POINT('Origin',(-2.29743788266369,-37.9763569026624,-2.09875497968932));
#64881=CARTESIAN_POINT('Ctrl Pts',(-6.53914701908,-37.9742356128,2.5806950957));
#64882=CARTESIAN_POINT('Ctrl Pts',(-6.53914701908,-36.2942356128,2.5806950957));
#64883=CARTESIAN_POINT('Ctrl Pts',(-6.47656235486,-37.9742356128,2.46438240697));
#64884=CARTESIAN_POINT('Ctrl Pts',(-6.47656235486,-36.2942356128,2.46438240697));
#64885=CARTESIAN_POINT('Ctrl Pts',(-6.42402346497,-37.9742356128,2.34266436496));
#64886=CARTESIAN_POINT('Ctrl Pts',(-6.42402346497,-36.2942356128,2.34266436496));
#64887=CARTESIAN_POINT('Ctrl Pts',(-6.3783983006,-37.9742356128,2.21678838042));
#64888=CARTESIAN_POINT('Ctrl Pts',(-6.3783983006,-36.2942356128,2.21678838042));
#64889=CARTESIAN_POINT('Ctrl Pts',(-6.29416488484,-37.9742356128,1.9543061278));
#64890=CARTESIAN_POINT('Ctrl Pts',(-6.29416488484,-36.2942356128,1.9543061278));
#64891=CARTESIAN_POINT('Ctrl Pts',(-6.22058475422,-37.9742356128,1.68729407213));
#64892=CARTESIAN_POINT('Ctrl Pts',(-6.22058475422,-36.2942356128,1.68729407213));
#64893=CARTESIAN_POINT('Ctrl Pts',(-6.19138019874,-37.9742356128,1.57972238661));
#64894=CARTESIAN_POINT('Ctrl Pts',(-6.19138019874,-36.2942356128,1.57972238661));
#64895=CARTESIAN_POINT('Ctrl Pts',(-6.00694923806,-37.9742356128,0.922077056884));
#64896=CARTESIAN_POINT('Ctrl Pts',(-6.00694923806,-36.2942356128,0.922077056884));
#64897=CARTESIAN_POINT('Ctrl Pts',(-5.76642241656,-37.9742356128,0.278662479729));
#64898=CARTESIAN_POINT('Ctrl Pts',(-5.76642241656,-36.2942356128,0.278662479729));
#64899=CARTESIAN_POINT('Ctrl Pts',(-5.47236260901,-37.9742356128,-0.180892800215));
#64900=CARTESIAN_POINT('Ctrl Pts',(-5.47236260901,-36.2942356128,-0.180892800215));
#64901=CARTESIAN_POINT('Ctrl Pts',(-4.83098837638,-37.9742356128,-0.890342468217));
#64902=CARTESIAN_POINT('Ctrl Pts',(-4.83098837638,-36.2942356128,-0.890342468217));
#64903=CARTESIAN_POINT('Ctrl Pts',(-4.05512009519,-37.9742356128,-1.45762154474));
#64904=CARTESIAN_POINT('Ctrl Pts',(-4.05512009519,-36.2942356128,-1.45762154474));
#64905=CARTESIAN_POINT('Ctrl Pts',(-3.70906725492,-37.9742356128,-1.67871445411));
#64906=CARTESIAN_POINT('Ctrl Pts',(-3.70906725492,-36.2942356128,-1.67871445411));
#64907=CARTESIAN_POINT('Ctrl Pts',(-3.24315352431,-37.9742356128,-1.95213056689));
#64908=CARTESIAN_POINT('Ctrl Pts',(-3.24315352431,-36.2942356128,-1.95213056689));
#64909=CARTESIAN_POINT('Ctrl Pts',(-2.77407974243,-37.9742356128,-2.19713947482));
#64910=CARTESIAN_POINT('Ctrl Pts',(-2.77407974243,-36.2942356128,-2.19713947482));
#64911=CARTESIAN_POINT('Ctrl Pts',(-2.65752099961,-37.9742356128,-2.2562168661));
#64912=CARTESIAN_POINT('Ctrl Pts',(-2.65752099961,-36.2942356128,-2.2562168661));
#64913=CARTESIAN_POINT('Ctrl Pts',(-2.54136162566,-37.9742356128,-2.31314371737));
#64914=CARTESIAN_POINT('Ctrl Pts',(-2.54136162566,-36.2942356128,-2.31314371737));
#64915=CARTESIAN_POINT('Ctrl Pts',(-2.42434411094,-37.9742356128,-2.36824808793));
#64916=CARTESIAN_POINT('Ctrl Pts',(-2.42434411094,-36.2942356128,-2.36824808793));
#64917=CARTESIAN_POINT('',(-2.42434411094,-37.2742356128,-2.36824808793));
#64918=CARTESIAN_POINT('Ctrl Pts',(-2.29653416635,-36.2742356128,-2.09683582206));
#64919=CARTESIAN_POINT('Ctrl Pts',(-2.33668684465,-36.2742356128,-2.18210250012));
#64920=CARTESIAN_POINT('Ctrl Pts',(-2.37683952295,-36.3112466293,-2.26736917817));
#64921=CARTESIAN_POINT('Ctrl Pts',(-2.40857619105,-36.3857400536,-2.33476394176));
#64922=CARTESIAN_POINT('Ctrl Pts',(-2.42434411094,-36.4799878332,-2.36824808793));
#64923=CARTESIAN_POINT('Ctrl Pts',(-2.42434411094,-36.5742356128,-2.36824808793));
#64924=CARTESIAN_POINT('Ctrl Pts',(-2.17844599916,-36.2742356128,-2.1524443704));
#64925=CARTESIAN_POINT('Ctrl Pts',(-2.21652342692,-36.2742356128,-2.23868829852));
#64926=CARTESIAN_POINT('Ctrl Pts',(-2.25460085469,-36.3112466293,-2.32493222664));
#64927=CARTESIAN_POINT('Ctrl Pts',(-2.28469724522,-36.3857400536,-2.39309940847));
#64928=CARTESIAN_POINT('Ctrl Pts',(-2.29965021614,-36.4799878332,-2.42696731985));
#64929=CARTESIAN_POINT('Ctrl Pts',(-2.29965021614,-36.5742356128,-2.42696731985));
#64930=CARTESIAN_POINT('Ctrl Pts',(-2.05865446461,-36.2742356128,-2.20446579111));
#64931=CARTESIAN_POINT('Ctrl Pts',(-2.09463456858,-36.2742356128,-2.29162022708));
#64932=CARTESIAN_POINT('Ctrl Pts',(-2.13061467256,-36.3112466293,-2.37877466305));
#64933=CARTESIAN_POINT('Ctrl Pts',(-2.15905333884,-36.3857400536,-2.44766151009));
#64934=CARTESIAN_POINT('Ctrl Pts',(-2.17318269263,-36.4799878332,-2.48188697706));
#64935=CARTESIAN_POINT('Ctrl Pts',(-2.17318269263,-36.5742356128,-2.48188697706));
#64936=CARTESIAN_POINT('Ctrl Pts',(-1.93731975861,-36.2742356128,-2.25284642822));
#64937=CARTESIAN_POINT('Ctrl Pts',(-1.97117776269,-36.2742356128,-2.3408461829));
#64938=CARTESIAN_POINT('Ctrl Pts',(-2.00503576677,-36.3112466293,-2.42884593757));
#64939=CARTESIAN_POINT('Ctrl Pts',(-2.03179719321,-36.3857400536,-2.49840091092));
#64940=CARTESIAN_POINT('Ctrl Pts',(-2.04509313286,-36.4799878332,-2.53295834717));
#64941=CARTESIAN_POINT('Ctrl Pts',(-2.04509313286,-36.5742356128,-2.53295834717));
#64942=CARTESIAN_POINT('Ctrl Pts',(-1.69184409393,-36.2742356128,-2.34222839622));
#64943=CARTESIAN_POINT('Ctrl Pts',(-1.7214278807,-36.2742356128,-2.4317855696));
#64944=CARTESIAN_POINT('Ctrl Pts',(-1.75101166748,-36.3112466293,-2.52134274297));
#64945=CARTESIAN_POINT('Ctrl Pts',(-1.77439461858,-36.3857400536,-2.59212872651));
#64946=CARTESIAN_POINT('Ctrl Pts',(-1.78601221194,-36.4799878332,-2.62729773286));
#64947=CARTESIAN_POINT('Ctrl Pts',(-1.78601221194,-36.5742356128,-2.62729773286));
#64948=CARTESIAN_POINT('Ctrl Pts',(-1.44144377776,-36.2742356128,-2.41663224395));
#64949=CARTESIAN_POINT('Ctrl Pts',(-1.46665418431,-36.2742356128,-2.50748826439));
#64950=CARTESIAN_POINT('Ctrl Pts',(-1.49186459086,-36.3112466293,-2.59834428482));
#64951=CARTESIAN_POINT('Ctrl Pts',(-1.51179095812,-36.3857400536,-2.67015685));
#64952=CARTESIAN_POINT('Ctrl Pts',(-1.52169099416,-36.4799878332,-2.70583593919));
#64953=CARTESIAN_POINT('Ctrl Pts',(-1.52169099416,-36.5742356128,-2.70583593919));
#64954=CARTESIAN_POINT('Ctrl Pts',(-1.31513154012,-36.2742356128,-2.45004581652));
#64955=CARTESIAN_POINT('Ctrl Pts',(-1.33815301486,-36.2742356128,-2.54148212378));
#64956=CARTESIAN_POINT('Ctrl Pts',(-1.3611744896,-36.3112466293,-2.63291843104));
#64957=CARTESIAN_POINT('Ctrl Pts',(-1.37937038832,-36.3857400536,-2.70518972178));
#64958=CARTESIAN_POINT('Ctrl Pts',(-1.38841117016,-36.4799878332,-2.7410966221));
#64959=CARTESIAN_POINT('Ctrl Pts',(-1.38841117016,-36.5742356128,-2.7410966221));
#64960=CARTESIAN_POINT('Ctrl Pts',(-1.18795712379,-36.2742356128,-2.47960053242));
#64961=CARTESIAN_POINT('Ctrl Pts',(-1.20872995768,-36.2742356128,-2.57155896492));
#64962=CARTESIAN_POINT('Ctrl Pts',(-1.22950279157,-36.3112466293,-2.66351739742));
#64963=CARTESIAN_POINT('Ctrl Pts',(-1.24592181481,-36.3857400536,-2.73620128653));
#64964=CARTESIAN_POINT('Ctrl Pts',(-1.2540791077,-36.4799878332,-2.77231331425));
#64965=CARTESIAN_POINT('Ctrl Pts',(-1.2540791077,-36.5742356128,-2.77231331425));
#64966=CARTESIAN_POINT('Ctrl Pts',(-1.05996478409,-36.2742356128,-2.50526963826));
#64967=CARTESIAN_POINT('Ctrl Pts',(-1.07849731386,-36.2742356128,-2.59767737229));
#64968=CARTESIAN_POINT('Ctrl Pts',(-1.09702984363,-36.3112466293,-2.69008510632));
#64969=CARTESIAN_POINT('Ctrl Pts',(-1.11167795108,-36.3857400536,-2.76312415899));
#64970=CARTESIAN_POINT('Ctrl Pts',(-1.1189556585,-36.4799878332,-2.79941259128));
#64971=CARTESIAN_POINT('Ctrl Pts',(-1.1189556585,-36.5742356128,-2.79941259128));
#64972=CARTESIAN_POINT('',(-1.11895565834,-36.5742356128,-2.79941259037));
#64973=CARTESIAN_POINT('Origin',(-1.06038177374648,-36.572114319719,-2.50734954270403));
#64974=CARTESIAN_POINT('Origin',(-0.445434424830266,-36.5742356128,1.4314036149712));
#64975=CARTESIAN_POINT('Ctrl Pts',(-1.11895565712,-37.9742356128,-2.79941258318));
#64976=CARTESIAN_POINT('Ctrl Pts',(-1.11895565712,-38.0684833925,-2.79941258318));
#64977=CARTESIAN_POINT('Ctrl Pts',(-1.1116780293,-38.1627311721,-2.76312413504));
#64978=CARTESIAN_POINT('Ctrl Pts',(-1.09703008208,-38.2372245964,-2.6900850505));
#64979=CARTESIAN_POINT('Ctrl Pts',(-1.07849775503,-38.2742356129,-2.59767727615));
#64980=CARTESIAN_POINT('Ctrl Pts',(-1.05996542799,-38.2742356128,-2.50526950182));
#64981=CARTESIAN_POINT('Ctrl Pts',(-1.25407581983,-37.9742356128,-2.7723140373));
#64982=CARTESIAN_POINT('Ctrl Pts',(-1.25407581979,-38.0684833925,-2.77231403731));
#64983=CARTESIAN_POINT('Ctrl Pts',(-1.24591947351,-38.1627311723,-2.73620181852));
#64984=CARTESIAN_POINT('Ctrl Pts',(-1.22950248938,-38.2372245966,-2.66351751812));
#64985=CARTESIAN_POINT('Ctrl Pts',(-1.20873217919,-38.274235613,-2.57155857651));
#64986=CARTESIAN_POINT('Ctrl Pts',(-1.18796186904,-38.2742356128,-2.47959963495));
#64987=CARTESIAN_POINT('Ctrl Pts',(-1.38841813634,-37.9742356128,-2.74109509296));
#64988=CARTESIAN_POINT('Ctrl Pts',(-1.38841812984,-38.0684833917,-2.74109509422));
#64989=CARTESIAN_POINT('Ctrl Pts',(-1.37937582186,-38.1627311705,-2.70518850284));
#64990=CARTESIAN_POINT('Ctrl Pts',(-1.36117665871,-38.2372245946,-2.63291787243));
#64991=CARTESIAN_POINT('Ctrl Pts',(-1.33815114202,-38.2742356116,-2.54148238272));
#64992=CARTESIAN_POINT('Ctrl Pts',(-1.31512562779,-38.2742356128,-2.45004689205));
#64993=CARTESIAN_POINT('Ctrl Pts',(-1.52169104358,-37.9742356128,-2.70583567795));
#64994=CARTESIAN_POINT('Ctrl Pts',(-1.52169102758,-38.068483392,-2.70583568235));
#64995=CARTESIAN_POINT('Ctrl Pts',(-1.51179115796,-38.1627311711,-2.67015661522));
#64996=CARTESIAN_POINT('Ctrl Pts',(-1.49186535352,-38.2372245952,-2.59834400459));
#64997=CARTESIAN_POINT('Ctrl Pts',(-1.46665558121,-38.2742356121,-2.50748795926));
#64998=CARTESIAN_POINT('Ctrl Pts',(-1.44144581512,-38.2742356128,-2.41663191191));
#64999=CARTESIAN_POINT('Ctrl Pts',(-1.78601349475,-37.9742356128,-2.62729758713));
#65000=CARTESIAN_POINT('Ctrl Pts',(-1.7860134747,-38.0684833923,-2.62729759371));
#65001=CARTESIAN_POINT('Ctrl Pts',(-1.77439565629,-38.1627311718,-2.59212858833));
#65002=CARTESIAN_POINT('Ctrl Pts',(-1.75101206839,-38.2372245961,-2.52134268314));
#65003=CARTESIAN_POINT('Ctrl Pts',(-1.72142757559,-38.2742356127,-2.4317855694));
#65004=CARTESIAN_POINT('Ctrl Pts',(-1.69184309062,-38.2742356128,-2.34222845301));
#65005=CARTESIAN_POINT('Ctrl Pts',(-2.04509216583,-37.9742356128,-2.53295838102));
#65006=CARTESIAN_POINT('Ctrl Pts',(-2.04509215359,-38.0684833931,-2.53295838601));
#65007=CARTESIAN_POINT('Ctrl Pts',(-2.03179639085,-38.1627311734,-2.49840097113));
#65008=CARTESIAN_POINT('Ctrl Pts',(-2.00503554375,-38.2372245979,-2.42884595021));
#65009=CARTESIAN_POINT('Ctrl Pts',(-1.97117819268,-38.2742356139,-2.34084616804));
#65010=CARTESIAN_POINT('Ctrl Pts',(-1.93732084657,-38.2742356128,-2.25284638431));
#65011=CARTESIAN_POINT('Ctrl Pts',(-2.17317993067,-37.9742356128,-2.48188822357));
#65012=CARTESIAN_POINT('Ctrl Pts',(-2.17317993101,-38.0684833925,-2.48188822361));
#65013=CARTESIAN_POINT('Ctrl Pts',(-2.15905113355,-38.1627311721,-2.44766249585));
#65014=CARTESIAN_POINT('Ctrl Pts',(-2.13061295397,-38.2372245964,-2.37877542164));
#65015=CARTESIAN_POINT('Ctrl Pts',(-2.09463373126,-38.2742356129,-2.29162057324));
#65016=CARTESIAN_POINT('Ctrl Pts',(-2.05865450841,-38.2742356128,-2.2044657248));
#65017=CARTESIAN_POINT('Ctrl Pts',(-2.2996499723,-37.9742356128,-2.42696743467));
#65018=CARTESIAN_POINT('Ctrl Pts',(-2.2996499723,-38.0684833924,-2.42696743467));
#65019=CARTESIAN_POINT('Ctrl Pts',(-2.28469686299,-38.1627311721,-2.39309958844));
#65020=CARTESIAN_POINT('Ctrl Pts',(-2.25460061566,-38.2372245963,-2.32493233923));
#65021=CARTESIAN_POINT('Ctrl Pts',(-2.21652319195,-38.2742356128,-2.23868840917));
#65022=CARTESIAN_POINT('Ctrl Pts',(-2.17844576824,-38.2742356128,-2.15244447914));
#65023=CARTESIAN_POINT('Ctrl Pts',(-2.42434411094,-37.9742356128,-2.36824808793));
#65024=CARTESIAN_POINT('Ctrl Pts',(-2.42434411094,-38.0684833924,-2.36824808793));
#65025=CARTESIAN_POINT('Ctrl Pts',(-2.40857619105,-38.1627311721,-2.33476394176));
#65026=CARTESIAN_POINT('Ctrl Pts',(-2.37683952295,-38.2372245963,-2.26736917817));
#65027=CARTESIAN_POINT('Ctrl Pts',(-2.33668684465,-38.2742356128,-2.18210250012));
#65028=CARTESIAN_POINT('Ctrl Pts',(-2.29653416635,-38.2742356128,-2.09683582206));
#65029=CARTESIAN_POINT('',(-1.11895565834,-37.9742356128,-2.79941259037));
#65030=CARTESIAN_POINT('Origin',(-0.44543442481793,-37.9742356128,1.43140361501597));
#65031=CARTESIAN_POINT('Origin',(-1.06038281360066,-37.9763568917485,-2.50734931579821));
#65032=CARTESIAN_POINT('Ctrl Pts',(-2.42434411094,-37.9742356128,-2.36824808793));
#65033=CARTESIAN_POINT('Ctrl Pts',(-2.42434411094,-36.2942356128,-2.36824808793));
#65034=CARTESIAN_POINT('Ctrl Pts',(-2.1749855611,-37.9742356128,-2.48567278256));
#65035=CARTESIAN_POINT('Ctrl Pts',(-2.1749855611,-36.2942356128,-2.48567278256));
#65036=CARTESIAN_POINT('Ctrl Pts',(-1.91849016776,-37.9742356128,-2.58792345825));
#65037=CARTESIAN_POINT('Ctrl Pts',(-1.91849016776,-36.2942356128,-2.58792345825));
#65038=CARTESIAN_POINT('Ctrl Pts',(-1.65613520407,-37.9742356128,-2.67457823688));
#65039=CARTESIAN_POINT('Ctrl Pts',(-1.65613520407,-36.2942356128,-2.67457823688));
#65040=CARTESIAN_POINT('Ctrl Pts',(-1.38919794322,-37.9742356128,-2.7452152403));
#65041=CARTESIAN_POINT('Ctrl Pts',(-1.38919794322,-36.2942356128,-2.7452152403));
#65042=CARTESIAN_POINT('Ctrl Pts',(-1.11895565834,-37.9742356128,-2.79941259037));
#65043=CARTESIAN_POINT('Ctrl Pts',(-1.11895565834,-36.2942356128,-2.79941259037));
#65044=CARTESIAN_POINT('',(-1.11895565834,-37.2742356128,-2.79941259037));
#65045=CARTESIAN_POINT('Ctrl Pts',(-1.05996499772,-36.2742356128,-2.50526959461));
#65046=CARTESIAN_POINT('Ctrl Pts',(-1.07849746032,-36.2742356128,-2.59767734207));
#65047=CARTESIAN_POINT('Ctrl Pts',(-1.09702992293,-36.3112466293,-2.69008508953));
#65048=CARTESIAN_POINT('Ctrl Pts',(-1.1116779773,-36.3857400536,-2.7631241528));
#65049=CARTESIAN_POINT('Ctrl Pts',(-1.11895565834,-36.4799878332,-2.79941259037));
#65050=CARTESIAN_POINT('Ctrl Pts',(-1.11895565834,-36.5742356128,-2.79941259037));
#65051=CARTESIAN_POINT('Ctrl Pts',(-0.937988992329,-36.2742356128,-2.52973199977));
#65052=CARTESIAN_POINT('Ctrl Pts',(-0.970994450831,-36.2742356128,-2.61923717399));
#65053=CARTESIAN_POINT('Ctrl Pts',(-1.00399990933,-36.3112466293,-2.7087423482));
#65054=CARTESIAN_POINT('Ctrl Pts',(-1.03008741817,-36.3857400536,-2.77948721657));
#65055=CARTESIAN_POINT('Ctrl Pts',(-1.04304862972,-36.4799878332,-2.81463581795));
#65056=CARTESIAN_POINT('Ctrl Pts',(-1.04304862972,-36.5742356128,-2.81463581795));
#65057=CARTESIAN_POINT('Ctrl Pts',(-0.821076773765,-36.2742356128,-2.57798936015));
#65058=CARTESIAN_POINT('Ctrl Pts',(-0.86770125157,-36.2742356128,-2.66182817053));
#65059=CARTESIAN_POINT('Ctrl Pts',(-0.914325729375,-36.3112466293,-2.74566698092));
#65060=CARTESIAN_POINT('Ctrl Pts',(-0.951177701909,-36.3857400536,-2.81193316369));
#65061=CARTESIAN_POINT('Ctrl Pts',(-0.969487096,-36.4799878332,-2.84485658206));
#65062=CARTESIAN_POINT('Ctrl Pts',(-0.969487096,-36.5742356128,-2.84485658206));
#65063=CARTESIAN_POINT('Ctrl Pts',(-0.714826514539,-36.2742356128,-2.64836711386));
#65064=CARTESIAN_POINT('Ctrl Pts',(-0.773989357268,-36.2742356128,-2.72393749335));
#65065=CARTESIAN_POINT('Ctrl Pts',(-0.833152199997,-36.3112466293,-2.79950787283));
#65066=CARTESIAN_POINT('Ctrl Pts',(-0.879914501023,-36.3857400536,-2.85923932342));
#65067=CARTESIAN_POINT('Ctrl Pts',(-0.903147691892,-36.4799878332,-2.88891510279));
#65068=CARTESIAN_POINT('Ctrl Pts',(-0.903147691892,-36.5742356128,-2.88891510279));
#65069=CARTESIAN_POINT('Ctrl Pts',(-0.556197836783,-36.2742356128,-2.80610207254));
#65070=CARTESIAN_POINT('Ctrl Pts',(-0.634097615818,-36.2742356128,-2.86306407596));
#65071=CARTESIAN_POINT('Ctrl Pts',(-0.711997394853,-36.3112466293,-2.92002607939));
#65072=CARTESIAN_POINT('Ctrl Pts',(-0.773569356126,-36.3857400536,-2.9650483506));
#65073=CARTESIAN_POINT('Ctrl Pts',(-0.804160534767,-36.4799878332,-2.98741776081));
#65074=CARTESIAN_POINT('Ctrl Pts',(-0.804160534767,-36.5742356128,-2.98741776081));
#65075=CARTESIAN_POINT('Ctrl Pts',(-0.460021515721,-36.2742356128,-3.00625265901));
#65076=CARTESIAN_POINT('Ctrl Pts',(-0.549251084872,-36.2742356128,-3.03960036015));
#65077=CARTESIAN_POINT('Ctrl Pts',(-0.638480654024,-36.3112466293,-3.0729480613));
#65078=CARTESIAN_POINT('Ctrl Pts',(-0.709007694683,-36.3857400536,-3.09930644297));
#65079=CARTESIAN_POINT('Ctrl Pts',(-0.744048055729,-36.4799878332,-3.11240168856));
#65080=CARTESIAN_POINT('Ctrl Pts',(-0.744048055729,-36.5742356128,-3.11240168856));
#65081=CARTESIAN_POINT('Ctrl Pts',(-0.431626462484,-36.2742356128,-3.09869414072));
#65082=CARTESIAN_POINT('Ctrl Pts',(-0.524172700417,-36.2742356128,-3.12125741915));
#65083=CARTESIAN_POINT('Ctrl Pts',(-0.616718938351,-36.3112466293,-3.14382069757));
#65084=CARTESIAN_POINT('Ctrl Pts',(-0.689867444729,-36.3857400536,-3.16165322052));
#65085=CARTESIAN_POINT('Ctrl Pts',(-0.726210287117,-36.4799878332,-3.17051528659));
#65086=CARTESIAN_POINT('Ctrl Pts',(-0.726210287117,-36.5742356128,-3.17051528659));
#65087=CARTESIAN_POINT('Ctrl Pts',(-0.417273517967,-36.2742356128,-3.19418486389));
#65088=CARTESIAN_POINT('Ctrl Pts',(-0.511521247419,-36.2742356128,-3.2054748872));
#65089=CARTESIAN_POINT('Ctrl Pts',(-0.605768976872,-36.3112466293,-3.21676491052));
#65090=CARTESIAN_POINT('Ctrl Pts',(-0.680262375652,-36.3857400536,-3.22568953251));
#65091=CARTESIAN_POINT('Ctrl Pts',(-0.717273358318,-36.4799878332,-3.23012212425));
#65092=CARTESIAN_POINT('Ctrl Pts',(-0.717273358318,-36.5742356128,-3.23012212425));
#65093=CARTESIAN_POINT('Ctrl Pts',(-0.41727348535,-36.2742356128,-3.28965270484));
#65094=CARTESIAN_POINT('Ctrl Pts',(-0.511521248788,-36.2742356128,-3.28965214022));
#65095=CARTESIAN_POINT('Ctrl Pts',(-0.605769012226,-36.3112466293,-3.28965157561));
#65096=CARTESIAN_POINT('Ctrl Pts',(-0.680262423725,-36.3857400536,-3.28965112934));
#65097=CARTESIAN_POINT('Ctrl Pts',(-0.71727343388,-36.4799878332,-3.28965090762));
#65098=CARTESIAN_POINT('Ctrl Pts',(-0.71727343388,-36.5742356128,-3.28965090762));
#65099=CARTESIAN_POINT('',(-0.717273428011933,-36.5742356128,-3.28965091325724));
#65100=CARTESIAN_POINT('Origin',(-0.419394826283105,-36.5721142715659,-3.28965392582749));
#65101=CARTESIAN_POINT('Ctrl Pts',(-1.11895565834,-36.5742356128,-2.79941259037));
#65102=CARTESIAN_POINT('Ctrl Pts',(-0.984348856958,-36.5742356128,-2.82640811382));
#65103=CARTESIAN_POINT('Ctrl Pts',(-0.858305199948,-36.5742356128,-2.90029762813));
#65104=CARTESIAN_POINT('Ctrl Pts',(-0.764935707726,-36.5742356128,-3.0142516443));
#65105=CARTESIAN_POINT('Ctrl Pts',(-0.717273426056,-36.5742356128,-3.15236381141));
#65106=CARTESIAN_POINT('Ctrl Pts',(-0.717273426056,-36.5742356128,-3.28965091665));
#65107=CARTESIAN_POINT('Ctrl Pts',(-0.717273426048,-37.9742356128,-3.28965091666));
#65108=CARTESIAN_POINT('Ctrl Pts',(-0.717273426048,-38.0684833924,-3.28965091666));
#65109=CARTESIAN_POINT('Ctrl Pts',(-0.680262409542,-38.1627311721,-3.28965091863));
#65110=CARTESIAN_POINT('Ctrl Pts',(-0.605768985255,-38.2372245963,-3.28965092261));
#65111=CARTESIAN_POINT('Ctrl Pts',(-0.51152120564,-38.2742356128,-3.28965092765));
#65112=CARTESIAN_POINT('Ctrl Pts',(-0.417273426023,-38.2742356128,-3.28965093269));
#65113=CARTESIAN_POINT('Ctrl Pts',(-0.717273419177,-37.9742356128,-3.22013522682));
#65114=CARTESIAN_POINT('Ctrl Pts',(-0.717273419176,-38.0684833915,-3.22013522525));
#65115=CARTESIAN_POINT('Ctrl Pts',(-0.680262405917,-38.1627311702,-3.2149372275));
#65116=CARTESIAN_POINT('Ctrl Pts',(-0.6057689684,-38.2372245936,-3.20445862027));
#65117=CARTESIAN_POINT('Ctrl Pts',(-0.51152117913,-38.2742356114,-3.19120816235));
#65118=CARTESIAN_POINT('Ctrl Pts',(-0.41727338975,-38.2742356128,-3.1779577045));
#65119=CARTESIAN_POINT('Ctrl Pts',(-0.729496094549,-37.9742356128,-3.15011357747));
#65120=CARTESIAN_POINT('Ctrl Pts',(-0.729496105134,-38.0684833954,-3.15011362984));
#65121=CARTESIAN_POINT('Ctrl Pts',(-0.693397562691,-38.1627311779,-3.13978673356));
#65122=CARTESIAN_POINT('Ctrl Pts',(-0.620740718576,-38.2372246041,-3.1190259698));
#65123=CARTESIAN_POINT('Ctrl Pts',(-0.528816534376,-38.2742356175,-3.09274944111));
#65124=CARTESIAN_POINT('Ctrl Pts',(-0.436892347128,-38.2742356128,-3.06647289285));
#65125=CARTESIAN_POINT('Ctrl Pts',(-0.753979035124,-37.9742356128,-3.08313484153));
#65126=CARTESIAN_POINT('Ctrl Pts',(-0.753979001334,-38.0684833919,-3.08313487243));
#65127=CARTESIAN_POINT('Ctrl Pts',(-0.719665250065,-38.162731171,-3.06787499254));
#65128=CARTESIAN_POINT('Ctrl Pts',(-0.650603626306,-38.237224595,-3.0371540007));
#65129=CARTESIAN_POINT('Ctrl Pts',(-0.563226878153,-38.274235612,-2.99828919133));
#65130=CARTESIAN_POINT('Ctrl Pts',(-0.475850143134,-38.2742356128,-2.95942436955));
#65131=CARTESIAN_POINT('Ctrl Pts',(-0.823421763256,-37.9742356128,-2.96275807432));
#65132=CARTESIAN_POINT('Ctrl Pts',(-0.823421795982,-38.068483393,-2.96275804439));
#65133=CARTESIAN_POINT('Ctrl Pts',(-0.794269071684,-38.1627311731,-2.93855494734));
#65134=CARTESIAN_POINT('Ctrl Pts',(-0.735589477825,-38.2372245976,-2.88984716793));
#65135=CARTESIAN_POINT('Ctrl Pts',(-0.661350237699,-38.2742356137,-2.8282201644));
#65136=CARTESIAN_POINT('Ctrl Pts',(-0.587110984843,-38.2742356128,-2.7665931729));
#65137=CARTESIAN_POINT('Ctrl Pts',(-0.929441126526,-37.9742356128,-2.87248382646));
#65138=CARTESIAN_POINT('Ctrl Pts',(-0.929441094831,-38.0684833919,-2.87248385545));
#65139=CARTESIAN_POINT('Ctrl Pts',(-0.908153241286,-38.162731171,-2.84158573857));
#65140=CARTESIAN_POINT('Ctrl Pts',(-0.865309169175,-38.2372245951,-2.77938948391));
#65141=CARTESIAN_POINT('Ctrl Pts',(-0.811102469518,-38.274235612,-2.70070256092));
#65142=CARTESIAN_POINT('Ctrl Pts',(-0.756895782199,-38.2742356128,-2.62201562628));
#65143=CARTESIAN_POINT('Ctrl Pts',(-0.988199684399,-37.9742356128,-2.83740276005));
#65144=CARTESIAN_POINT('Ctrl Pts',(-0.98819966439,-38.0684833915,-2.83740274799));
#65145=CARTESIAN_POINT('Ctrl Pts',(-0.971255993125,-38.1627311702,-2.80393138744));
#65146=CARTESIAN_POINT('Ctrl Pts',(-0.937141997279,-38.2372245934,-2.7365650062));
#65147=CARTESIAN_POINT('Ctrl Pts',(-0.893986145252,-38.2742356114,-2.6513331367));
#65148=CARTESIAN_POINT('Ctrl Pts',(-0.850830300288,-38.2742356128,-2.56610127211));
#65149=CARTESIAN_POINT('Ctrl Pts',(-1.05294849577,-37.9742356128,-2.81265039029));
#65150=CARTESIAN_POINT('Ctrl Pts',(-1.05294849577,-38.0684833924,-2.81265039029));
#65151=CARTESIAN_POINT('Ctrl Pts',(-1.04072612657,-38.1627311721,-2.77735371605));
#65152=CARTESIAN_POINT('Ctrl Pts',(-1.01613297159,-38.2372245968,-2.70630905049));
#65153=CARTESIAN_POINT('Ctrl Pts',(-0.985015094421,-38.2742356128,-2.61642532043));
#65154=CARTESIAN_POINT('Ctrl Pts',(-0.953897217654,-38.2742356128,-2.52654158988));
#65155=CARTESIAN_POINT('Ctrl Pts',(-1.11895565834,-37.9742356128,-2.79941259037));
#65156=CARTESIAN_POINT('Ctrl Pts',(-1.11895565834,-38.0684833924,-2.79941259037));
#65157=CARTESIAN_POINT('Ctrl Pts',(-1.1116779773,-38.1627311721,-2.7631241528));
#65158=CARTESIAN_POINT('Ctrl Pts',(-1.09702992293,-38.2372245963,-2.69008508953));
#65159=CARTESIAN_POINT('Ctrl Pts',(-1.07849746032,-38.2742356128,-2.59767734207));
#65160=CARTESIAN_POINT('Ctrl Pts',(-1.05996499772,-38.2742356128,-2.50526959461));
#65161=CARTESIAN_POINT('',(-0.717273426056,-37.9742356128,-3.28965091665));
#65162=CARTESIAN_POINT('Ctrl Pts',(-1.11895565834,-37.9742356128,-2.79941259037));
#65163=CARTESIAN_POINT('Ctrl Pts',(-1.05294849577,-37.9742356128,-2.81265039029));
#65164=CARTESIAN_POINT('Ctrl Pts',(-0.988199684399,-37.9742356128,-2.83740276005));
#65165=CARTESIAN_POINT('Ctrl Pts',(-0.929441126526,-37.9742356128,-2.87248382646));
#65166=CARTESIAN_POINT('Ctrl Pts',(-0.823421763256,-37.9742356128,-2.96275807432));
#65167=CARTESIAN_POINT('Ctrl Pts',(-0.753979035124,-37.9742356128,-3.08313484153));
#65168=CARTESIAN_POINT('Ctrl Pts',(-0.729496094549,-37.9742356128,-3.15011357747));
#65169=CARTESIAN_POINT('Ctrl Pts',(-0.717273419177,-37.9742356128,-3.22013522682));
#65170=CARTESIAN_POINT('Ctrl Pts',(-0.717273426056,-37.9742356128,-3.28965091665));
#65171=CARTESIAN_POINT('Origin',(-0.419394766787071,-37.9763569535626,-3.28965094375126));
#65172=CARTESIAN_POINT('Ctrl Pts',(-1.11895565834,-37.9742356128,-2.79941259037));
#65173=CARTESIAN_POINT('Ctrl Pts',(-1.11895565834,-36.2942356128,-2.79941259037));
#65174=CARTESIAN_POINT('Ctrl Pts',(-0.984348856958,-37.9742356128,-2.82640811382));
#65175=CARTESIAN_POINT('Ctrl Pts',(-0.984348856958,-36.2942356128,-2.82640811382));
#65176=CARTESIAN_POINT('Ctrl Pts',(-0.858305199948,-37.9742356128,-2.90029762813));
#65177=CARTESIAN_POINT('Ctrl Pts',(-0.858305199948,-36.2942356128,-2.90029762813));
#65178=CARTESIAN_POINT('Ctrl Pts',(-0.764935707726,-37.9742356128,-3.0142516443));
#65179=CARTESIAN_POINT('Ctrl Pts',(-0.764935707726,-36.2942356128,-3.0142516443));
#65180=CARTESIAN_POINT('Ctrl Pts',(-0.717273426056,-37.9742356128,-3.15236381141));
#65181=CARTESIAN_POINT('Ctrl Pts',(-0.717273426056,-36.2942356128,-3.15236381141));
#65182=CARTESIAN_POINT('Ctrl Pts',(-0.717273426056,-37.9742356128,-3.28965091665));
#65183=CARTESIAN_POINT('Ctrl Pts',(-0.717273426056,-36.2942356128,-3.28965091665));
#65184=CARTESIAN_POINT('',(-0.717273426056,-37.2742356128,-3.28965091665));
#65185=CARTESIAN_POINT('Origin',(-0.417273426056,-36.5742356128,0.915007091638));
#65186=CARTESIAN_POINT('',(-0.717294771012954,-36.5742356128,-7.94951669056715));
#65187=CARTESIAN_POINT('Ctrl Pts',(-0.717273426055526,-36.5742356127522,
-7.94951682269996));
#65188=CARTESIAN_POINT('Ctrl Pts',(-0.717273426052653,-36.5562023660265,
-7.94949943022529));
#65189=CARTESIAN_POINT('Ctrl Pts',(-0.715643103341005,-36.5381711705819,
-7.94948981501555));
#65190=CARTESIAN_POINT('Ctrl Pts',(-0.712409414919946,-36.5204327497068,
-7.94948727993358));
#65191=CARTESIAN_POINT('Ctrl Pts',(-0.709174428725905,-36.5026872098889,
-7.94948474383421));
#65192=CARTESIAN_POINT('Ctrl Pts',(-0.704334899389936,-36.4852352845449,
-7.94948929354667));
#65193=CARTESIAN_POINT('Ctrl Pts',(-0.697969075237865,-36.4683585495138,
-7.9495002310941));
#65194=CARTESIAN_POINT('Ctrl Pts',(-0.691605209984622,-36.4514870078113,
-7.94951116527583));
#65195=CARTESIAN_POINT('Ctrl Pts',(-0.683716207778636,-36.4351908765912,
-7.94952848336179));
#65196=CARTESIAN_POINT('Ctrl Pts',(-0.674428984546402,-36.4197331249972,
-7.94955148801929));
#65197=CARTESIAN_POINT('Ctrl Pts',(-0.665142406327905,-36.4042764469708,
-7.94957449107908));
#65198=CARTESIAN_POINT('Ctrl Pts',(-0.654458114349865,-36.389658560481,
-7.94960317992055));
#65199=CARTESIAN_POINT('Ctrl Pts',(-0.642547746664798,-36.3761157488943,
-7.94963685735628));
#65200=CARTESIAN_POINT('Ctrl Pts',(-0.63832252716711,-36.3713114176525,
-7.94964880447344));
#65201=CARTESIAN_POINT('Ctrl Pts',(-0.633943394736352,-36.366642101442,
-7.94966137939795));
#65202=CARTESIAN_POINT('Ctrl Pts',(-0.629419239159912,-36.3621173580875,
-7.94967455100391));
#65203=CARTESIAN_POINT('Ctrl Pts',(-0.616649081950513,-36.34934554178,-7.9497117299815));
#65204=CARTESIAN_POINT('Ctrl Pts',(-0.60272441955601,-36.3377319027218,
-7.94975346407593));
#65205=CARTESIAN_POINT('Ctrl Pts',(-0.587870725940692,-36.327463326528,
-7.9497985353943));
#65206=CARTESIAN_POINT('Ctrl Pts',(-0.573010913676518,-36.3171905204226,
-7.9498436252788));
#65207=CARTESIAN_POINT('Ctrl Pts',(-0.557221806446512,-36.3082642321724,
-7.9498920551372));
#65208=CARTESIAN_POINT('Ctrl Pts',(-0.540758644704151,-36.3008285887949,
-7.94994260557092));
#65209=CARTESIAN_POINT('Ctrl Pts',(-0.524300920430384,-36.2933954012688,
-7.9499931393088));
#65210=CARTESIAN_POINT('Ctrl Pts',(-0.507170142757527,-36.2874521238513,
-7.95004579222147));
#65211=CARTESIAN_POINT('Ctrl Pts',(-0.489642808887459,-36.2830953159867,
-7.95009934611819));
#65212=CARTESIAN_POINT('Ctrl Pts',(-0.47211842679632,-36.2787392418523,
-7.95015289099589));
#65213=CARTESIAN_POINT('Ctrl Pts',(-0.454198211897778,-36.2759692553201,
-7.95020733655421));
#65214=CARTESIAN_POINT('Ctrl Pts',(-0.436171421743446,-36.274831428195,
-7.95026146521776));
#65215=CARTESIAN_POINT('Ctrl Pts',(-0.429888168625485,-36.2744348375779,
-7.95028033180971));
#65216=CARTESIAN_POINT('Ctrl Pts',(-0.423592041068198,-36.2742360758603,
-7.95029915990285));
#65217=CARTESIAN_POINT('Ctrl Pts',(-0.417295449967826,-36.2742356136084,
-7.95031789793937));
#65218=CARTESIAN_POINT('',(-0.717273426056,-36.5742356128,-5.61958386968));
#65219=CARTESIAN_POINT('Origin',(-0.417273426056,-37.9742356128,0.916320001688));
#65220=CARTESIAN_POINT('',(-0.717273426055838,-37.9742356128056,-7.94951682185356));
#65221=CARTESIAN_POINT('',(-0.717273426056,-37.9742356128,-5.61958386968));
#65222=CARTESIAN_POINT('Ctrl Pts',(-0.417297207529238,-38.2742356118574,
-7.95031787674147));
#65223=CARTESIAN_POINT('Ctrl Pts',(-0.435362516829087,-38.2742341797918,
-7.95026423190646));
#65224=CARTESIAN_POINT('Ctrl Pts',(-0.453423450071235,-38.2725966404015,
-7.95020987106186));
#65225=CARTESIAN_POINT('Ctrl Pts',(-0.471188408770116,-38.269351140414,
-7.95015599844639));
#65226=CARTESIAN_POINT('Ctrl Pts',(-0.488964591978895,-38.2661035898084,
-7.95010209179235));
#65227=CARTESIAN_POINT('Ctrl Pts',(-0.50644382759733,-38.2612461595882,
-7.95004867398459));
#65228=CARTESIAN_POINT('Ctrl Pts',(-0.523343807223555,-38.2548582673361,
-7.94999695154591));
#65229=CARTESIAN_POINT('Ctrl Pts',(-0.540240303205797,-38.2484716918395,
-7.94994523976893));
#65230=CARTESIAN_POINT('Ctrl Pts',(-0.556557214267629,-38.2405555058911,
-7.94989522266216));
#65231=CARTESIAN_POINT('Ctrl Pts',(-0.572031007252925,-38.2312377354798,
-7.94984810600243));
#65232=CARTESIAN_POINT('Ctrl Pts',(-0.587504862496621,-38.2219199275787,
-7.94980098915313));
#65233=CARTESIAN_POINT('Ctrl Pts',(-0.602135070451866,-38.2112008365223,
-7.94975677277421));
#65234=CARTESIAN_POINT('Ctrl Pts',(-0.615684888811112,-38.1992531486659,
-7.94971666265708));
#65235=CARTESIAN_POINT('Ctrl Pts',(-0.620396768694504,-38.195098401453,
-7.94970271456943));
#65236=CARTESIAN_POINT('Ctrl Pts',(-0.624978274211824,-38.1907954572478,
-7.94968926303764));
#65237=CARTESIAN_POINT('Ctrl Pts',(-0.629420380828565,-38.1863527256893,
-7.94967635876712));
#65238=CARTESIAN_POINT('Ctrl Pts',(-0.642172077260688,-38.1735992352735,
-7.94963931523024));
#65239=CARTESIAN_POINT('Ctrl Pts',(-0.65376871421763,-38.1596947618457,
-7.94960697677183));
#65240=CARTESIAN_POINT('Ctrl Pts',(-0.664024067325533,-38.1448642183526,
-7.94958002984277));
#65241=CARTESIAN_POINT('Ctrl Pts',(-0.674284581348108,-38.1300262115211,
-7.94955306935291));
#65242=CARTESIAN_POINT('Ctrl Pts',(-0.683202112686164,-38.1142617086487,
-7.94953150582025));
#65243=CARTESIAN_POINT('Ctrl Pts',(-0.690633204454852,-38.0978253840331,
-7.94951602673255));
#65244=CARTESIAN_POINT('Ctrl Pts',(-0.698062440582742,-38.0813931637827,
-7.94950055151018));
#65245=CARTESIAN_POINT('Ctrl Pts',(-0.704005730097513,-38.0642900186617,
-7.94949115769443));
#65246=CARTESIAN_POINT('Ctrl Pts',(-0.708367224207067,-38.0467918025958,
-7.94948853225816));
#65247=CARTESIAN_POINT('Ctrl Pts',(-0.712728772489379,-38.02929336919,-7.94948590678928));
#65248=CARTESIAN_POINT('Ctrl Pts',(-0.715508335709052,-38.0114004503762,
-7.94949004986802));
#65249=CARTESIAN_POINT('Ctrl Pts',(-0.716660575355175,-37.9934015939698,
-7.94950164849284));
#65250=CARTESIAN_POINT('Ctrl Pts',(-0.717068990960827,-37.9870218327239,
-7.94950575966832));
#65251=CARTESIAN_POINT('Ctrl Pts',(-0.717273426055341,-37.9806288349119,
-7.94951080753942));
#65252=CARTESIAN_POINT('Ctrl Pts',(-0.717273426055477,-37.9742356128064,
-7.9495168227));
#65253=CARTESIAN_POINT('Origin',(-0.717273426056,-38.2742356128,-3.28965091665));
#65254=CARTESIAN_POINT('',(-0.717273426056,-37.2742356128,-7.9495168227));
#65255=CARTESIAN_POINT('Ctrl Pts',(-0.417871464025,-36.2742356128,-7.90065580382));
#65256=CARTESIAN_POINT('Ctrl Pts',(-0.512080830433,-36.2742356128,-7.90334683551));
#65257=CARTESIAN_POINT('Ctrl Pts',(-0.606290196842,-36.3112466293,-7.90603786721));
#65258=CARTESIAN_POINT('Ctrl Pts',(-0.680753259338,-36.3857400536,-7.90816485807));
#65259=CARTESIAN_POINT('Ctrl Pts',(-0.717749191014,-36.4799878332,-7.90922162374));
#65260=CARTESIAN_POINT('Ctrl Pts',(-0.717749191014,-36.5742356128,-7.90922162374));
#65261=CARTESIAN_POINT('Ctrl Pts',(-0.411668939385,-36.2742356128,-8.11771935816));
#65262=CARTESIAN_POINT('Ctrl Pts',(-0.506253640511,-36.2742356128,-8.10730633567));
#65263=CARTESIAN_POINT('Ctrl Pts',(-0.600838341638,-36.3112466293,-8.09689331319));
#65264=CARTESIAN_POINT('Ctrl Pts',(-0.675598077836,-36.3857400536,-8.08866280292));
#65265=CARTESIAN_POINT('Ctrl Pts',(-0.712741393888,-36.4799878332,-8.08457367815));
#65266=CARTESIAN_POINT('Ctrl Pts',(-0.712741393888,-36.5742356128,-8.08457367815));
#65267=CARTESIAN_POINT('Ctrl Pts',(-0.446634901181,-36.2742356128,-8.34322072055));
#65268=CARTESIAN_POINT('Ctrl Pts',(-0.538971580196,-36.2742356128,-8.31457120306));
#65269=CARTESIAN_POINT('Ctrl Pts',(-0.631308259211,-36.3112466293,-8.28592168556));
#65270=CARTESIAN_POINT('Ctrl Pts',(-0.704291136778,-36.3857400536,-8.26327720324));
#65271=CARTESIAN_POINT('Ctrl Pts',(-0.74055167906,-36.4799878332,-8.25202647401));
#65272=CARTESIAN_POINT('Ctrl Pts',(-0.74055167906,-36.5742356128,-8.25202647401));
#65273=CARTESIAN_POINT('Ctrl Pts',(-0.527277494643,-36.2742356128,-8.55090781155));
#65274=CARTESIAN_POINT('Ctrl Pts',(-0.614087616783,-36.2742356128,-8.51039722073));
#65275=CARTESIAN_POINT('Ctrl Pts',(-0.700897738923,-36.3112466293,-8.46988662992));
#65276=CARTESIAN_POINT('Ctrl Pts',(-0.769512681606,-36.3857400536,-8.43786699893));
#65277=CARTESIAN_POINT('Ctrl Pts',(-0.803602695624,-36.4799878332,-8.42195859603));
#65278=CARTESIAN_POINT('Ctrl Pts',(-0.803602695624,-36.5742356128,-8.42195859603));
#65279=CARTESIAN_POINT('Ctrl Pts',(-0.799039246885,-36.2742356128,-8.98598340477));
#65280=CARTESIAN_POINT('Ctrl Pts',(-0.86757857227,-36.2742356128,-8.91521826287));
#65281=CARTESIAN_POINT('Ctrl Pts',(-0.936117897654,-36.3112466293,-8.84445312098));
#65282=CARTESIAN_POINT('Ctrl Pts',(-0.990291056463,-36.3857400536,-8.78852045906));
#65283=CARTESIAN_POINT('Ctrl Pts',(-1.01720669551,-36.4799878332,-8.76073096214));
#65284=CARTESIAN_POINT('Ctrl Pts',(-1.01720669551,-36.5742356128,-8.76073096214));
#65285=CARTESIAN_POINT('Ctrl Pts',(-1.23565010735,-36.2742356128,-9.26373079525));
#65286=CARTESIAN_POINT('Ctrl Pts',(-1.27482326726,-36.2742356128,-9.17557264423));
#65287=CARTESIAN_POINT('Ctrl Pts',(-1.31399642717,-36.3112466293,-9.08741449321));
#65288=CARTESIAN_POINT('Ctrl Pts',(-1.3449592797,-36.3857400536,-9.01773419077));
#65289=CARTESIAN_POINT('Ctrl Pts',(-1.36034214807,-36.4799878332,-8.98311468508));
#65290=CARTESIAN_POINT('Ctrl Pts',(-1.36034214807,-36.5742356128,-8.98311468508));
#65291=CARTESIAN_POINT('Ctrl Pts',(-1.51660510295,-36.2742356128,-9.35601196175));
#65292=CARTESIAN_POINT('Ctrl Pts',(-1.53690836451,-36.2742356128,-9.2608811536));
#65293=CARTESIAN_POINT('Ctrl Pts',(-1.55721162606,-36.3112466293,-9.16575034545));
#65294=CARTESIAN_POINT('Ctrl Pts',(-1.573257749,-36.3857400536,-9.09055929278));
#65295=CARTESIAN_POINT('Ctrl Pts',(-1.5812323917,-36.4799878332,-9.0532011946));
#65296=CARTESIAN_POINT('Ctrl Pts',(-1.5812323917,-36.5742356128,-9.0532011946));
#65297=CARTESIAN_POINT('Ctrl Pts',(-1.80824865356,-36.2742356128,-9.37150440154));
#65298=CARTESIAN_POINT('Ctrl Pts',(-1.80877064489,-36.2742356128,-9.27537219373));
#65299=CARTESIAN_POINT('Ctrl Pts',(-1.80929263621,-36.3112466293,-9.17923998592));
#65300=CARTESIAN_POINT('Ctrl Pts',(-1.80970626455,-36.3857400536,-9.10325689802));
#65301=CARTESIAN_POINT('Ctrl Pts',(-1.80991020356,-36.4799878332,-9.06550608028));
#65302=CARTESIAN_POINT('Ctrl Pts',(-1.80991020356,-36.5742356128,-9.06550608028));
#65303=CARTESIAN_POINT('Ctrl Pts',(-2.08574139369,-36.2742356128,-9.31728165018));
#65304=CARTESIAN_POINT('Ctrl Pts',(-2.06766705511,-36.2742356128,-9.22478320569));
#65305=CARTESIAN_POINT('Ctrl Pts',(-2.04959271653,-36.3112466293,-9.13228476119));
#65306=CARTESIAN_POINT('Ctrl Pts',(-2.03530676328,-36.3857400536,-9.059174011));
#65307=CARTESIAN_POINT('Ctrl Pts',(-2.02820898712,-36.4799878332,-9.02284995679));
#65308=CARTESIAN_POINT('Ctrl Pts',(-2.02820898712,-36.5742356128,-9.02284995679));
#65309=CARTESIAN_POINT('Ctrl Pts',(-0.717294771012954,-36.5742356128,-7.94951669056715));
#65310=CARTESIAN_POINT('Ctrl Pts',(-0.717469199646846,-36.5742356128,-7.97769417776938));
#65311=CARTESIAN_POINT('Ctrl Pts',(-0.718686505327239,-36.5742356128,-8.00568861695275));
#65312=CARTESIAN_POINT('Ctrl Pts',(-0.72096154011341,-36.5742356128,-8.03353757677499));
#65313=CARTESIAN_POINT('Ctrl Pts',(-0.723452189808266,-36.5742356128,-8.06402590324145));
#65314=CARTESIAN_POINT('Ctrl Pts',(-0.727210703773945,-36.5742356128,-8.09433991822543));
#65315=CARTESIAN_POINT('Ctrl Pts',(-0.732240265268736,-36.5742356128,-8.12446475504702));
#65316=CARTESIAN_POINT('Ctrl Pts',(-0.737584387333829,-36.5742356128,-8.15647366980674));
#65317=CARTESIAN_POINT('Ctrl Pts',(-0.744363567783376,-36.5742356128,-8.18826835117234));
#65318=CARTESIAN_POINT('Ctrl Pts',(-0.752562528474982,-36.5742356128,-8.21976675650004));
#65319=CARTESIAN_POINT('Ctrl Pts',(-0.761700247367715,-36.5742356128,-8.25487164165317));
#65320=CARTESIAN_POINT('Ctrl Pts',(-0.772601684950244,-36.5742356128,-8.28960751029073));
#65321=CARTESIAN_POINT('Ctrl Pts',(-0.785220319760699,-36.5742356128,-8.32379577982941));
#65322=CARTESIAN_POINT('Ctrl Pts',(-0.80131191002952,-36.5742356128,-8.36739349334441));
#65323=CARTESIAN_POINT('Ctrl Pts',(-0.820197223142365,-36.5742356128,-8.41009700371508));
#65324=CARTESIAN_POINT('Ctrl Pts',(-0.841726991467189,-36.5742356128,-8.45146835090127));
#65325=CARTESIAN_POINT('Ctrl Pts',(-0.85905852894392,-36.5742356128,-8.48477242753611));
#65326=CARTESIAN_POINT('Ctrl Pts',(-0.878102400020843,-36.5742356128,-8.5172097589679));
#65327=CARTESIAN_POINT('Ctrl Pts',(-0.898758903658759,-36.5742356128,-8.54857028838719));
#65328=CARTESIAN_POINT('Ctrl Pts',(-0.916170691277028,-36.5742356128,-8.57500471734074));
#65329=CARTESIAN_POINT('Ctrl Pts',(-0.934727842012251,-36.5742356128,-8.60067345421032));
#65330=CARTESIAN_POINT('Ctrl Pts',(-0.954362786820594,-36.5742356128,-8.62548528033089));
#65331=CARTESIAN_POINT('Ctrl Pts',(-0.973577822556822,-36.5742356128,-8.64976648561266));
#65332=CARTESIAN_POINT('Ctrl Pts',(-0.993824890950002,-36.5742356128,-8.67322601345517));
#65333=CARTESIAN_POINT('Ctrl Pts',(-1.01503616875631,-36.5742356128,-8.69582657056637));
#65334=CARTESIAN_POINT('Ctrl Pts',(-1.0434088924849,-36.5742356128,-8.72605762825577));
#65335=CARTESIAN_POINT('Ctrl Pts',(-1.07350815510844,-36.5742356128,-8.75475646899135));
#65336=CARTESIAN_POINT('Ctrl Pts',(-1.10513647482402,-36.5742356128,-8.78168472107411));
#65337=CARTESIAN_POINT('Ctrl Pts',(-1.13768537200219,-36.5742356128,-8.80939674991761));
#65338=CARTESIAN_POINT('Ctrl Pts',(-1.1718534896272,-36.5742356128,-8.83523358574093));
#65339=CARTESIAN_POINT('Ctrl Pts',(-1.20740369439064,-36.5742356128,-8.85898666122346));
#65340=CARTESIAN_POINT('Ctrl Pts',(-1.24369561876335,-36.5742356128,-8.88323532096443));
#65341=CARTESIAN_POINT('Ctrl Pts',(-1.2814276875808,-36.5742356128,-8.90531243574938));
#65342=CARTESIAN_POINT('Ctrl Pts',(-1.32032791047747,-36.5742356128,-8.92504834875626));
#65343=CARTESIAN_POINT('Ctrl Pts',(-1.36014940215674,-36.5742356128,-8.94525166475457));
#65344=CARTESIAN_POINT('Ctrl Pts',(-1.40119477440393,-36.5742356128,-8.96300167001931));
#65345=CARTESIAN_POINT('Ctrl Pts',(-1.44315545812899,-36.5742356128,-8.9781692782255));
#65346=CARTESIAN_POINT('Ctrl Pts',(-1.48624235752379,-36.5742356128,-8.99374398175327));
#65347=CARTESIAN_POINT('Ctrl Pts',(-1.53029404515485,-36.5742356128,-9.00659593404456));
#65348=CARTESIAN_POINT('Ctrl Pts',(-1.57496335937971,-36.5742356128,-9.01663882853403));
#65349=CARTESIAN_POINT('Ctrl Pts',(-1.62168047791899,-36.5742356128,-9.02714212594264));
#65350=CARTESIAN_POINT('Ctrl Pts',(-1.66907275594992,-36.5742356128,-9.03457295234747));
#65351=CARTESIAN_POINT('Ctrl Pts',(-1.71673443676159,-36.5742356128,-9.03888917782942));
#65352=CARTESIAN_POINT('Ctrl Pts',(-1.76580780739923,-36.5742356128,-9.04333324545826));
#65353=CARTESIAN_POINT('Ctrl Pts',(-1.8151662456494,-36.5742356128,-9.04447577049441));
#65354=CARTESIAN_POINT('Ctrl Pts',(-1.86436515483982,-36.5742356128,-9.04232661394204));
#65355=CARTESIAN_POINT('Ctrl Pts',(-1.9156186980022,-36.5742356128,-9.04008770478873));
#65356=CARTESIAN_POINT('Ctrl Pts',(-1.96669841756014,-36.5742356128,-9.03427676321613));
#65357=CARTESIAN_POINT('Ctrl Pts',(-2.01710937080252,-36.5742356128,-9.02496003509282));
#65358=CARTESIAN_POINT('Ctrl Pts',(-2.02081291067215,-36.5742356128,-9.02427556332945));
#65359=CARTESIAN_POINT('Ctrl Pts',(-2.02451284712871,-36.5742356128,-9.02357219170736));
#65360=CARTESIAN_POINT('Ctrl Pts',(-2.02820898712,-36.5742356128,-9.02284995679));
#65361=CARTESIAN_POINT('Ctrl Pts',(-2.02820898715,-37.9742356128,-9.02284995683));
#65362=CARTESIAN_POINT('Ctrl Pts',(-2.02820898715,-38.0684833924,-9.02284995683));
#65363=CARTESIAN_POINT('Ctrl Pts',(-2.03530687718,-38.162731172,-9.05917398875));
#65364=CARTESIAN_POINT('Ctrl Pts',(-2.0495930596,-38.2372245963,-9.13228469408));
#65365=CARTESIAN_POINT('Ctrl Pts',(-2.06766768814,-38.2742356128,-9.22478308183));
#65366=CARTESIAN_POINT('Ctrl Pts',(-2.08574231668,-38.2742356128,-9.3172814696));
#65367=CARTESIAN_POINT('Ctrl Pts',(-1.83318359957,-37.9742356128,-9.06095854776));
#65368=CARTESIAN_POINT('Ctrl Pts',(-1.83318360004,-38.0684833904,-9.06095854767));
#65369=CARTESIAN_POINT('Ctrl Pts',(-1.83376258883,-38.1627311679,-9.09855639141));
#65370=CARTESIAN_POINT('Ctrl Pts',(-1.83492595186,-38.2372245913,-9.17423135128));
#65371=CARTESIAN_POINT('Ctrl Pts',(-1.83639865331,-38.2742356096,-9.26997381923));
#65372=CARTESIAN_POINT('Ctrl Pts',(-1.83787135482,-38.2742356128,-9.36571628839));
#65373=CARTESIAN_POINT('Ctrl Pts',(-1.62996049743,-37.9742356128,-9.05518464578));
#65374=CARTESIAN_POINT('Ctrl Pts',(-1.62996053955,-38.068483395,-9.05518463237));
#65375=CARTESIAN_POINT('Ctrl Pts',(-1.62363224748,-38.1627311772,-9.09260850541));
#65376=CARTESIAN_POINT('Ctrl Pts',(-1.61089799618,-38.2372246026,-9.16793230913));
#65377=CARTESIAN_POINT('Ctrl Pts',(-1.59478556452,-38.2742356169,-9.26323093271));
#65378=CARTESIAN_POINT('Ctrl Pts',(-1.57867311595,-38.2742356128,-9.35852956011));
#65379=CARTESIAN_POINT('Ctrl Pts',(-1.43126328637,-37.9742356128,-9.0035760363));
#65380=CARTESIAN_POINT('Ctrl Pts',(-1.43126339204,-38.0684833845,-9.00357619207));
#65381=CARTESIAN_POINT('Ctrl Pts',(-1.41826547793,-38.1627311561,-9.03899098571));
#65382=CARTESIAN_POINT('Ctrl Pts',(-1.39210322077,-38.2372245775,-9.11027159813));
#65383=CARTESIAN_POINT('Ctrl Pts',(-1.35900343843,-38.2742356003,-9.20045442478));
#65384=CARTESIAN_POINT('Ctrl Pts',(-1.3259036101,-38.2742356128,-9.2906371902));
#65385=CARTESIAN_POINT('Ctrl Pts',(-1.07356983998,-37.9742356128,-8.81183251553));
#65386=CARTESIAN_POINT('Ctrl Pts',(-1.07356973553,-38.0684834003,-8.81183236157));
#65387=CARTESIAN_POINT('Ctrl Pts',(-1.04853912901,-38.1627311879,-8.84130344029));
#65388=CARTESIAN_POINT('Ctrl Pts',(-0.998159990023,-38.237224615,-8.90062099705));
#65389=CARTESIAN_POINT('Ctrl Pts',(-0.934420934844,-38.2742356252,-8.97566868954));
#65390=CARTESIAN_POINT('Ctrl Pts',(-0.870681925128,-38.2742356128,-9.05071644255));
#65391=CARTESIAN_POINT('Ctrl Pts',(-0.831386669736,-37.9742356128,-8.48987492086));
#65392=CARTESIAN_POINT('Ctrl Pts',(-0.831386772977,-38.0684833846,-8.48987507304));
#65393=CARTESIAN_POINT('Ctrl Pts',(-0.798242271358,-38.1627311564,-8.50804339173));
#65394=CARTESIAN_POINT('Ctrl Pts',(-0.731530250254,-38.2372245779,-8.54461138493));
#65395=CARTESIAN_POINT('Ctrl Pts',(-0.647127613959,-38.2742356006,-8.59087641987));
#65396=CARTESIAN_POINT('Ctrl Pts',(-0.562724932724,-38.2742356128,-8.63714139499));
#65397=CARTESIAN_POINT('Ctrl Pts',(-0.748943343284,-37.9742356128,-8.29926876182));
#65398=CARTESIAN_POINT('Ctrl Pts',(-0.748943241627,-38.0684834236,-8.29926864484));
#65399=CARTESIAN_POINT('Ctrl Pts',(-0.712958599203,-38.1627312344,-8.31224349504));
#65400=CARTESIAN_POINT('Ctrl Pts',(-0.640531165206,-38.2372246698,-8.33835860351));
#65401=CARTESIAN_POINT('Ctrl Pts',(-0.548897295487,-38.2742356618,-8.37139905011));
#65402=CARTESIAN_POINT('Ctrl Pts',(-0.457263484888,-38.2742356128,-8.40443954395));
#65403=CARTESIAN_POINT('Ctrl Pts',(-0.712043400129,-37.9742356128,-8.10864879918));
#65404=CARTESIAN_POINT('Ctrl Pts',(-0.712043400168,-38.0684833681,-8.10864879958));
#65405=CARTESIAN_POINT('Ctrl Pts',(-0.674879713076,-38.1627311233,-8.11345818589));
#65406=CARTESIAN_POINT('Ctrl Pts',(-0.600078971346,-38.2372245389,-8.12313820437));
#65407=CARTESIAN_POINT('Ctrl Pts',(-0.505442382683,-38.2742355746,-8.13538519743));
#65408=CARTESIAN_POINT('Ctrl Pts',(-0.410805778999,-38.2742356128,-8.14763218938));
#65409=CARTESIAN_POINT('Ctrl Pts',(-0.717751010187,-37.9742356128,-7.90915770911));
#65410=CARTESIAN_POINT('Ctrl Pts',(-0.717751010183,-38.0684833977,-7.90915770865));
#65411=CARTESIAN_POINT('Ctrl Pts',(-0.680755121224,-38.1627311826,-7.90809921391));
#65412=CARTESIAN_POINT('Ctrl Pts',(-0.606292144623,-38.2372246088,-7.90596874344));
#65413=CARTESIAN_POINT('Ctrl Pts',(-0.512082889029,-38.2742356211,-7.90327330976));
#65414=CARTESIAN_POINT('Ctrl Pts',(-0.417873636697,-38.2742356128,-7.90057787635));
#65415=CARTESIAN_POINT('Ctrl Pts',(-0.717273426056,-37.9742356128,-7.9495168227));
#65416=CARTESIAN_POINT('Ctrl Pts',(-0.719470863523,-37.9742356128,-8.33628951564));
#65417=CARTESIAN_POINT('Ctrl Pts',(-0.890959353803,-37.9742356128,-8.72278991704));
#65418=CARTESIAN_POINT('Ctrl Pts',(-1.23586688919,-37.9742356128,-9.00518418336));
#65419=CARTESIAN_POINT('Ctrl Pts',(-1.64860914359,-37.9742356128,-9.09702477361));
#65420=CARTESIAN_POINT('Ctrl Pts',(-2.02820898725,-37.9742356128,-9.02284995699));
#65421=CARTESIAN_POINT('Ctrl Pts',(-0.717273426056,-37.9742356128,-7.9495168227));
#65422=CARTESIAN_POINT('Ctrl Pts',(-0.717273426056,-36.2942356128,-7.9495168227));
#65423=CARTESIAN_POINT('Ctrl Pts',(-0.719470863523,-37.9742356128,-8.33628951564));
#65424=CARTESIAN_POINT('Ctrl Pts',(-0.719470863523,-36.2942356128,-8.33628951564));
#65425=CARTESIAN_POINT('Ctrl Pts',(-0.890959353803,-37.9742356128,-8.72278991704));
#65426=CARTESIAN_POINT('Ctrl Pts',(-0.890959353803,-36.2942356128,-8.72278991704));
#65427=CARTESIAN_POINT('Ctrl Pts',(-1.23586688919,-37.9742356128,-9.00518418336));
#65428=CARTESIAN_POINT('Ctrl Pts',(-1.23586688919,-36.2942356128,-9.00518418336));
#65429=CARTESIAN_POINT('Ctrl Pts',(-1.64860914359,-37.9742356128,-9.09702477361));
#65430=CARTESIAN_POINT('Ctrl Pts',(-1.64860914359,-36.2942356128,-9.09702477361));
#65431=CARTESIAN_POINT('Ctrl Pts',(-2.02820898725,-37.9742356128,-9.02284995699));
#65432=CARTESIAN_POINT('Ctrl Pts',(-2.02820898725,-36.2942356128,-9.02284995699));
#65433=CARTESIAN_POINT('Ctrl Pts',(-4.67800175618,-36.2742356128,1.76632657396));
#65434=CARTESIAN_POINT('Ctrl Pts',(-4.58800309105,-36.2742356128,1.79430664252));
#65435=CARTESIAN_POINT('Ctrl Pts',(-4.49800442593,-36.3112466293,1.82228671108));
#65436=CARTESIAN_POINT('Ctrl Pts',(-4.4268695008,-36.3857400536,1.84440215111));
#65437=CARTESIAN_POINT('Ctrl Pts',(-4.39152710765,-36.4799878332,1.85538989834));
#65438=CARTESIAN_POINT('Ctrl Pts',(-4.39152710765,-36.5742356128,1.85538989834));
#65439=CARTESIAN_POINT('Ctrl Pts',(-4.79388308266,-36.2742356128,2.13906206864));
#65440=CARTESIAN_POINT('Ctrl Pts',(-4.70258956167,-36.2742356128,2.16287719746));
#65441=CARTESIAN_POINT('Ctrl Pts',(-4.61129604067,-36.3112466293,2.18669232628));
#65442=CARTESIAN_POINT('Ctrl Pts',(-4.53913766232,-36.3857400536,2.20551579977));
#65443=CARTESIAN_POINT('Ctrl Pts',(-4.5032867799,-36.4799878332,2.21486797807));
#65444=CARTESIAN_POINT('Ctrl Pts',(-4.5032867799,-36.5742356128,2.21486797807));
#65445=CARTESIAN_POINT('Ctrl Pts',(-4.874573183,-36.2742356128,2.47604452564));
#65446=CARTESIAN_POINT('Ctrl Pts',(-4.78398140424,-36.2742356128,2.50204305306));
#65447=CARTESIAN_POINT('Ctrl Pts',(-4.69338962548,-36.3112466293,2.52804158049));
#65448=CARTESIAN_POINT('Ctrl Pts',(-4.62178590273,-36.3857400536,2.54859080965));
#65449=CARTESIAN_POINT('Ctrl Pts',(-4.58621059513,-36.4799878332,2.55880040869));
#65450=CARTESIAN_POINT('Ctrl Pts',(-4.58621059513,-36.5742356128,2.55880040869));
#65451=CARTESIAN_POINT('Ctrl Pts',(-4.98880289939,-36.2742356128,2.81842348726));
#65452=CARTESIAN_POINT('Ctrl Pts',(-4.89986264517,-36.2742356128,2.84961910006));
#65453=CARTESIAN_POINT('Ctrl Pts',(-4.81092239094,-36.3112466293,2.88081471287));
#65454=CARTESIAN_POINT('Ctrl Pts',(-4.74062403475,-36.3857400536,2.90547169884));
#65455=CARTESIAN_POINT('Ctrl Pts',(-4.70569727739,-36.4799878332,2.91772220687));
#65456=CARTESIAN_POINT('Ctrl Pts',(-4.70569727739,-36.5742356128,2.91772220687));
#65457=CARTESIAN_POINT('Ctrl Pts',(-5.24786437575,-36.2742356128,3.5327503947));
#65458=CARTESIAN_POINT('Ctrl Pts',(-5.15891348452,-36.2742356128,3.56414221201));
#65459=CARTESIAN_POINT('Ctrl Pts',(-5.06996259329,-36.3112466293,3.59553402932));
#65460=CARTESIAN_POINT('Ctrl Pts',(-4.99965582749,-36.3857400536,3.62034613592));
#65461=CARTESIAN_POINT('Ctrl Pts',(-4.96472489511,-36.4799878332,3.63267365265));
#65462=CARTESIAN_POINT('Ctrl Pts',(-4.96472489511,-36.5742356128,3.63267365265));
#65463=CARTESIAN_POINT('Ctrl Pts',(-5.46683572271,-36.2742356128,4.323032583));
#65464=CARTESIAN_POINT('Ctrl Pts',(-5.37431098316,-36.2742356128,4.342975072));
#65465=CARTESIAN_POINT('Ctrl Pts',(-5.2817862436,-36.3112466293,4.362917561));
#65466=CARTESIAN_POINT('Ctrl Pts',(-5.20865471042,-36.3857400536,4.37868007713));
#65467=CARTESIAN_POINT('Ctrl Pts',(-5.17232032954,-36.4799878332,4.38651149704));
#65468=CARTESIAN_POINT('Ctrl Pts',(-5.17232032954,-36.5742356128,4.38651149704));
#65469=CARTESIAN_POINT('Ctrl Pts',(-5.54455876033,-36.2742356128,4.75670536352));
#65470=CARTESIAN_POINT('Ctrl Pts',(-5.45006559684,-36.2742356128,4.7675841363));
#65471=CARTESIAN_POINT('Ctrl Pts',(-5.35557243336,-36.3112466293,4.77846290907));
#65472=CARTESIAN_POINT('Ctrl Pts',(-5.28088505457,-36.3857400536,4.78706157927));
#65473=CARTESIAN_POINT('Ctrl Pts',(-5.24377767918,-36.4799878332,4.79133357276));
#65474=CARTESIAN_POINT('Ctrl Pts',(-5.24377767918,-36.5742356128,4.79133357276));
#65475=CARTESIAN_POINT('Ctrl Pts',(-5.55370519489,-36.2742356128,5.19552744206));
#65476=CARTESIAN_POINT('Ctrl Pts',(-5.45936283056,-36.2742356128,5.19676129607));
#65477=CARTESIAN_POINT('Ctrl Pts',(-5.36502046622,-36.3112466293,5.19799515009));
#65478=CARTESIAN_POINT('Ctrl Pts',(-5.2904522842,-36.3857400536,5.19897032753));
#65479=CARTESIAN_POINT('Ctrl Pts',(-5.25340412236,-36.4799878332,5.19945492138));
#65480=CARTESIAN_POINT('Ctrl Pts',(-5.25340412236,-36.5742356128,5.19945492138));
#65481=CARTESIAN_POINT('Ctrl Pts',(-5.5398869008,-36.2742356128,5.60697988192));
#65482=CARTESIAN_POINT('Ctrl Pts',(-5.44569223012,-36.2742356128,5.60381634432));
#65483=CARTESIAN_POINT('Ctrl Pts',(-5.35149755944,-36.3112466293,5.60065280673));
#65484=CARTESIAN_POINT('Ctrl Pts',(-5.27704611245,-36.3857400536,5.59815234731));
#65485=CARTESIAN_POINT('Ctrl Pts',(-5.24005595177,-36.4799878332,5.596910029));
#65486=CARTESIAN_POINT('Ctrl Pts',(-5.24005595177,-36.5742356128,5.596910029));
#65487=CARTESIAN_POINT('',(-4.39149643123322,-36.5742356128,1.8552912333684));
#65488=CARTESIAN_POINT('Ctrl Pts',(-4.39152710765,-36.5742356128,1.85538989834));
#65489=CARTESIAN_POINT('Ctrl Pts',(-4.39152710765,-36.4799879394397,1.85538989834));
#65490=CARTESIAN_POINT('Ctrl Pts',(-4.42686942112142,-36.3857402660795,
1.84440217588161));
#65491=CARTESIAN_POINT('Ctrl Pts',(-4.49800418537203,-36.3112468812157,
1.82228678586809));
#65492=CARTESIAN_POINT('Ctrl Pts',(-4.58800268525026,-36.2742357796813,
1.79430676868081));
#65493=CARTESIAN_POINT('Ctrl Pts',(-4.67790730062965,-36.2742356128005,
1.76602456790413));
#65494=CARTESIAN_POINT('',(-5.24005595428587,-36.5742356128,5.59690998217945));
#65495=CARTESIAN_POINT('Origin',(-5.5377667962234,-36.5721143211971,5.60690896671464));
#65496=CARTESIAN_POINT('Ctrl Pts',(-4.39152710765,-36.5742356128,1.85538989834));
#65497=CARTESIAN_POINT('Ctrl Pts',(-4.43790342461,-36.5742356128,2.00456060571));
#65498=CARTESIAN_POINT('Ctrl Pts',(-4.47967500954,-36.5742356128,2.15155097868));
#65499=CARTESIAN_POINT('Ctrl Pts',(-4.51875357762,-36.5742356128,2.29074629422));
#65500=CARTESIAN_POINT('Ctrl Pts',(-4.62316453233,-36.5742356128,2.64995398242));
#65501=CARTESIAN_POINT('Ctrl Pts',(-4.7368681034,-36.5742356128,3.00222967269));
#65502=CARTESIAN_POINT('Ctrl Pts',(-4.81153097626,-36.5742356128,3.21707824382));
#65503=CARTESIAN_POINT('Ctrl Pts',(-5.00839926013,-36.5742356128,3.79030695886));
#65504=CARTESIAN_POINT('Ctrl Pts',(-5.17504642388,-36.5742356128,4.39981761668));
#65505=CARTESIAN_POINT('Ctrl Pts',(-5.24470483276,-36.5742356128,4.80219931419));
#65506=CARTESIAN_POINT('Ctrl Pts',(-5.25311376105,-36.5742356128,5.20808711269));
#65507=CARTESIAN_POINT('Ctrl Pts',(-5.2400559546,-36.5742356128,5.59690998219));
#65508=CARTESIAN_POINT('Ctrl Pts',(-5.24005597119,-37.9742356128,5.59690969873));
#65509=CARTESIAN_POINT('Ctrl Pts',(-5.24005597123,-38.0684833924,5.59690969762));
#65510=CARTESIAN_POINT('Ctrl Pts',(-5.27704612802,-38.162731172,5.59815213305));
#65511=CARTESIAN_POINT('Ctrl Pts',(-5.35149756715,-38.2372245963,5.60065282954));
#65512=CARTESIAN_POINT('Ctrl Pts',(-5.44569222786,-38.2742356128,5.60381666774));
#65513=CARTESIAN_POINT('Ctrl Pts',(-5.53988688857,-38.2742356128,5.60698050638));
#65514=CARTESIAN_POINT('Ctrl Pts',(-5.25247857027,-37.9742356128,5.22700723411));
#65515=CARTESIAN_POINT('Ctrl Pts',(-5.25247856712,-38.0684833932,5.22700731824));
#65516=CARTESIAN_POINT('Ctrl Pts',(-5.28952290833,-38.1627311736,5.22663645984));
#65517=CARTESIAN_POINT('Ctrl Pts',(-5.36408340703,-38.2372245982,5.22589001703));
#65518=CARTESIAN_POINT('Ctrl Pts',(-5.458416051,-38.2742356141,5.22494553728));
#65519=CARTESIAN_POINT('Ctrl Pts',(-5.55274869571,-38.2742356128,5.22400102455));
#65520=CARTESIAN_POINT('Ctrl Pts',(-5.24502230691,-37.9742356128,4.84784070798));
#65521=CARTESIAN_POINT('Ctrl Pts',(-5.24502231123,-38.0684833706,4.84784059887));
#65522=CARTESIAN_POINT('Ctrl Pts',(-5.28211738334,-38.1627311283,4.84408996285));
#65523=CARTESIAN_POINT('Ctrl Pts',(-5.35677998902,-38.2372245448,4.83654090413));
#65524=CARTESIAN_POINT('Ctrl Pts',(-5.45124181784,-38.2742355785,4.82699009502));
#65525=CARTESIAN_POINT('Ctrl Pts',(-5.54570365822,-38.2742356128,4.81743932663));
#65526=CARTESIAN_POINT('Ctrl Pts',(-5.18672938264,-37.9742356128,4.4719460563));
#65527=CARTESIAN_POINT('Ctrl Pts',(-5.1867294224,-38.0684834176,4.47194621772));
#65528=CARTESIAN_POINT('Ctrl Pts',(-5.22320733103,-38.1627312223,4.46483612118));
#65529=CARTESIAN_POINT('Ctrl Pts',(-5.29662769908,-38.2372246556,4.45052520587));
#65530=CARTESIAN_POINT('Ctrl Pts',(-5.3895178338,-38.2742356523,4.43241917655));
#65531=CARTESIAN_POINT('Ctrl Pts',(-5.4824079379,-38.2742356128,4.41431308756));
#65532=CARTESIAN_POINT('Ctrl Pts',(-4.99350448344,-37.9742356128,3.70895298504));
#65533=CARTESIAN_POINT('Ctrl Pts',(-4.99350444008,-38.068483365,3.70895280905));
#65534=CARTESIAN_POINT('Ctrl Pts',(-5.02859209909,-38.1627311172,3.69695602726));
#65535=CARTESIAN_POINT('Ctrl Pts',(-5.09921436755,-38.2372245317,3.67280984657));
#65536=CARTESIAN_POINT('Ctrl Pts',(-5.18856446387,-38.2742355698,3.64226063907));
#65537=CARTESIAN_POINT('Ctrl Pts',(-5.27791459357,-38.2742356128,3.61171149664));
#65538=CARTESIAN_POINT('Ctrl Pts',(-4.73234118526,-37.9742356128,2.99459752937));
#65539=CARTESIAN_POINT('Ctrl Pts',(-4.73234123253,-38.0684834223,2.99459772126));
#65540=CARTESIAN_POINT('Ctrl Pts',(-4.76713902192,-38.1627312318,2.98201159698));
#65541=CARTESIAN_POINT('Ctrl Pts',(-4.83717774109,-38.2372246668,2.95667884794));
#65542=CARTESIAN_POINT('Ctrl Pts',(-4.92578946733,-38.2742356598,2.92462816718));
#65543=CARTESIAN_POINT('Ctrl Pts',(-5.01440115718,-38.2742356128,2.89257741547));
#65544=CARTESIAN_POINT('Ctrl Pts',(-4.59818751884,-37.9742356128,2.61020157177));
#65545=CARTESIAN_POINT('Ctrl Pts',(-4.59818738771,-38.0684833728,2.61020114916));
#65546=CARTESIAN_POINT('Ctrl Pts',(-4.63371504264,-38.1627311328,2.5997905378));
#65547=CARTESIAN_POINT('Ctrl Pts',(-4.70522301975,-38.2372245501,2.57883726165));
#65548=CARTESIAN_POINT('Ctrl Pts',(-4.79569374678,-38.274235582,2.55232778505));
#65549=CARTESIAN_POINT('Ctrl Pts',(-4.88616453703,-38.2742356128,2.52581847142));
#65550=CARTESIAN_POINT('Ctrl Pts',(-4.51145651853,-37.9742356128,2.24114616857));
#65551=CARTESIAN_POINT('Ctrl Pts',(-4.51145651853,-38.0684833924,2.24114616857));
#65552=CARTESIAN_POINT('Ctrl Pts',(-4.54734457339,-38.1627311721,2.23191355632));
#65553=CARTESIAN_POINT('Ctrl Pts',(-4.61957776562,-38.2372245963,2.21333072384));
#65554=CARTESIAN_POINT('Ctrl Pts',(-4.71096594196,-38.2742356128,2.18982005656));
#65555=CARTESIAN_POINT('Ctrl Pts',(-4.80235411815,-38.2742356128,2.16630938881));
#65556=CARTESIAN_POINT('Ctrl Pts',(-4.39152710765,-37.9742356128,1.85538989834));
#65557=CARTESIAN_POINT('Ctrl Pts',(-4.39152710765,-38.0684833924,1.85538989834));
#65558=CARTESIAN_POINT('Ctrl Pts',(-4.4268695008,-38.1627311721,1.84440215111));
#65559=CARTESIAN_POINT('Ctrl Pts',(-4.49800442593,-38.2372245963,1.82228671108));
#65560=CARTESIAN_POINT('Ctrl Pts',(-4.58800309105,-38.2742356128,1.79430664252));
#65561=CARTESIAN_POINT('Ctrl Pts',(-4.67800175618,-38.2742356128,1.76632657396));
#65562=CARTESIAN_POINT('',(-4.39147468411897,-37.9742356128,1.85522128783252));
#65563=CARTESIAN_POINT('Ctrl Pts',(-4.67790746367798,-38.2742356127995,
1.76602510278827));
#65564=CARTESIAN_POINT('Ctrl Pts',(-4.58800268668313,-38.274235446508,1.79430676823534));
#65565=CARTESIAN_POINT('Ctrl Pts',(-4.49800418622144,-38.2372243452739,
1.82228678560402));
#65566=CARTESIAN_POINT('Ctrl Pts',(-4.42686942140277,-38.1627309603708,
1.84440217579414));
#65567=CARTESIAN_POINT('Ctrl Pts',(-4.39152710765,-38.0684832865354,1.85538989834));
#65568=CARTESIAN_POINT('Ctrl Pts',(-4.39152710765,-37.9742356128,1.85538989834));
#65569=CARTESIAN_POINT('',(-5.2400559546,-37.9742356128,5.59690998219));
#65570=CARTESIAN_POINT('Ctrl Pts',(-4.39152710765,-37.9742356128,1.85538989834));
#65571=CARTESIAN_POINT('Ctrl Pts',(-4.43790342461,-37.9742356128,2.00456060571));
#65572=CARTESIAN_POINT('Ctrl Pts',(-4.47967500954,-37.9742356128,2.15155097868));
#65573=CARTESIAN_POINT('Ctrl Pts',(-4.51875357762,-37.9742356128,2.29074629422));
#65574=CARTESIAN_POINT('Ctrl Pts',(-4.62316453233,-37.9742356128,2.64995398242));
#65575=CARTESIAN_POINT('Ctrl Pts',(-4.7368681034,-37.9742356128,3.00222967269));
#65576=CARTESIAN_POINT('Ctrl Pts',(-4.81153097626,-37.9742356128,3.21707824382));
#65577=CARTESIAN_POINT('Ctrl Pts',(-5.00839926013,-37.9742356128,3.79030695886));
#65578=CARTESIAN_POINT('Ctrl Pts',(-5.17504642388,-37.9742356128,4.39981761668));
#65579=CARTESIAN_POINT('Ctrl Pts',(-5.24470483276,-37.9742356128,4.80219931419));
#65580=CARTESIAN_POINT('Ctrl Pts',(-5.25311376105,-37.9742356128,5.20808711269));
#65581=CARTESIAN_POINT('Ctrl Pts',(-5.2400559546,-37.9742356128,5.59690998219));
#65582=CARTESIAN_POINT('Origin',(-5.5377667758297,-37.9763568898754,5.60691012513041));
#65583=CARTESIAN_POINT('Ctrl Pts',(-4.39143626758763,-37.9742356128,1.8550977087646));
#65584=CARTESIAN_POINT('Ctrl Pts',(-4.39143626758763,-36.2942356128,1.8550977087646));
#65585=CARTESIAN_POINT('Ctrl Pts',(-4.3914544356001,-37.9742356128,1.85515614667968));
#65586=CARTESIAN_POINT('Ctrl Pts',(-4.3914544356001,-36.2942356128,1.85515614667968));
#65587=CARTESIAN_POINT('Ctrl Pts',(-4.39147260361258,-37.9742356128,1.85521458459476));
#65588=CARTESIAN_POINT('Ctrl Pts',(-4.39147260361258,-36.2942356128,1.85521458459476));
#65589=CARTESIAN_POINT('Ctrl Pts',(-4.39149077162505,-37.9742356128,1.85527302250984));
#65590=CARTESIAN_POINT('Ctrl Pts',(-4.39149077162505,-36.2942356128,1.85527302250984));
#65591=CARTESIAN_POINT('Ctrl Pts',(-4.39150893963753,-37.9742356128,1.85533146042492));
#65592=CARTESIAN_POINT('Ctrl Pts',(-4.39150893963753,-36.2942356128,1.85533146042492));
#65593=CARTESIAN_POINT('Ctrl Pts',(-4.39152710765,-37.9742356128,1.85538989834));
#65594=CARTESIAN_POINT('Ctrl Pts',(-4.39152710765,-36.2942356128,1.85538989834));
#65595=CARTESIAN_POINT('Ctrl Pts',(-4.43790342461,-37.9742356128,2.00456060571));
#65596=CARTESIAN_POINT('Ctrl Pts',(-4.43790342461,-36.2942356128,2.00456060571));
#65597=CARTESIAN_POINT('Ctrl Pts',(-4.47967500954,-37.9742356128,2.15155097868));
#65598=CARTESIAN_POINT('Ctrl Pts',(-4.47967500954,-36.2942356128,2.15155097868));
#65599=CARTESIAN_POINT('Ctrl Pts',(-4.51875357762,-37.9742356128,2.29074629422));
#65600=CARTESIAN_POINT('Ctrl Pts',(-4.51875357762,-36.2942356128,2.29074629422));
#65601=CARTESIAN_POINT('Ctrl Pts',(-4.62316453233,-37.9742356128,2.64995398242));
#65602=CARTESIAN_POINT('Ctrl Pts',(-4.62316453233,-36.2942356128,2.64995398242));
#65603=CARTESIAN_POINT('Ctrl Pts',(-4.7368681034,-37.9742356128,3.00222967269));
#65604=CARTESIAN_POINT('Ctrl Pts',(-4.7368681034,-36.2942356128,3.00222967269));
#65605=CARTESIAN_POINT('Ctrl Pts',(-4.81153097626,-37.9742356128,3.21707824382));
#65606=CARTESIAN_POINT('Ctrl Pts',(-4.81153097626,-36.2942356128,3.21707824382));
#65607=CARTESIAN_POINT('Ctrl Pts',(-5.00839926013,-37.9742356128,3.79030695886));
#65608=CARTESIAN_POINT('Ctrl Pts',(-5.00839926013,-36.2942356128,3.79030695886));
#65609=CARTESIAN_POINT('Ctrl Pts',(-5.17504642388,-37.9742356128,4.39981761668));
#65610=CARTESIAN_POINT('Ctrl Pts',(-5.17504642388,-36.2942356128,4.39981761668));
#65611=CARTESIAN_POINT('Ctrl Pts',(-5.24470483276,-37.9742356128,4.80219931419));
#65612=CARTESIAN_POINT('Ctrl Pts',(-5.24470483276,-36.2942356128,4.80219931419));
#65613=CARTESIAN_POINT('Ctrl Pts',(-5.25311376105,-37.9742356128,5.20808711269));
#65614=CARTESIAN_POINT('Ctrl Pts',(-5.25311376105,-36.2942356128,5.20808711269));
#65615=CARTESIAN_POINT('Ctrl Pts',(-5.2400559546,-37.9742356128,5.59690998219));
#65616=CARTESIAN_POINT('Ctrl Pts',(-5.2400559546,-36.2942356128,5.59690998219));
#65617=CARTESIAN_POINT('',(-4.39143626207,-37.2742356128,1.85509771048));
#65618=CARTESIAN_POINT('',(-5.2400559546,-37.2742356128,5.59690998219));
#65619=CARTESIAN_POINT('Ctrl Pts',(-5.53988692571,-36.2742356128,5.60697918103));
#65620=CARTESIAN_POINT('Ctrl Pts',(-5.4456922481,-36.2742356128,5.60381584892));
#65621=CARTESIAN_POINT('Ctrl Pts',(-5.35149757048,-36.3112466293,5.60065251681));
#65622=CARTESIAN_POINT('Ctrl Pts',(-5.277046118,-36.3857400536,5.59815221981));
#65623=CARTESIAN_POINT('Ctrl Pts',(-5.2400559546,-36.4799878332,5.59690998219));
#65624=CARTESIAN_POINT('Ctrl Pts',(-5.2400559546,-36.5742356128,5.59690998219));
#65625=CARTESIAN_POINT('Ctrl Pts',(-5.51566436809,-36.2742356128,6.32825533085));
#65626=CARTESIAN_POINT('Ctrl Pts',(-5.42188047368,-36.2742356128,6.31286008937));
#65627=CARTESIAN_POINT('Ctrl Pts',(-5.32809657928,-36.3112466293,6.29746484788));
#65628=CARTESIAN_POINT('Ctrl Pts',(-5.25396980975,-36.3857400536,6.28529645234));
#65629=CARTESIAN_POINT('Ctrl Pts',(-5.21714096054,-36.4799878332,6.27925075521));
#65630=CARTESIAN_POINT('Ctrl Pts',(-5.21714096054,-36.5742356128,6.27925075521));
#65631=CARTESIAN_POINT('Ctrl Pts',(-5.37435587484,-36.2742356128,7.04580159469));
#65632=CARTESIAN_POINT('Ctrl Pts',(-5.28297016404,-36.2742356128,7.01818508491));
#65633=CARTESIAN_POINT('Ctrl Pts',(-5.19158445325,-36.3112466293,6.99056857513));
#65634=CARTESIAN_POINT('Ctrl Pts',(-5.11935320751,-36.3857400536,6.96874049199));
#65635=CARTESIAN_POINT('Ctrl Pts',(-5.08346612282,-36.4799878332,6.95789551384));
#65636=CARTESIAN_POINT('Ctrl Pts',(-5.08346612282,-36.5742356128,6.95789551384));
#65637=CARTESIAN_POINT('Ctrl Pts',(-5.11602160615,-36.2742356128,7.73361379617));
#65638=CARTESIAN_POINT('Ctrl Pts',(-5.02905151582,-36.2742356128,7.69427724615));
#65639=CARTESIAN_POINT('Ctrl Pts',(-4.94208142549,-36.3112466293,7.65494069614));
#65640=CARTESIAN_POINT('Ctrl Pts',(-4.87334027673,-36.3857400536,7.6238490956));
#65641=CARTESIAN_POINT('Ctrl Pts',(-4.83918721061,-36.4799878332,7.60840166858));
#65642=CARTESIAN_POINT('Ctrl Pts',(-4.83918721061,-36.5742356128,7.60840166858));
#65643=CARTESIAN_POINT('Ctrl Pts',(-4.25296434,-36.2742356128,9.22903839862));
#65644=CARTESIAN_POINT('Ctrl Pts',(-4.1806520628,-36.2742356128,9.16427735215));
#65645=CARTESIAN_POINT('Ctrl Pts',(-4.10833978559,-36.3112466293,9.09951630568));
#65646=CARTESIAN_POINT('Ctrl Pts',(-4.05118418906,-36.3857400536,9.04832918894));
#65647=CARTESIAN_POINT('Ctrl Pts',(-4.02278721273,-36.4799878332,9.02289758531));
#65648=CARTESIAN_POINT('Ctrl Pts',(-4.02278721273,-36.5742356128,9.02289758531));
#65649=CARTESIAN_POINT('Ctrl Pts',(-2.88301385607,-36.2742356128,10.310599153));
#65650=CARTESIAN_POINT('Ctrl Pts',(-2.83398118867,-36.2742356128,10.2274899849));
#65651=CARTESIAN_POINT('Ctrl Pts',(-2.78494852128,-36.3112466293,10.1443808169));
#65652=CARTESIAN_POINT('Ctrl Pts',(-2.74619309625,-36.3857400536,10.0786913484));
#65653=CARTESIAN_POINT('Ctrl Pts',(-2.7269380283,-36.4799878332,10.0460544548));
#65654=CARTESIAN_POINT('Ctrl Pts',(-2.7269380283,-36.5742356128,10.0460544548));
#65655=CARTESIAN_POINT('Ctrl Pts',(-1.96549293319,-36.2742356128,10.7471218767));
#65656=CARTESIAN_POINT('Ctrl Pts',(-1.93197492963,-36.2742356128,10.6565618655));
#65657=CARTESIAN_POINT('Ctrl Pts',(-1.89845692606,-36.3112466293,10.5660018543));
#65658=CARTESIAN_POINT('Ctrl Pts',(-1.87196436596,-36.3857400536,10.4944232419));
#65659=CARTESIAN_POINT('Ctrl Pts',(-1.85880181419,-36.4799878332,10.4588604081));
#65660=CARTESIAN_POINT('Ctrl Pts',(-1.85880181419,-36.5742356128,10.4588604081));
#65661=CARTESIAN_POINT('Ctrl Pts',(-0.9824065633,-36.2742356128,10.9642669745));
#65662=CARTESIAN_POINT('Ctrl Pts',(-0.965785252294,-36.2742356128,10.8700205667));
#65663=CARTESIAN_POINT('Ctrl Pts',(-0.949163941288,-36.3112466293,10.7757741588));
#65664=CARTESIAN_POINT('Ctrl Pts',(-0.936026419048,-36.3857400536,10.7012818184));
#65665=CARTESIAN_POINT('Ctrl Pts',(-0.929499287155,-36.4799878332,10.664271341));
#65666=CARTESIAN_POINT('Ctrl Pts',(-0.929499287155,-36.5742356128,10.664271341));
#65667=CARTESIAN_POINT('Ctrl Pts',(-2.46701990947E-5,-36.2742356128,10.9643459861));
#65668=CARTESIAN_POINT('Ctrl Pts',(-1.69198316304E-5,-36.2742356128,10.8700982068));
#65669=CARTESIAN_POINT('Ctrl Pts',(-9.16946416574E-6,-36.3112466293,10.7758504274));
#65670=CARTESIAN_POINT('Ctrl Pts',(-3.04357542591E-6,-36.3857400536,10.7013570034));
#65671=CARTESIAN_POINT('Ctrl Pts',(-1.32396316133E-11,-36.4799878332,10.664345987));
#65672=CARTESIAN_POINT('Ctrl Pts',(-1.32396316133E-11,-36.5742356128,10.664345987));
#65673=CARTESIAN_POINT('',(3.21923099319093E-10,-36.5742356128,10.66434598565));
#65674=CARTESIAN_POINT('Origin',(-5.43957144643002E-5,-36.5721143038111,
10.9622246741472));
#65675=CARTESIAN_POINT('Ctrl Pts',(-5.2400559546,-36.5742356128,5.59690998219));
#65676=CARTESIAN_POINT('Ctrl Pts',(-5.18595136098,-36.5742356128,7.20798481558));
#65677=CARTESIAN_POINT('Ctrl Pts',(-4.51434339457,-36.5742356128,8.79964985146));
#65678=CARTESIAN_POINT('Ctrl Pts',(-3.22524412625,-36.5742356128,10.0462831132));
#65679=CARTESIAN_POINT('Ctrl Pts',(-1.61198306736,-36.5742356128,10.6642180635));
#65680=CARTESIAN_POINT('Ctrl Pts',(-8.881784197E-16,-36.5742356128,10.664345987));
#65681=CARTESIAN_POINT('Ctrl Pts',(2.47493525452E-10,-37.9742356128,10.6643459881));
#65682=CARTESIAN_POINT('Ctrl Pts',(2.51954845654E-10,-38.0684833924,10.6643459881));
#65683=CARTESIAN_POINT('Ctrl Pts',(-2.95195493277E-6,-38.1627311721,10.7013570045));
#65684=CARTESIAN_POINT('Ctrl Pts',(-8.89397497965E-6,-38.2372245963,10.7758504286));
#65685=CARTESIAN_POINT('Ctrl Pts',(-1.64117176949E-5,-38.2742356128,10.8700982079));
#65686=CARTESIAN_POINT('Ctrl Pts',(-2.39294621618E-5,-38.2742356128,10.9643459873));
#65687=CARTESIAN_POINT('Ctrl Pts',(-0.781410362137,-37.9742356128,10.6642834957));
#65688=CARTESIAN_POINT('Ctrl Pts',(-0.781410363148,-38.068483393,10.6642834957));
#65689=CARTESIAN_POINT('Ctrl Pts',(-0.786907976509,-38.1627311731,10.7012940655));
#65690=CARTESIAN_POINT('Ctrl Pts',(-0.797973495794,-38.2372245975,10.7757865915));
#65691=CARTESIAN_POINT('Ctrl Pts',(-0.811973282143,-38.2742356136,10.8700332341));
#65692=CARTESIAN_POINT('Ctrl Pts',(-0.8259730681,-38.2742356128,10.9642798764));
#65693=CARTESIAN_POINT('Ctrl Pts',(-1.56278771434,-37.9742356128,10.5190720913));
#65694=CARTESIAN_POINT('Ctrl Pts',(-1.56278775086,-38.0684833913,10.5190720271));
#65695=CARTESIAN_POINT('Ctrl Pts',(-1.57383244467,-38.1627311698,10.5550601671));
#65696=CARTESIAN_POINT('Ctrl Pts',(-1.59606204838,-38.2372245937,10.6274948874));
#65697=CARTESIAN_POINT('Ctrl Pts',(-1.6241867049,-38.2742356111,10.7191380707));
#65698=CARTESIAN_POINT('Ctrl Pts',(-1.65231134708,-38.2742356128,10.8107812798));
#65699=CARTESIAN_POINT('Ctrl Pts',(-2.30773304724,-37.9742356128,10.2275491754));
#65700=CARTESIAN_POINT('Ctrl Pts',(-2.3077327816,-38.0684833927,10.2275493948));
#65701=CARTESIAN_POINT('Ctrl Pts',(-2.32403298045,-38.1627311726,10.2614708417));
#65702=CARTESIAN_POINT('Ctrl Pts',(-2.3568414097,-38.237224597,10.3297456012));
#65703=CARTESIAN_POINT('Ctrl Pts',(-2.39835018111,-38.2742356133,10.4161254622));
#65704=CARTESIAN_POINT('Ctrl Pts',(-2.43985905679,-38.2742356128,10.5025052368));
#65705=CARTESIAN_POINT('Ctrl Pts',(-3.69592891366,-37.9742356128,9.354903989));
#65706=CARTESIAN_POINT('Ctrl Pts',(-3.69592919608,-38.0684833921,9.35490375571));
#65707=CARTESIAN_POINT('Ctrl Pts',(-3.72202345283,-38.1627311714,9.38267044843));
#65708=CARTESIAN_POINT('Ctrl Pts',(-3.77454386522,-38.2372245956,9.43855767121));
#65709=CARTESIAN_POINT('Ctrl Pts',(-3.84099164681,-38.2742356124,9.50926539283));
#65710=CARTESIAN_POINT('Ctrl Pts',(-3.90743931755,-38.2742356128,9.57997320631));
#65711=CARTESIAN_POINT('Ctrl Pts',(-4.66459380705,-37.9742356128,8.0273898467));
#65712=CARTESIAN_POINT('Ctrl Pts',(-4.66459350678,-38.0684833928,8.02739009474));
#65713=CARTESIAN_POINT('Ctrl Pts',(-4.69751121102,-38.1627311727,8.04579864842));
#65714=CARTESIAN_POINT('Ctrl Pts',(-4.76376635599,-38.2372245971,8.08285001799));
#65715=CARTESIAN_POINT('Ctrl Pts',(-4.84759134344,-38.2742356134,8.12972656905));
#65716=CARTESIAN_POINT('Ctrl Pts',(-4.93141644876,-38.2742356128,8.17660302246));
#65717=CARTESIAN_POINT('Ctrl Pts',(-5.02028636901,-37.9742356128,7.25209197216));
#65718=CARTESIAN_POINT('Ctrl Pts',(-5.02028638981,-38.0684833959,7.25209217123));
#65719=CARTESIAN_POINT('Ctrl Pts',(-5.05572819588,-38.162731179,7.26502088603));
#65720=CARTESIAN_POINT('Ctrl Pts',(-5.12706320165,-38.2372246045,7.29104232124));
#65721=CARTESIAN_POINT('Ctrl Pts',(-5.21731498541,-38.2742356183,7.32396424097));
#65722=CARTESIAN_POINT('Ctrl Pts',(-5.30756675884,-38.2742356128,7.35688608211));
#65723=CARTESIAN_POINT('Ctrl Pts',(-5.21217205227,-37.9742356128,6.4272101526));
#65724=CARTESIAN_POINT('Ctrl Pts',(-5.21217205227,-38.0684833924,6.4272101526));
#65725=CARTESIAN_POINT('Ctrl Pts',(-5.24896592505,-38.1627311721,6.43429734393));
#65726=CARTESIAN_POINT('Ctrl Pts',(-5.32302228695,-38.2372245964,6.44856227116));
#65727=CARTESIAN_POINT('Ctrl Pts',(-5.41671710674,-38.2742356128,6.46660989106));
#65728=CARTESIAN_POINT('Ctrl Pts',(-5.51041192654,-38.2742356128,6.48465751096));
#65729=CARTESIAN_POINT('Ctrl Pts',(-5.2400559546,-37.9742356128,5.59690998219));
#65730=CARTESIAN_POINT('Ctrl Pts',(-5.2400559546,-38.0684833924,5.59690998219));
#65731=CARTESIAN_POINT('Ctrl Pts',(-5.277046118,-38.1627311721,5.59815221981));
#65732=CARTESIAN_POINT('Ctrl Pts',(-5.35149757048,-38.2372245963,5.60065251681));
#65733=CARTESIAN_POINT('Ctrl Pts',(-5.4456922481,-38.2742356128,5.60381584892));
#65734=CARTESIAN_POINT('Ctrl Pts',(-5.53988692571,-38.2742356128,5.60697918103));
#65735=CARTESIAN_POINT('',(1.72248049157275E-10,-37.9742356128,10.6643459863));
#65736=CARTESIAN_POINT('Ctrl Pts',(-5.2400559546,-37.9742356128,5.59690998219));
#65737=CARTESIAN_POINT('Ctrl Pts',(-5.18595136098,-37.9742356128,7.20798481558));
#65738=CARTESIAN_POINT('Ctrl Pts',(-4.51434339457,-37.9742356128,8.79964985146));
#65739=CARTESIAN_POINT('Ctrl Pts',(-3.22524412625,-37.9742356128,10.0462831132));
#65740=CARTESIAN_POINT('Ctrl Pts',(-1.61198306736,-37.9742356128,10.6642180635));
#65741=CARTESIAN_POINT('Ctrl Pts',(-8.881784197E-16,-37.9742356128,10.664345987));
#65742=CARTESIAN_POINT('Ctrl Pts',(-2.39294567467071E-5,-38.2742356128,
10.9643459746877));
#65743=CARTESIAN_POINT('Ctrl Pts',(1.65351811779069E-5,-38.2742356089377,
10.8700981935102));
#65744=CARTESIAN_POINT('Ctrl Pts',(8.96134118167951E-6,-38.2372245904188,
10.7758504184188));
#65745=CARTESIAN_POINT('Ctrl Pts',(2.97497562388355E-6,-38.1627311670551,
10.7013569985189));
#65746=CARTESIAN_POINT('Ctrl Pts',(7.28328000219216E-10,-38.0684833899775,
10.6643459842));
#65747=CARTESIAN_POINT('Ctrl Pts',(-8.881784197E-16,-37.9742356128,10.664345987));
#65748=CARTESIAN_POINT('Ctrl Pts',(-5.2400559546,-37.9742356128,5.59690998219));
#65749=CARTESIAN_POINT('Ctrl Pts',(-5.2400559546,-36.2942356128,5.59690998219));
#65750=CARTESIAN_POINT('Ctrl Pts',(-5.18595136098,-37.9742356128,7.20798481558));
#65751=CARTESIAN_POINT('Ctrl Pts',(-5.18595136098,-36.2942356128,7.20798481558));
#65752=CARTESIAN_POINT('Ctrl Pts',(-4.51434339457,-37.9742356128,8.79964985146));
#65753=CARTESIAN_POINT('Ctrl Pts',(-4.51434339457,-36.2942356128,8.79964985146));
#65754=CARTESIAN_POINT('Ctrl Pts',(-3.22524412625,-37.9742356128,10.0462831132));
#65755=CARTESIAN_POINT('Ctrl Pts',(-3.22524412625,-36.2942356128,10.0462831132));
#65756=CARTESIAN_POINT('Ctrl Pts',(-1.61198306736,-37.9742356128,10.6642180635));
#65757=CARTESIAN_POINT('Ctrl Pts',(-1.61198306736,-36.2942356128,10.6642180635));
#65758=CARTESIAN_POINT('Ctrl Pts',(1.22124532709E-15,-37.9742356128,10.664345987));
#65759=CARTESIAN_POINT('Ctrl Pts',(1.22124532709E-15,-36.2942356128,10.664345987));
#65760=CARTESIAN_POINT('',(-4.4408920985E-16,-37.2742356128,10.664345987));
#65761=CARTESIAN_POINT('Ctrl Pts',(2.32481332798E-5,-36.2742356128,10.9643459795));
#65762=CARTESIAN_POINT('Ctrl Pts',(1.59449213495E-5,-36.2742356128,10.8700982006));
#65763=CARTESIAN_POINT('Ctrl Pts',(8.64170941739E-6,-36.3112466293,10.7758504216));
#65764=CARTESIAN_POINT('Ctrl Pts',(2.86925231308E-6,-36.3857400536,10.7013569978));
#65765=CARTESIAN_POINT('Ctrl Pts',(1.2876946176E-9,-36.4799878332,10.6643459816));
#65766=CARTESIAN_POINT('Ctrl Pts',(1.2876946176E-9,-36.5742356128,10.6643459816));
#65767=CARTESIAN_POINT('Ctrl Pts',(0.852036142414,-36.2742356128,10.9642783046));
#65768=CARTESIAN_POINT('Ctrl Pts',(0.837609587463,-36.2742356128,10.8700316767));
#65769=CARTESIAN_POINT('Ctrl Pts',(0.823183032512,-36.3112466293,10.7757850489));
#65770=CARTESIAN_POINT('Ctrl Pts',(0.811780239059,-36.3857400536,10.7012925346));
#65771=CARTESIAN_POINT('Ctrl Pts',(0.806114991769,-36.4799878332,10.6642819707));
#65772=CARTESIAN_POINT('Ctrl Pts',(0.806114991769,-36.5742356128,10.6642819707));
#65773=CARTESIAN_POINT('Ctrl Pts',(1.70453832905,-36.2742356128,10.8009343674));
#65774=CARTESIAN_POINT('Ctrl Pts',(1.6754994877,-36.2742356128,10.7094585914));
#65775=CARTESIAN_POINT('Ctrl Pts',(1.64646064634,-36.3112466293,10.6179828154));
#65776=CARTESIAN_POINT('Ctrl Pts',(1.62350842394,-36.3857400536,10.5456803825));
#65777=CARTESIAN_POINT('Ctrl Pts',(1.61210482618,-36.4799878332,10.5097579288));
#65778=CARTESIAN_POINT('Ctrl Pts',(1.61210482618,-36.5742356128,10.5097579288));
#65779=CARTESIAN_POINT('Ctrl Pts',(2.51436099301,-36.2742356128,10.4728151835));
#65780=CARTESIAN_POINT('Ctrl Pts',(2.47159007241,-36.2742356128,10.3869496626));
#65781=CARTESIAN_POINT('Ctrl Pts',(2.42881915182,-36.3112466293,10.3010841417));
#65782=CARTESIAN_POINT('Ctrl Pts',(2.39501300852,-36.3857400536,10.2332160276));
#65783=CARTESIAN_POINT('Ctrl Pts',(2.37821692435,-36.4799878332,10.1994967416));
#65784=CARTESIAN_POINT('Ctrl Pts',(2.37821692435,-36.5742356128,10.1994967416));
#65785=CARTESIAN_POINT('Ctrl Pts',(3.9668324501,-36.2742356128,9.52325772634));
#65786=CARTESIAN_POINT('Ctrl Pts',(3.89937291488,-36.2742356128,9.45350328533));
#65787=CARTESIAN_POINT('Ctrl Pts',(3.83191337967,-36.3112466293,9.38374884432));
#65788=CARTESIAN_POINT('Ctrl Pts',(3.77859339503,-36.3857400536,9.32861497459));
#65789=CARTESIAN_POINT('Ctrl Pts',(3.75210208034,-36.4799878332,9.30122244455));
#65790=CARTESIAN_POINT('Ctrl Pts',(3.75210208034,-36.5742356128,9.30122244455));
#65791=CARTESIAN_POINT('Ctrl Pts',(4.96450063028,-36.2742356128,8.10336572511));
#65792=CARTESIAN_POINT('Ctrl Pts',(4.88011657299,-36.2742356128,8.05774290187));
#65793=CARTESIAN_POINT('Ctrl Pts',(4.7957325157,-36.3112466293,8.01212007863));
#65794=CARTESIAN_POINT('Ctrl Pts',(4.72903535812,-36.3857400536,7.97605978415));
#65795=CARTESIAN_POINT('Ctrl Pts',(4.69589783357,-36.4799878332,7.95814376839));
#65796=CARTESIAN_POINT('Ctrl Pts',(4.69589783357,-36.5742356128,7.95814376839));
#65797=CARTESIAN_POINT('Ctrl Pts',(5.31945709196,-36.2742356128,7.30507701677));
#65798=CARTESIAN_POINT('Ctrl Pts',(5.22900416127,-36.2742356128,7.27301018271));
#65799=CARTESIAN_POINT('Ctrl Pts',(5.13855123059,-36.3112466293,7.24094334865));
#65800=CARTESIAN_POINT('Ctrl Pts',(5.06705725129,-36.3857400536,7.21559783004));
#65801=CARTESIAN_POINT('Ctrl Pts',(5.03153647124,-36.4799878332,7.20300511378));
#65802=CARTESIAN_POINT('Ctrl Pts',(5.03153647124,-36.5742356128,7.20300511378));
#65803=CARTESIAN_POINT('Ctrl Pts',(5.51128814508,-36.2742356128,6.45856839125));
#65804=CARTESIAN_POINT('Ctrl Pts',(5.41757775177,-36.2742356128,6.44098444573));
#65805=CARTESIAN_POINT('Ctrl Pts',(5.32386735846,-36.3112466293,6.4234005002));
#65806=CARTESIAN_POINT('Ctrl Pts',(5.24979868601,-36.3857400536,6.40950208689));
#65807=CARTESIAN_POINT('Ctrl Pts',(5.21299869879,-36.4799878332,6.40259695426));
#65808=CARTESIAN_POINT('Ctrl Pts',(5.21299869879,-36.5742356128,6.40259695426));
#65809=CARTESIAN_POINT('Ctrl Pts',(5.53988691225,-36.2742356128,5.60697948238));
#65810=CARTESIAN_POINT('Ctrl Pts',(5.44569223796,-36.2742356128,5.60381605578));
#65811=CARTESIAN_POINT('Ctrl Pts',(5.35149756366,-36.3112466293,5.60065262919));
#65812=CARTESIAN_POINT('Ctrl Pts',(5.27704611381,-36.3857400536,5.5981522575));
#65813=CARTESIAN_POINT('Ctrl Pts',(5.24005595171,-36.4799878332,5.59690998278));
#65814=CARTESIAN_POINT('Ctrl Pts',(5.24005595171,-36.5742356128,5.59690998278));
#65815=CARTESIAN_POINT('',(5.2400559538775,-36.5742356128,5.5969099823375));
#65816=CARTESIAN_POINT('Origin',(5.53776680476872,-36.5721143148321,5.60690846915117));
#65817=CARTESIAN_POINT('Ctrl Pts',(1.28769461759875E-9,-36.5742356128,10.6643459816));
#65818=CARTESIAN_POINT('Ctrl Pts',(0.147840141500339,-36.5742356128,10.6643342421081));
#65819=CARTESIAN_POINT('Ctrl Pts',(0.295679233170314,-36.5742356128,10.6580838271699));
#65820=CARTESIAN_POINT('Ctrl Pts',(0.442988225077906,-36.5742356128,10.6456029881052));
#65821=CARTESIAN_POINT('Ctrl Pts',(0.592364761454907,-36.5742356128,10.6329469751461));
#65822=CARTESIAN_POINT('Ctrl Pts',(0.741195961727722,-36.5742356128,10.6138844583169));
#65823=CARTESIAN_POINT('Ctrl Pts',(0.888934980438098,-36.5742356128,10.5884776060529));
#65824=CARTESIAN_POINT('Ctrl Pts',(1.03778268782953,-36.5742356128,10.5628800912965));
#65825=CARTESIAN_POINT('Ctrl Pts',(1.18552149683487,-36.5742356128,10.5308427707656));
#65826=CARTESIAN_POINT('Ctrl Pts',(1.33160089085122,-36.5742356128,10.4924820059666));
#65827=CARTESIAN_POINT('Ctrl Pts',(1.47862414497429,-36.5742356128,10.4538733814623));
#65828=CARTESIAN_POINT('Ctrl Pts',(1.62396619622945,-36.5742356128,10.408859457976));
#65829=CARTESIAN_POINT('Ctrl Pts',(1.76707866522786,-36.5742356128,10.3576103681606));
#65830=CARTESIAN_POINT('Ctrl Pts',(1.91093255878637,-36.5742356128,10.3060957715438));
#65831=CARTESIAN_POINT('Ctrl Pts',(2.05253342556236,-36.5742356128,10.2482813783103));
#65832=CARTESIAN_POINT('Ctrl Pts',(2.19134149631081,-36.5742356128,10.1843898178516));
#65833=CARTESIAN_POINT('Ctrl Pts',(2.33084529538293,-36.5742356128,10.1201780226399));
#65834=CARTESIAN_POINT('Ctrl Pts',(2.46752793929734,-36.5742356128,10.0498281384951));
#65835=CARTESIAN_POINT('Ctrl Pts',(2.60086315421496,-36.5742356128,9.97361415794421));
#65836=CARTESIAN_POINT('Ctrl Pts',(2.73433276278183,-36.5742356128,9.8973233584151));
#65837=CARTESIAN_POINT('Ctrl Pts',(2.86444790857184,-36.5742356128,9.8151568205301));
#65838=CARTESIAN_POINT('Ctrl Pts',(2.99070667424014,-36.5742356128,9.72743476808259));
#65839=CARTESIAN_POINT('Ctrl Pts',(3.11682204767723,-36.5742356128,9.63981234167499));
#65840=CARTESIAN_POINT('Ctrl Pts',(3.23908952393931,-36.5742356128,9.54664721325454));
#65841=CARTESIAN_POINT('Ctrl Pts',(3.3570389094003,-36.5742356128,9.44830087319822));
#65842=CARTESIAN_POINT('Ctrl Pts',(3.456001761657,-36.5742356128,9.36578552745953));
#65843=CARTESIAN_POINT('Ctrl Pts',(3.55192525354885,-36.5742356128,9.27962356642855));
#65844=CARTESIAN_POINT('Ctrl Pts',(3.64455010326894,-36.5742356128,9.19005000033049));
#65845=CARTESIAN_POINT('Ctrl Pts',(3.75506240265809,-36.5742356128,9.08317823984834));
#65846=CARTESIAN_POINT('Ctrl Pts',(3.86087792258727,-36.5742356128,8.97144924806346));
#65847=CARTESIAN_POINT('Ctrl Pts',(3.96158460510385,-36.5742356128,8.85529518741082));
#65848=CARTESIAN_POINT('Ctrl Pts',(4.06235959274001,-36.5742356128,8.73906234432981));
#65849=CARTESIAN_POINT('Ctrl Pts',(4.15801862492861,-36.5742356128,8.61839866232239));
#65850=CARTESIAN_POINT('Ctrl Pts',(4.24818890413247,-36.5742356128,8.49377048410246));
#65851=CARTESIAN_POINT('Ctrl Pts',(4.33823238792445,-36.5742356128,8.36931755521443));
#65852=CARTESIAN_POINT('Ctrl Pts',(4.42280237436131,-36.5742356128,8.24091151652117));
#65853=CARTESIAN_POINT('Ctrl Pts',(4.50157025117896,-36.5742356128,8.10904633222281));
#65854=CARTESIAN_POINT('Ctrl Pts',(4.58012232474487,-36.5742356128,7.97754242382412));
#65855=CARTESIAN_POINT('Ctrl Pts',(4.65290388085685,-36.5742356128,7.84259854510023));
#65856=CARTESIAN_POINT('Ctrl Pts',(4.71963384069473,-36.5742356128,7.70473036952541));
#65857=CARTESIAN_POINT('Ctrl Pts',(4.78609874864947,-36.5742356128,7.56740980734118));
#65858=CARTESIAN_POINT('Ctrl Pts',(4.84655989621262,-36.5742356128,7.42718837846509));
#65859=CARTESIAN_POINT('Ctrl Pts',(4.90078630758145,-36.5742356128,7.28459753902635));
#65860=CARTESIAN_POINT('Ctrl Pts',(4.95456804763369,-36.5742356128,7.14317598323936));
#65861=CARTESIAN_POINT('Ctrl Pts',(5.00221678397136,-36.5742356128,6.99942396510125));
#65862=CARTESIAN_POINT('Ctrl Pts',(5.04355503451248,-36.5742356128,6.85387786797466));
#65863=CARTESIAN_POINT('Ctrl Pts',(5.08466686288025,-36.5742356128,6.70912897109731));
#65864=CARTESIAN_POINT('Ctrl Pts',(5.11953702859418,-36.5742356128,6.56260582424903));
#65865=CARTESIAN_POINT('Ctrl Pts',(5.14804013322182,-36.5742356128,6.41485027913283));
#65866=CARTESIAN_POINT('Ctrl Pts',(5.17626254570044,-36.5742356128,6.26854979731691));
#65867=CARTESIAN_POINT('Ctrl Pts',(5.19824261046229,-36.5742356128,6.12104129530587));
#65868=CARTESIAN_POINT('Ctrl Pts',(5.21390829155022,-36.5742356128,5.9728613808213));
#65869=CARTESIAN_POINT('Ctrl Pts',(5.22711794574893,-36.5742356128,5.84791274829469));
#65870=CARTESIAN_POINT('Ctrl Pts',(5.23583872043894,-36.5742356128,5.7224869695072));
#65871=CARTESIAN_POINT('Ctrl Pts',(5.24005595171,-36.5742356128,5.59690998278));
#65872=CARTESIAN_POINT('Ctrl Pts',(5.24005594912,-37.9742356128,5.5969099833));
#65873=CARTESIAN_POINT('Ctrl Pts',(5.24005594912,-38.0684833924,5.59690998329));
#65874=CARTESIAN_POINT('Ctrl Pts',(5.27704611469,-38.162731172,5.59815215178));
#65875=CARTESIAN_POINT('Ctrl Pts',(5.35149757153,-38.2372245963,5.60065230967));
#65876=CARTESIAN_POINT('Ctrl Pts',(5.44569225468,-38.2742356128,5.60381546578));
#65877=CARTESIAN_POINT('Ctrl Pts',(5.53988693785,-38.2742356128,5.6069786219));
#65878=CARTESIAN_POINT('Ctrl Pts',(5.21299946948,-37.9742356128,6.40257078081));
#65879=CARTESIAN_POINT('Ctrl Pts',(5.21299946951,-38.068483391,6.40257077998));
#65880=CARTESIAN_POINT('Ctrl Pts',(5.24979957977,-38.1627311691,6.40947213682));
#65881=CARTESIAN_POINT('Ctrl Pts',(5.32386850147,-38.2372245928,6.42336289407));
#65882=CARTESIAN_POINT('Ctrl Pts',(5.41757921002,-38.2742356105,6.4409371779));
#65883=CARTESIAN_POINT('Ctrl Pts',(5.51128991946,-38.2742356128,6.4585114621));
#65884=CARTESIAN_POINT('Ctrl Pts',(5.03157376442,-37.9742356128,7.20293447587));
#65885=CARTESIAN_POINT('Ctrl Pts',(5.03157368764,-38.0684833946,7.20293453622));
#65886=CARTESIAN_POINT('Ctrl Pts',(5.06709410499,-38.1627311763,7.21553462796));
#65887=CARTESIAN_POINT('Ctrl Pts',(5.13858744567,-38.2372246013,7.24089500381));
#65888=CARTESIAN_POINT('Ctrl Pts',(5.22903961522,-38.2742356162,7.27298056211));
#65889=CARTESIAN_POINT('Ctrl Pts',(5.31949181364,-38.2742356128,7.30506609664));
#65890=CARTESIAN_POINT('Ctrl Pts',(4.69583353882,-37.9742356128,7.95822794629));
#65891=CARTESIAN_POINT('Ctrl Pts',(4.69583375753,-38.0684833911,7.9582276781));
#65892=CARTESIAN_POINT('Ctrl Pts',(4.72897185598,-38.1627311693,7.97614326012));
#65893=CARTESIAN_POINT('Ctrl Pts',(4.79566992348,-38.237224593,8.01220298795));
#65894=CARTESIAN_POINT('Ctrl Pts',(4.88005499,-38.2742356106,8.0578252665));
#65895=CARTESIAN_POINT('Ctrl Pts',(4.96443997088,-38.2742356128,8.10344765091));
#65896=CARTESIAN_POINT('Ctrl Pts',(3.75205884826,-37.9742356128,9.30126426068));
#65897=CARTESIAN_POINT('Ctrl Pts',(3.75205862954,-38.0684833938,9.30126452888));
#65898=CARTESIAN_POINT('Ctrl Pts',(3.77854861256,-38.1627311749,9.32865838142));
#65899=CARTESIAN_POINT('Ctrl Pts',(3.83186616208,-38.2372245996,9.38379460661));
#65900=CARTESIAN_POINT('Ctrl Pts',(3.89932275841,-38.274235615,9.45355185547));
#65901=CARTESIAN_POINT('Ctrl Pts',(3.9667794404,-38.2742356128,9.52330899846));
#65902=CARTESIAN_POINT('Ctrl Pts',(2.37813062282,-37.9742356128,10.1995581826));
#65903=CARTESIAN_POINT('Ctrl Pts',(2.37813084155,-38.068483391,10.1995579144));
#65904=CARTESIAN_POINT('Ctrl Pts',(2.39492734371,-38.1627311693,10.2332766055));
#65905=CARTESIAN_POINT('Ctrl Pts',(2.42873408312,-38.237224593,10.3011438287));
#65906=CARTESIAN_POINT('Ctrl Pts',(2.4715056159,-38.2742356106,10.3870083947));
#65907=CARTESIAN_POINT('Ctrl Pts',(2.51427706302,-38.2742356128,10.4728730665));
#65908=CARTESIAN_POINT('Ctrl Pts',(1.61217671584,-37.9742356128,10.5097230164));
#65909=CARTESIAN_POINT('Ctrl Pts',(1.61217703526,-38.0684834004,10.5097230175));
#65910=CARTESIAN_POINT('Ctrl Pts',(1.62357348219,-38.162731188,10.5456455438));
#65911=CARTESIAN_POINT('Ctrl Pts',(1.64651083532,-38.2372246151,10.6179481209));
#65912=CARTESIAN_POINT('Ctrl Pts',(1.67553070609,-38.2742356254,10.7094240756));
#65913=CARTESIAN_POINT('Ctrl Pts',(1.70455045076,-38.2742356128,10.8009000251));
#65914=CARTESIAN_POINT('Ctrl Pts',(0.806141183123,-37.9742356128,10.6642820769));
#65915=CARTESIAN_POINT('Ctrl Pts',(0.806141182686,-38.0684833912,10.6642820769));
#65916=CARTESIAN_POINT('Ctrl Pts',(0.811810207047,-38.1627311695,10.7012926437));
#65917=CARTESIAN_POINT('Ctrl Pts',(0.823220660712,-38.2372245933,10.7757851643));
#65918=CARTESIAN_POINT('Ctrl Pts',(0.837656883379,-38.2742356108,10.8700318005));
#65919=CARTESIAN_POINT('Ctrl Pts',(0.852093106215,-38.2742356128,10.9642784374));
#65920=CARTESIAN_POINT('Ctrl Pts',(6.88994417075E-10,-37.9742356128,10.6643459842));
#65921=CARTESIAN_POINT('Ctrl Pts',(6.97641722169E-10,-38.0684833925,10.6643459842));
#65922=CARTESIAN_POINT('Ctrl Pts',(2.97494488111E-6,-38.1627311721,10.7013570005));
#65923=CARTESIAN_POINT('Ctrl Pts',(8.96131032624E-6,-38.2372245964,10.7758504244));
#65924=CARTESIAN_POINT('Ctrl Pts',(1.65351501034E-5,-38.2742356129,10.8700982036));
#65925=CARTESIAN_POINT('Ctrl Pts',(2.41089864841E-5,-38.2742356128,10.9643459827));
#65926=CARTESIAN_POINT('',(5.24005595186,-37.9742356128,5.596909982745));
#65927=CARTESIAN_POINT('Ctrl Pts',(6.88994195030546E-10,-37.9742356128,
10.6643459842));
#65928=CARTESIAN_POINT('Ctrl Pts',(0.148543738141462,-37.9742356128,10.6643342083109));
#65929=CARTESIAN_POINT('Ctrl Pts',(0.297086910377638,-37.9742356128,10.6580232678524));
#65930=CARTESIAN_POINT('Ctrl Pts',(0.445090815547211,-37.9742356128,10.6454233478295));
#65931=CARTESIAN_POINT('Ctrl Pts',(0.59487372187678,-37.9742356128,10.63267197726));
#65932=CARTESIAN_POINT('Ctrl Pts',(0.744104091924914,-37.9742356128,10.6134795752124));
#65933=CARTESIAN_POINT('Ctrl Pts',(0.892229989798875,-37.9742356128,10.5879098461637));
#65934=CARTESIAN_POINT('Ctrl Pts',(1.04131204338439,-37.9742356128,10.5621750639892));
#65935=CARTESIAN_POINT('Ctrl Pts',(1.1892750857725,-37.9742356128,10.5299804567442));
#65936=CARTESIAN_POINT('Ctrl Pts',(1.33556638280071,-37.9742356128,10.4914433340022));
#65937=CARTESIAN_POINT('Ctrl Pts',(1.4826794306896,-37.9742356128,10.4526897396422));
#65938=CARTESIAN_POINT('Ctrl Pts',(1.62810165638871,-37.9742356128,10.4075222877044));
#65939=CARTESIAN_POINT('Ctrl Pts',(1.77128460050933,-37.9742356128,10.3561114475755));
#65940=CARTESIAN_POINT('Ctrl Pts',(1.91512843540153,-37.9742356128,10.3044633099808));
#65941=CARTESIAN_POINT('Ctrl Pts',(2.05671201996512,-37.9742356128,10.2465141426538));
#65942=CARTESIAN_POINT('Ctrl Pts',(2.19549670562412,-37.9742356128,10.182486467514));
#65943=CARTESIAN_POINT('Ctrl Pts',(2.33495214390865,-37.9742356128,10.1181493437415));
#65944=CARTESIAN_POINT('Ctrl Pts',(2.4715813047956,-37.9742356128,10.0476749455133));
#65945=CARTESIAN_POINT('Ctrl Pts',(2.6048590942595,-37.9742356128,9.97133714374602));
#65946=CARTESIAN_POINT('Ctrl Pts',(2.73831338899758,-37.9742356128,9.89489824467904));
#65947=CARTESIAN_POINT('Ctrl Pts',(2.86840717985693,-37.9742356128,9.81258056317965));
#65948=CARTESIAN_POINT('Ctrl Pts',(2.99463849904681,-37.9742356128,9.72470493579735));
#65949=CARTESIAN_POINT('Ctrl Pts',(3.12086957170909,-37.9742356128,9.63682948003464));
#65950=CARTESIAN_POINT('Ctrl Pts',(3.24323794320094,-37.9742356128,9.54339627268128));
#65951=CARTESIAN_POINT('Ctrl Pts',(3.36127054935203,-37.9742356128,9.44476947023749));
#65952=CARTESIAN_POINT('Ctrl Pts',(3.45873626436591,-37.9742356128,9.36332814539365));
#65953=CARTESIAN_POINT('Ctrl Pts',(3.55324602203091,-37.9742356128,9.27834630722957));
#65954=CARTESIAN_POINT('Ctrl Pts',(3.64455010326812,-37.9742356128,9.19005000034558));
#65955=CARTESIAN_POINT('Ctrl Pts',(3.75483187955168,-37.9742356128,9.08340116898452));
#65956=CARTESIAN_POINT('Ctrl Pts',(3.86043575496047,-37.9742356128,8.97191598143711));
#65957=CARTESIAN_POINT('Ctrl Pts',(3.96095362281167,-37.9742356128,8.85602145332094));
#65958=CARTESIAN_POINT('Ctrl Pts',(4.06169428001623,-37.9742356128,8.73987005478434));
#65959=CARTESIAN_POINT('Ctrl Pts',(4.15732614237061,-37.9742356128,8.61929000585443));
#65960=CARTESIAN_POINT('Ctrl Pts',(4.24747728584571,-37.9742356128,8.49474609398298));
#65961=CARTESIAN_POINT('Ctrl Pts',(4.33754043554632,-37.9742356128,8.3703237456156));
#65962=CARTESIAN_POINT('Ctrl Pts',(4.42213336493615,-37.9742356128,8.24194554434444));
#65963=CARTESIAN_POINT('Ctrl Pts',(4.50092708273691,-37.9742356128,8.11010570734388));
#65964=CARTESIAN_POINT('Ctrl Pts',(4.5795067479302,-37.9742356128,7.97862402911112));
#65965=CARTESIAN_POINT('Ctrl Pts',(4.65231848790631,-37.9742356128,7.84369977752986));
#65966=CARTESIAN_POINT('Ctrl Pts',(4.71908040770882,-37.9742356128,7.70584961888401));
#65967=CARTESIAN_POINT('Ctrl Pts',(4.78555342045735,-37.9742356128,7.56859599615778));
#65968=CARTESIAN_POINT('Ctrl Pts',(4.8460286985358,-37.9742356128,7.42844201386812));
#65969=CARTESIAN_POINT('Ctrl Pts',(4.90027461525642,-37.9742356128,7.28591974913334));
#65970=CARTESIAN_POINT('Ctrl Pts',(4.95401280665947,-37.9742356128,7.14473144954282));
#65971=CARTESIAN_POINT('Ctrl Pts',(5.00163758895503,-37.9742356128,7.0012192733805));
#65972=CARTESIAN_POINT('Ctrl Pts',(5.04297160369282,-37.9742356128,6.85591803740467));
#65973=CARTESIAN_POINT('Ctrl Pts',(5.08404289066266,-37.9742356128,6.71154036691482));
#65974=CARTESIAN_POINT('Ctrl Pts',(5.11890299934201,-37.9742356128,6.56539656577722));
#65975=CARTESIAN_POINT('Ctrl Pts',(5.14742718798799,-37.9742356128,6.41802472866415));
#65976=CARTESIAN_POINT('Ctrl Pts',(5.17562330555142,-37.9742356128,6.27234788939091));
#65977=CARTESIAN_POINT('Ctrl Pts',(5.1976283358666,-37.9742356128,6.12547135028398));
#65978=CARTESIAN_POINT('Ctrl Pts',(5.21337150408987,-37.9742356128,5.9779242168455));
#65979=CARTESIAN_POINT('Ctrl Pts',(5.22688216218712,-37.9742356128,5.85130047473441));
#65980=CARTESIAN_POINT('Ctrl Pts',(5.23578174108458,-37.9742356128,5.72418307648716));
#65981=CARTESIAN_POINT('Ctrl Pts',(5.24005594912,-37.9742356128,5.5969099833));
#65982=CARTESIAN_POINT('Origin',(5.5377668413967,-37.9763569043018,5.60690742687626));
#65983=CARTESIAN_POINT('Ctrl Pts',(0.,-37.9742356128,10.664345987));
#65984=CARTESIAN_POINT('Ctrl Pts',(0.,-36.2942356128,10.664345987));
#65985=CARTESIAN_POINT('Ctrl Pts',(1.61198306736,-37.9742356128,10.6642180635));
#65986=CARTESIAN_POINT('Ctrl Pts',(1.61198306736,-36.2942356128,10.6642180635));
#65987=CARTESIAN_POINT('Ctrl Pts',(3.22524412625,-37.9742356128,10.0462831132));
#65988=CARTESIAN_POINT('Ctrl Pts',(3.22524412625,-36.2942356128,10.0462831132));
#65989=CARTESIAN_POINT('Ctrl Pts',(4.51434339457,-37.9742356128,8.79964985146));
#65990=CARTESIAN_POINT('Ctrl Pts',(4.51434339457,-36.2942356128,8.79964985146));
#65991=CARTESIAN_POINT('Ctrl Pts',(5.18595136098,-37.9742356128,7.20798481558));
#65992=CARTESIAN_POINT('Ctrl Pts',(5.18595136098,-36.2942356128,7.20798481558));
#65993=CARTESIAN_POINT('Ctrl Pts',(5.2400559546,-37.9742356128,5.59690998219));
#65994=CARTESIAN_POINT('Ctrl Pts',(5.2400559546,-36.2942356128,5.59690998219));
#65995=CARTESIAN_POINT('',(5.2400559546,-37.2742356128,5.59690998219));
#65996=CARTESIAN_POINT('Ctrl Pts',(5.53988692571,-36.2742356128,5.60697918103));
#65997=CARTESIAN_POINT('Ctrl Pts',(5.4456922481,-36.2742356128,5.60381584892));
#65998=CARTESIAN_POINT('Ctrl Pts',(5.35149757048,-36.3112466293,5.60065251681));
#65999=CARTESIAN_POINT('Ctrl Pts',(5.277046118,-36.3857400536,5.59815221981));
#66000=CARTESIAN_POINT('Ctrl Pts',(5.2400559546,-36.4799878332,5.59690998219));
#66001=CARTESIAN_POINT('Ctrl Pts',(5.2400559546,-36.5742356128,5.59690998219));
#66002=CARTESIAN_POINT('Ctrl Pts',(5.55319667202,-36.2742356128,5.21065428735));
#66003=CARTESIAN_POINT('Ctrl Pts',(5.4588608737,-36.2742356128,5.21169311262));
#66004=CARTESIAN_POINT('Ctrl Pts',(5.36452507538,-36.3112466293,5.21273193789));
#66005=CARTESIAN_POINT('Ctrl Pts',(5.28996208088,-36.3857400536,5.21355302628));
#66006=CARTESIAN_POINT('Ctrl Pts',(5.25291649976,-36.4799878332,5.21396097089));
#66007=CARTESIAN_POINT('Ctrl Pts',(5.25291649976,-36.5742356128,5.21396097089));
#66008=CARTESIAN_POINT('Ctrl Pts',(5.54519742229,-36.2742356128,4.78859077007));
#66009=CARTESIAN_POINT('Ctrl Pts',(5.45071977967,-36.2742356128,4.79882974975));
#66010=CARTESIAN_POINT('Ctrl Pts',(5.35624213705,-36.3112466293,4.80906872944));
#66011=CARTESIAN_POINT('Ctrl Pts',(5.28156702935,-36.3857400536,4.81716161496));
#66012=CARTESIAN_POINT('Ctrl Pts',(5.24446574559,-36.4799878332,4.82118245465));
#66013=CARTESIAN_POINT('Ctrl Pts',(5.24446574559,-36.5742356128,4.82118245465));
#66014=CARTESIAN_POINT('Ctrl Pts',(5.47535951132,-36.2742356128,4.37143582924));
#66015=CARTESIAN_POINT('Ctrl Pts',(5.38263787774,-36.2742356128,4.39040588335));
#66016=CARTESIAN_POINT('Ctrl Pts',(5.28991624416,-36.3112466293,4.40937593746));
#66017=CARTESIAN_POINT('Ctrl Pts',(5.21662908074,-36.3857400536,4.42436985031));
#66018=CARTESIAN_POINT('Ctrl Pts',(5.180217385,-36.4799878332,4.43181938688));
#66019=CARTESIAN_POINT('Ctrl Pts',(5.180217385,-36.5742356128,4.43181938688));
#66020=CARTESIAN_POINT('Ctrl Pts',(5.26366547685,-36.2742356128,3.57390225037));
#66021=CARTESIAN_POINT('Ctrl Pts',(5.17451246306,-36.2742356128,3.60488329763));
#66022=CARTESIAN_POINT('Ctrl Pts',(5.08535944927,-36.3112466293,3.6358643449));
#66023=CARTESIAN_POINT('Ctrl Pts',(5.01489293121,-36.3857400536,3.66035177163));
#66024=CARTESIAN_POINT('Ctrl Pts',(4.97988262013,-36.4799878332,3.67251798666));
#66025=CARTESIAN_POINT('Ctrl Pts',(4.97988262013,-36.5742356128,3.67251798666));
#66026=CARTESIAN_POINT('Ctrl Pts',(5.00219757732,-36.2742356128,2.85773196192));
#66027=CARTESIAN_POINT('Ctrl Pts',(4.91343107087,-36.2742356128,2.88936313774));
#66028=CARTESIAN_POINT('Ctrl Pts',(4.82466456442,-36.3112466293,2.92099431357));
#66029=CARTESIAN_POINT('Ctrl Pts',(4.75450353299,-36.3857400536,2.94599557417));
#66030=CARTESIAN_POINT('Ctrl Pts',(4.71964501167,-36.4799878332,2.95841712169));
#66031=CARTESIAN_POINT('Ctrl Pts',(4.71964501167,-36.5742356128,2.95841712169));
#66032=CARTESIAN_POINT('Ctrl Pts',(4.8804439272,-36.2742356128,2.50135880489));
#66033=CARTESIAN_POINT('Ctrl Pts',(4.78990764639,-36.2742356128,2.5276002033));
#66034=CARTESIAN_POINT('Ctrl Pts',(4.69937136558,-36.3112466293,2.5538416017));
#66035=CARTESIAN_POINT('Ctrl Pts',(4.62781152696,-36.3857400536,2.57458285528));
#66036=CARTESIAN_POINT('Ctrl Pts',(4.59225799479,-36.4799878332,2.58488777028));
#66037=CARTESIAN_POINT('Ctrl Pts',(4.59225799479,-36.5742356128,2.58488777028));
#66038=CARTESIAN_POINT('Ctrl Pts',(4.79845683709,-36.2742356128,2.15377208868));
#66039=CARTESIAN_POINT('Ctrl Pts',(4.70711530139,-36.2742356128,2.17743291681));
#66040=CARTESIAN_POINT('Ctrl Pts',(4.61577376569,-36.3112466293,2.20109374493));
#66041=CARTESIAN_POINT('Ctrl Pts',(4.54357742413,-36.3857400536,2.21979521964));
#66042=CARTESIAN_POINT('Ctrl Pts',(4.50770769876,-36.4799878332,2.22908684376));
#66043=CARTESIAN_POINT('Ctrl Pts',(4.50770769876,-36.5742356128,2.22908684376));
#66044=CARTESIAN_POINT('Ctrl Pts',(4.67794710935,-36.2742356128,1.76615076209));
#66045=CARTESIAN_POINT('Ctrl Pts',(4.58794861595,-36.2742356128,1.79413138544));
#66046=CARTESIAN_POINT('Ctrl Pts',(4.49795012256,-36.3112466293,1.82211200878));
#66047=CARTESIAN_POINT('Ctrl Pts',(4.42681533316,-36.3857400536,1.84422788732));
#66048=CARTESIAN_POINT('Ctrl Pts',(4.39147300745,-36.4799878332,1.85521585242));
#66049=CARTESIAN_POINT('Ctrl Pts',(4.39147300745,-36.5742356128,1.85521585242));
#66050=CARTESIAN_POINT('Ctrl Pts',(4.67555993961595,-36.2742356128,1.75847239523564));
#66051=CARTESIAN_POINT('Ctrl Pts',(4.5855880504577,-36.2742356128,1.78653858914164));
#66052=CARTESIAN_POINT('Ctrl Pts',(4.49561616130965,-36.3112466293,1.81460478303764));
#66053=CARTESIAN_POINT('Ctrl Pts',(4.42450240013065,-36.3857400536,1.83678829729166));
#66054=CARTESIAN_POINT('Ctrl Pts',(4.38917052164785,-36.4799878332,1.84780986510509));
#66055=CARTESIAN_POINT('Ctrl Pts',(4.38917052164785,-36.5742356128,1.84780986510509));
#66056=CARTESIAN_POINT('Ctrl Pts',(4.6731727698819,-36.2742356128,1.75079402838127));
#66057=CARTESIAN_POINT('Ctrl Pts',(4.5832274849654,-36.2742356128,1.77894579284327));
#66058=CARTESIAN_POINT('Ctrl Pts',(4.4932822000593,-36.3112466293,1.80709755729528));
#66059=CARTESIAN_POINT('Ctrl Pts',(4.4221894671013,-36.3857400536,1.82934870726333));
#66060=CARTESIAN_POINT('Ctrl Pts',(4.38686803584571,-36.4799878332,1.84040387779018));
#66061=CARTESIAN_POINT('Ctrl Pts',(4.38686803584571,-36.5742356128,1.84040387779018));
#66062=CARTESIAN_POINT('Ctrl Pts',(4.67078560014785,-36.2742356128,1.7431156615269));
#66063=CARTESIAN_POINT('Ctrl Pts',(4.58086691947311,-36.2742356128,1.77135299654491));
#66064=CARTESIAN_POINT('Ctrl Pts',(4.49094823880895,-36.3112466293,1.79959033155291));
#66065=CARTESIAN_POINT('Ctrl Pts',(4.41987653407195,-36.3857400536,1.821909117235));
#66066=CARTESIAN_POINT('Ctrl Pts',(4.38456555004357,-36.4799878332,1.83299789047527));
#66067=CARTESIAN_POINT('Ctrl Pts',(4.38456555004357,-36.5742356128,1.83299789047527));
#66068=CARTESIAN_POINT('Ctrl Pts',(4.6683984304138,-36.2742356128,1.73543729467253));
#66069=CARTESIAN_POINT('Ctrl Pts',(4.57850635398081,-36.2742356128,1.76376020024654));
#66070=CARTESIAN_POINT('Ctrl Pts',(4.4886142775586,-36.3112466293,1.79208310581055));
#66071=CARTESIAN_POINT('Ctrl Pts',(4.4175636010426,-36.3857400536,1.81446952720666));
#66072=CARTESIAN_POINT('Ctrl Pts',(4.38226306424141,-36.4799878332,1.82559190316036));
#66073=CARTESIAN_POINT('Ctrl Pts',(4.38226306424141,-36.5742356128,1.82559190316036));
#66074=CARTESIAN_POINT('Ctrl Pts',(4.66601126067975,-36.2742356128,1.72775892781816));
#66075=CARTESIAN_POINT('Ctrl Pts',(4.57614578848851,-36.2742356128,1.75616740394817));
#66076=CARTESIAN_POINT('Ctrl Pts',(4.48628031630825,-36.3112466293,1.78457588006819));
#66077=CARTESIAN_POINT('Ctrl Pts',(4.41525066801324,-36.3857400536,1.80702993717832));
#66078=CARTESIAN_POINT('Ctrl Pts',(4.37996057843927,-36.4799878332,1.81818591584544));
#66079=CARTESIAN_POINT('Ctrl Pts',(4.37996057843927,-36.5742356128,1.81818591584544));
#66080=CARTESIAN_POINT('',(4.39146896866,-36.5742356128,1.85520291202));
#66081=CARTESIAN_POINT('Origin',(4.67591768253123,-36.5721143218718,1.76676845393353));
#66082=CARTESIAN_POINT('Ctrl Pts',(5.2400559546,-36.5742356128,5.59690998219));
#66083=CARTESIAN_POINT('Ctrl Pts',(5.25311376105,-36.5742356128,5.20808711269));
#66084=CARTESIAN_POINT('Ctrl Pts',(5.24470483276,-36.5742356128,4.80219931419));
#66085=CARTESIAN_POINT('Ctrl Pts',(5.17504642388,-36.5742356128,4.39981761669));
#66086=CARTESIAN_POINT('Ctrl Pts',(5.00839926013,-36.5742356128,3.79030695888));
#66087=CARTESIAN_POINT('Ctrl Pts',(4.81153097626,-36.5742356128,3.21707824383));
#66088=CARTESIAN_POINT('Ctrl Pts',(4.73686810339,-36.5742356128,3.00222967268));
#66089=CARTESIAN_POINT('Ctrl Pts',(4.62316453236,-36.5742356128,2.6499539825));
#66090=CARTESIAN_POINT('Ctrl Pts',(4.51875357768,-36.5742356128,2.29074629441));
#66091=CARTESIAN_POINT('Ctrl Pts',(4.47967500948,-36.5742356128,2.15155097848));
#66092=CARTESIAN_POINT('Ctrl Pts',(4.43790342458,-36.5742356128,2.00456060561));
#66093=CARTESIAN_POINT('Ctrl Pts',(4.39146896866,-36.5742356128,1.85520291202));
#66094=CARTESIAN_POINT('Ctrl Pts',(4.39147614152,-37.9742356128,1.85522626202));
#66095=CARTESIAN_POINT('Ctrl Pts',(4.3914761461,-38.0684833925,1.85522627644));
#66096=CARTESIAN_POINT('Ctrl Pts',(4.42681839499,-38.1627311722,1.84423808607));
#66097=CARTESIAN_POINT('Ctrl Pts',(4.49795302417,-38.2372245965,1.82212173648));
#66098=CARTESIAN_POINT('Ctrl Pts',(4.58795131206,-38.274235613,1.79414050842));
#66099=CARTESIAN_POINT('Ctrl Pts',(4.6779495981,-38.2742356128,1.76615927471));
#66100=CARTESIAN_POINT('Ctrl Pts',(4.50961312754,-37.9742356128,2.23520776943));
#66101=CARTESIAN_POINT('Ctrl Pts',(4.50961297784,-38.0684833942,2.23520729805));
#66102=CARTESIAN_POINT('Ctrl Pts',(4.54549269235,-38.1627311756,2.22594725384));
#66103=CARTESIAN_POINT('Ctrl Pts',(4.61770933618,-38.2372246005,2.20730995948));
#66104=CARTESIAN_POINT('Ctrl Pts',(4.70907664249,-38.2742356156,2.18373060025));
#66105=CARTESIAN_POINT('Ctrl Pts',(4.8004440065,-38.2742356128,2.16015142631));
#66106=CARTESIAN_POINT('Ctrl Pts',(4.59532849366,-37.9742356128,2.59792165201));
#66107=CARTESIAN_POINT('Ctrl Pts',(4.59532871153,-38.0684834119,2.59792233911));
#66108=CARTESIAN_POINT('Ctrl Pts',(4.63086911606,-38.162731211,2.58756440064));
#66109=CARTESIAN_POINT('Ctrl Pts',(4.70240224551,-38.2372246422,2.56671552146));
#66110=CARTESIAN_POINT('Ctrl Pts',(4.79290460312,-38.2742356434,2.54033756838));
#66111=CARTESIAN_POINT('Ctrl Pts',(4.88340686381,-38.2742356128,2.51395934938));
#66112=CARTESIAN_POINT('Ctrl Pts',(4.72598707696,-37.9742356128,2.97653900944));
#66113=CARTESIAN_POINT('Ctrl Pts',(4.72598702354,-38.0684833705,2.97653884209));
#66114=CARTESIAN_POINT('Ctrl Pts',(4.76081453341,-38.1627311281,2.96403785534));
#66115=CARTESIAN_POINT('Ctrl Pts',(4.83091321213,-38.2372245445,2.93887706303));
#66116=CARTESIAN_POINT('Ctrl Pts',(4.91960087198,-38.2742355783,2.90704408516));
#66117=CARTESIAN_POINT('Ctrl Pts',(5.00828856587,-38.2742356128,2.87521116975));
#66118=CARTESIAN_POINT('Ctrl Pts',(4.98677022447,-37.9742356128,3.69093161808));
#66119=CARTESIAN_POINT('Ctrl Pts',(4.98677027514,-38.0684834133,3.69093177682));
#66120=CARTESIAN_POINT('Ctrl Pts',(5.02181898916,-38.1627312138,3.6788456217));
#66121=CARTESIAN_POINT('Ctrl Pts',(5.09236274059,-38.2372246455,3.65451899528));
#66122=CARTESIAN_POINT('Ctrl Pts',(5.18161342975,-38.2742356456,3.62374135649));
#66123=CARTESIAN_POINT('Ctrl Pts',(5.27086408663,-38.2742356128,3.59296365845));
#66124=CARTESIAN_POINT('Ctrl Pts',(5.18352491332,-37.9742356128,4.45190028227));
#66125=CARTESIAN_POINT('Ctrl Pts',(5.18352486526,-38.0684833727,4.4519001317));
#66126=CARTESIAN_POINT('Ctrl Pts',(5.21997029761,-38.1627311325,4.44462444175));
#66127=CARTESIAN_POINT('Ctrl Pts',(5.29332542209,-38.2372245497,4.42998075713));
#66128=CARTESIAN_POINT('Ctrl Pts',(5.38613307587,-38.2742355818,4.41145383762));
#66129=CARTESIAN_POINT('Ctrl Pts',(5.47894076028,-38.2742356128,4.39292697431));
#66130=CARTESIAN_POINT('Ctrl Pts',(5.24475584762,-37.9742356128,4.83460482733));
#66131=CARTESIAN_POINT('Ctrl Pts',(5.24475584748,-38.0684834044,4.83460481263));
#66132=CARTESIAN_POINT('Ctrl Pts',(5.281854554,-38.1627311959,4.83070605882));
#66133=CARTESIAN_POINT('Ctrl Pts',(5.35652449165,-38.2372246244,4.82285841894));
#66134=CARTESIAN_POINT('Ctrl Pts',(5.45099558138,-38.2742356315,4.81292993959));
#66135=CARTESIAN_POINT('Ctrl Pts',(5.54546666392,-38.2742356128,4.80300146625));
#66136=CARTESIAN_POINT('Ctrl Pts',(5.2526976354,-37.9742356128,5.22047810427));
#66137=CARTESIAN_POINT('Ctrl Pts',(5.2526976354,-38.0684833924,5.22047810427));
#66138=CARTESIAN_POINT('Ctrl Pts',(5.28974227713,-38.1627311721,5.22009813259));
#66139=CARTESIAN_POINT('Ctrl Pts',(5.36430336964,-38.2372245963,5.21933367912));
#66140=CARTESIAN_POINT('Ctrl Pts',(5.45863676635,-38.2742356128,5.21836636703));
#66141=CARTESIAN_POINT('Ctrl Pts',(5.55297016303,-38.2742356128,5.21739905525));
#66142=CARTESIAN_POINT('Ctrl Pts',(5.2400559546,-37.9742356128,5.59690998219));
#66143=CARTESIAN_POINT('Ctrl Pts',(5.2400559546,-38.0684833924,5.59690998219));
#66144=CARTESIAN_POINT('Ctrl Pts',(5.277046118,-38.1627311721,5.59815221981));
#66145=CARTESIAN_POINT('Ctrl Pts',(5.35149757048,-38.2372245963,5.60065251681));
#66146=CARTESIAN_POINT('Ctrl Pts',(5.4456922481,-38.2742356128,5.60381584892));
#66147=CARTESIAN_POINT('Ctrl Pts',(5.53988692571,-38.2742356128,5.60697918103));
#66148=CARTESIAN_POINT('',(4.3914713655969,-37.9742356128,1.85521069141137));
#66149=CARTESIAN_POINT('Ctrl Pts',(5.2400559546,-37.9742356128,5.59690998219));
#66150=CARTESIAN_POINT('Ctrl Pts',(5.2418605608663,-37.9742356128,5.54317414306575));
#66151=CARTESIAN_POINT('Ctrl Pts',(5.24315737610566,-37.9742356128,5.48920776658016));
#66152=CARTESIAN_POINT('Ctrl Pts',(5.24376788585,-37.9742356128,5.43508810427703));
#66153=CARTESIAN_POINT('Ctrl Pts',(5.24439174263741,-37.9742356128,5.37978527090855));
#66154=CARTESIAN_POINT('Ctrl Pts',(5.24429909977124,-37.9742356128,5.32432243841033));
#66155=CARTESIAN_POINT('Ctrl Pts',(5.24335412274884,-37.9742356128,5.26877728160842));
#66156=CARTESIAN_POINT('Ctrl Pts',(5.24238610864014,-37.9742356128,5.2118780193198));
#66157=CARTESIAN_POINT('Ctrl Pts',(5.24052385945121,-37.9742356128,5.15489244461267));
#66158=CARTESIAN_POINT('Ctrl Pts',(5.23767577778745,-37.9742356128,5.0978980588865));
#66159=CARTESIAN_POINT('Ctrl Pts',(5.23470185843848,-37.9742356128,5.03838547234427));
#66160=CARTESIAN_POINT('Ctrl Pts',(5.23065312103343,-37.9742356128,4.97886339674345));
#66161=CARTESIAN_POINT('Ctrl Pts',(5.22548247270875,-37.9742356128,4.91941208132394));
#66162=CARTESIAN_POINT('Ctrl Pts',(5.22014830848689,-37.9742356128,4.85808068538671));
#66163=CARTESIAN_POINT('Ctrl Pts',(5.21362040513255,-37.9742356128,4.7968247209684));
#66164=CARTESIAN_POINT('Ctrl Pts',(5.20590409543257,-37.9742356128,4.73572210301911));
#66165=CARTESIAN_POINT('Ctrl Pts',(5.19790447046991,-37.9742356128,4.67237601572666));
#66166=CARTESIAN_POINT('Ctrl Pts',(5.18862788453177,-37.9742356128,4.60919490621015));
#66167=CARTESIAN_POINT('Ctrl Pts',(5.17813629890928,-37.9742356128,4.54625254168015));
#66168=CARTESIAN_POINT('Ctrl Pts',(5.16719017838142,-37.9742356128,4.48058327744837));
#66169=CARTESIAN_POINT('Ctrl Pts',(5.15492191671971,-37.9742356128,4.41517411713375));
#66170=CARTESIAN_POINT('Ctrl Pts',(5.14145615885331,-37.9742356128,4.35009182413807));
#66171=CARTESIAN_POINT('Ctrl Pts',(5.12692746384431,-37.9742356128,4.27987217554486));
#66172=CARTESIAN_POINT('Ctrl Pts',(5.11100518230485,-37.9742356128,4.21003348647402));
#66173=CARTESIAN_POINT('Ctrl Pts',(5.09390154139431,-37.9742356128,4.14063468475526));
#66174=CARTESIAN_POINT('Ctrl Pts',(5.07529743225982,-37.9742356128,4.06514766490191));
#66175=CARTESIAN_POINT('Ctrl Pts',(5.05529654521998,-37.9742356128,3.99018183403256));
#66176=CARTESIAN_POINT('Ctrl Pts',(5.03422469803328,-37.9742356128,3.91577491776497));
#66177=CARTESIAN_POINT('Ctrl Pts',(5.01581896365487,-37.9742356128,3.85078232719598));
#66178=CARTESIAN_POINT('Ctrl Pts',(4.99659773718505,-37.9742356128,3.78621567165843));
#66179=CARTESIAN_POINT('Ctrl Pts',(4.9767959506457,-37.9742356128,3.72207308531392));
#66180=CARTESIAN_POINT('Ctrl Pts',(4.95996155632885,-37.9742356128,3.66754257167158));
#66181=CARTESIAN_POINT('Ctrl Pts',(4.94270644688682,-37.9742356128,3.6133124923039));
#66182=CARTESIAN_POINT('Ctrl Pts',(4.92516971522254,-37.9742356128,3.55925405827158));
#66183=CARTESIAN_POINT('Ctrl Pts',(4.90642740291784,-37.9742356128,3.50147932163688));
#66184=CARTESIAN_POINT('Ctrl Pts',(4.88736441624655,-37.9742356128,3.44390092271876));
#66185=CARTESIAN_POINT('Ctrl Pts',(4.86816362318974,-37.9742356128,3.38642084337562));
#66186=CARTESIAN_POINT('Ctrl Pts',(4.84680217663087,-37.9742356128,3.32247256585111));
#66187=CARTESIAN_POINT('Ctrl Pts',(4.82527213582349,-37.9742356128,3.25864633151042));
#66188=CARTESIAN_POINT('Ctrl Pts',(4.80381712909044,-37.9742356128,3.19487377343086));
#66189=CARTESIAN_POINT('Ctrl Pts',(4.78399437868539,-37.9742356128,3.13595291093793));
#66190=CARTESIAN_POINT('Ctrl Pts',(4.76423690135756,-37.9742356128,3.07707965248936));
#66191=CARTESIAN_POINT('Ctrl Pts',(4.74470721823347,-37.9742356128,3.01823474641582));
#66192=CARTESIAN_POINT('Ctrl Pts',(4.72646159352314,-37.9742356128,2.96325883792256));
#66193=CARTESIAN_POINT('Ctrl Pts',(4.7084154678586,-37.9742356128,2.9083087377769));
#66194=CARTESIAN_POINT('Ctrl Pts',(4.69066177721658,-37.9742356128,2.85338122442281));
#66195=CARTESIAN_POINT('Ctrl Pts',(4.67394673917456,-37.9742356128,2.80166716148346));
#66196=CARTESIAN_POINT('Ctrl Pts',(4.65749130213224,-37.9742356128,2.74997378582983));
#66197=CARTESIAN_POINT('Ctrl Pts',(4.64132952175512,-37.9742356128,2.69829811051436));
#66198=CARTESIAN_POINT('Ctrl Pts',(4.62594632441804,-37.9742356128,2.64911187655035));
#66199=CARTESIAN_POINT('Ctrl Pts',(4.61082943066444,-37.9742356128,2.5999421252798));
#66200=CARTESIAN_POINT('Ctrl Pts',(4.59596307105996,-37.9742356128,2.55077829977098));
#66201=CARTESIAN_POINT('Ctrl Pts',(4.58169099754295,-37.9742356128,2.50357980930611));
#66202=CARTESIAN_POINT('Ctrl Pts',(4.56765002431437,-37.9742356128,2.4563871039601));
#66203=CARTESIAN_POINT('Ctrl Pts',(4.55378028303625,-37.9742356128,2.40917787062285));
#66204=CARTESIAN_POINT('Ctrl Pts',(4.54031359363548,-37.9742356128,2.36334052806158));
#66205=CARTESIAN_POINT('Ctrl Pts',(4.52700852277083,-37.9742356128,2.3174878454883));
#66206=CARTESIAN_POINT('Ctrl Pts',(4.51376315077643,-37.9742356128,2.27158273796349));
#66207=CARTESIAN_POINT('Ctrl Pts',(4.50111844828701,-37.9742356128,2.22775939894054));
#66208=CARTESIAN_POINT('Ctrl Pts',(4.48852817727415,-37.9742356128,2.1838885088515));
#66209=CARTESIAN_POINT('Ctrl Pts',(4.4758590226742,-37.9742356128,2.1399200426657));
#66210=CARTESIAN_POINT('Ctrl Pts',(4.4634537013424,-37.9742356128,2.09686721327618));
#66211=CARTESIAN_POINT('Ctrl Pts',(4.45097289120161,-37.9742356128,2.05372100321262));
#66212=CARTESIAN_POINT('Ctrl Pts',(4.43824617315795,-37.9742356128,2.0104141381816));
#66213=CARTESIAN_POINT('Ctrl Pts',(4.42584830060044,-37.9742356128,1.9682262786189));
#66214=CARTESIAN_POINT('Ctrl Pts',(4.41321713264896,-37.9742356128,1.92588608013858));
#66215=CARTESIAN_POINT('Ctrl Pts',(4.40015024268932,-37.9742356128,1.8833097637315));
#66216=CARTESIAN_POINT('Ctrl Pts',(4.39728088028414,-37.9742356128,1.87396041725143));
#66217=CARTESIAN_POINT('Ctrl Pts',(4.39439032942952,-37.9742356128,1.86459959675658));
#66218=CARTESIAN_POINT('Ctrl Pts',(4.39147614152,-37.9742356128,1.85522626202));
#66219=CARTESIAN_POINT('Ctrl Pts',(4.6779495981,-38.2742356128,1.76615927471));
#66220=CARTESIAN_POINT('Ctrl Pts',(4.58794136979949,-38.2742356128,1.79410813492836));
#66221=CARTESIAN_POINT('Ctrl Pts',(4.4979443455795,-38.2372245963,1.82209348096837));
#66222=CARTESIAN_POINT('Ctrl Pts',(4.4268107174295,-38.1627311721,1.84421309232839));
#66223=CARTESIAN_POINT('Ctrl Pts',(4.3914689686595,-38.0684833924,1.8552029120184));
#66224=CARTESIAN_POINT('Ctrl Pts',(4.39146896866,-37.9742356128,1.85520291202));
#66225=CARTESIAN_POINT('Ctrl Pts',(5.2400559546,-37.9742356128,5.59690998219));
#66226=CARTESIAN_POINT('Ctrl Pts',(5.2400559546,-36.2942356128,5.59690998219));
#66227=CARTESIAN_POINT('Ctrl Pts',(5.25311376105,-37.9742356128,5.20808711269));
#66228=CARTESIAN_POINT('Ctrl Pts',(5.25311376105,-36.2942356128,5.20808711269));
#66229=CARTESIAN_POINT('Ctrl Pts',(5.24470483276,-37.9742356128,4.80219931419));
#66230=CARTESIAN_POINT('Ctrl Pts',(5.24470483276,-36.2942356128,4.80219931419));
#66231=CARTESIAN_POINT('Ctrl Pts',(5.17504642388,-37.9742356128,4.39981761669));
#66232=CARTESIAN_POINT('Ctrl Pts',(5.17504642388,-36.2942356128,4.39981761669));
#66233=CARTESIAN_POINT('Ctrl Pts',(5.00839926013,-37.9742356128,3.79030695888));
#66234=CARTESIAN_POINT('Ctrl Pts',(5.00839926013,-36.2942356128,3.79030695888));
#66235=CARTESIAN_POINT('Ctrl Pts',(4.81153097626,-37.9742356128,3.21707824383));
#66236=CARTESIAN_POINT('Ctrl Pts',(4.81153097626,-36.2942356128,3.21707824383));
#66237=CARTESIAN_POINT('Ctrl Pts',(4.73686810339,-37.9742356128,3.00222967268));
#66238=CARTESIAN_POINT('Ctrl Pts',(4.73686810339,-36.2942356128,3.00222967268));
#66239=CARTESIAN_POINT('Ctrl Pts',(4.62316453236,-37.9742356128,2.6499539825));
#66240=CARTESIAN_POINT('Ctrl Pts',(4.62316453236,-36.2942356128,2.6499539825));
#66241=CARTESIAN_POINT('Ctrl Pts',(4.51875357768,-37.9742356128,2.29074629441));
#66242=CARTESIAN_POINT('Ctrl Pts',(4.51875357768,-36.2942356128,2.29074629441));
#66243=CARTESIAN_POINT('Ctrl Pts',(4.47967500948,-37.9742356128,2.15155097848));
#66244=CARTESIAN_POINT('Ctrl Pts',(4.47967500948,-36.2942356128,2.15155097848));
#66245=CARTESIAN_POINT('Ctrl Pts',(4.43790342458,-37.9742356128,2.00456060561));
#66246=CARTESIAN_POINT('Ctrl Pts',(4.43790342458,-36.2942356128,2.00456060561));
#66247=CARTESIAN_POINT('Ctrl Pts',(4.39146896866,-37.9742356128,1.85520291202));
#66248=CARTESIAN_POINT('Ctrl Pts',(4.39146896866,-36.2942356128,1.85520291202));
#66249=CARTESIAN_POINT('',(4.39146896866,-37.2742356128,1.85520291202));
#66250=CARTESIAN_POINT('Ctrl Pts',(4.67793839402,-36.2742356128,1.76612278889));
#66251=CARTESIAN_POINT('Ctrl Pts',(4.5879413698,-36.2742356128,1.79410813493));
#66252=CARTESIAN_POINT('Ctrl Pts',(4.49794434558,-36.3112466293,1.82209348097));
#66253=CARTESIAN_POINT('Ctrl Pts',(4.42681071743,-36.3857400536,1.84421309233));
#66254=CARTESIAN_POINT('Ctrl Pts',(4.39146896866,-36.4799878332,1.85520291202));
#66255=CARTESIAN_POINT('Ctrl Pts',(4.39146896866,-36.5742356128,1.85520291202));
#66256=CARTESIAN_POINT('Ctrl Pts',(4.57998241553,-36.2742356128,1.45110983336));
#66257=CARTESIAN_POINT('Ctrl Pts',(4.49109393546,-36.2742356128,1.48266010491));
#66258=CARTESIAN_POINT('Ctrl Pts',(4.40220545538,-36.3112466293,1.51421037645));
#66259=CARTESIAN_POINT('Ctrl Pts',(4.33194802025,-36.3857400536,1.5391477041));
#66260=CARTESIAN_POINT('Ctrl Pts',(4.29704159577,-36.4799878332,1.5515374668));
#66261=CARTESIAN_POINT('Ctrl Pts',(4.29704159577,-36.5742356128,1.5515374668));
#66262=CARTESIAN_POINT('Ctrl Pts',(4.46666859078,-36.2742356128,1.14155311765));
#66263=CARTESIAN_POINT('Ctrl Pts',(4.3790579831,-36.2742356128,1.17661454934));
#66264=CARTESIAN_POINT('Ctrl Pts',(4.29144737541,-36.3112466293,1.21167598103));
#66265=CARTESIAN_POINT('Ctrl Pts',(4.22219997042,-36.3857400536,1.23938852904));
#66266=CARTESIAN_POINT('Ctrl Pts',(4.18779536517,-36.4799878332,1.25315712095));
#66267=CARTESIAN_POINT('Ctrl Pts',(4.18779536517,-36.5742356128,1.25315712095));
#66268=CARTESIAN_POINT('Ctrl Pts',(4.33903994549,-36.2742356128,0.842275524713));
#66269=CARTESIAN_POINT('Ctrl Pts',(4.25305209744,-36.2742356128,0.881099274512));
#66270=CARTESIAN_POINT('Ctrl Pts',(4.16706424939,-36.3112466293,0.919923024311));
#66271=CARTESIAN_POINT('Ctrl Pts',(4.09909947328,-36.3857400536,0.950609307675));
#66272=CARTESIAN_POINT('Ctrl Pts',(4.06533212422,-36.4799878332,0.96585535851));
#66273=CARTESIAN_POINT('Ctrl Pts',(4.06533212422,-36.5742356128,0.96585535851));
#66274=CARTESIAN_POINT('Ctrl Pts',(4.09052289333,-36.2742356128,0.331506343655));
#66275=CARTESIAN_POINT('Ctrl Pts',(4.00737841693,-36.2742356128,0.37623718636));
#66276=CARTESIAN_POINT('Ctrl Pts',(3.92423394053,-36.3112466293,0.420968029064));
#66277=CARTESIAN_POINT('Ctrl Pts',(3.8585165647,-36.3857400536,0.456323277416));
#66278=CARTESIAN_POINT('Ctrl Pts',(3.82586580513,-36.4799878332,0.473889038156));
#66279=CARTESIAN_POINT('Ctrl Pts',(3.82586580513,-36.5742356128,0.473889038156));
#66280=CARTESIAN_POINT('Ctrl Pts',(3.79239464833,-36.2742356128,-0.161386595149));
#66281=CARTESIAN_POINT('Ctrl Pts',(3.71291098531,-36.2742356128,-0.110612175752));
#66282=CARTESIAN_POINT('Ctrl Pts',(3.6334273223,-36.3112466293,-0.0598377563554));
#66283=CARTESIAN_POINT('Ctrl Pts',(3.57060345243,-36.3857400536,-0.0197056666316));
#66284=CARTESIAN_POINT('Ctrl Pts',(3.53939029105,-36.4799878332,0.000233401443254));
#66285=CARTESIAN_POINT('Ctrl Pts',(3.53939029105,-36.5742356128,0.000233401443254));
#66286=CARTESIAN_POINT('Ctrl Pts',(3.65536373033,-36.2742356128,-0.369783971346));
#66287=CARTESIAN_POINT('Ctrl Pts',(3.57749719054,-36.2742356128,-0.316462440475));
#66288=CARTESIAN_POINT('Ctrl Pts',(3.49963065075,-36.3112466293,-0.263140909604));
#66289=CARTESIAN_POINT('Ctrl Pts',(3.43808495466,-36.3857400536,-0.220995583714));
#66290=CARTESIAN_POINT('Ctrl Pts',(3.40750683616,-36.4799878332,-0.200056267119));
#66291=CARTESIAN_POINT('Ctrl Pts',(3.40750683616,-36.5742356128,-0.200056267119));
#66292=CARTESIAN_POINT('Ctrl Pts',(3.30318535597,-36.2742356128,-0.851087598324));
#66293=CARTESIAN_POINT('Ctrl Pts',(3.23120788587,-36.2742356128,-0.789523577996));
#66294=CARTESIAN_POINT('Ctrl Pts',(3.15923041576,-36.3112466293,-0.727959557669));
#66295=CARTESIAN_POINT('Ctrl Pts',(3.10233943926,-36.3857400536,-0.679299369581));
#66296=CARTESIAN_POINT('Ctrl Pts',(3.0740739528,-36.4799878332,-0.65512323529));
#66297=CARTESIAN_POINT('Ctrl Pts',(3.0740739528,-36.5742356128,-0.65512323529));
#66298=CARTESIAN_POINT('Ctrl Pts',(2.87113584445,-36.2742356128,-1.27814713268));
#66299=CARTESIAN_POINT('Ctrl Pts',(2.80938320589,-36.2742356128,-1.20614411812));
#66300=CARTESIAN_POINT('Ctrl Pts',(2.74763056733,-36.3112466293,-1.13414110356));
#66301=CARTESIAN_POINT('Ctrl Pts',(2.69882129557,-36.3857400536,-1.07722993587));
#66302=CARTESIAN_POINT('Ctrl Pts',(2.67457109093,-36.4799878332,-1.04895441899));
#66303=CARTESIAN_POINT('Ctrl Pts',(2.67457109093,-36.5742356128,-1.04895441899));
#66304=CARTESIAN_POINT('Ctrl Pts',(2.59469364023,-36.2742356128,-1.49279721696));
#66305=CARTESIAN_POINT('Ctrl Pts',(2.54027280659,-36.2742356128,-1.41505897416));
#66306=CARTESIAN_POINT('Ctrl Pts',(2.48585197294,-36.3112466293,-1.33732073137));
#66307=CARTESIAN_POINT('Ctrl Pts',(2.44283775848,-36.3857400536,-1.27587644097));
#66308=CARTESIAN_POINT('Ctrl Pts',(2.42146674659,-36.4799878332,-1.2453487048));
#66309=CARTESIAN_POINT('Ctrl Pts',(2.42146674659,-36.5742356128,-1.2453487048));
#66310=CARTESIAN_POINT('Ctrl Pts',(2.05156482251,-36.2742356128,-1.81763077189));
#66311=CARTESIAN_POINT('Ctrl Pts',(2.0106619921,-36.2742356128,-1.73209067968));
#66312=CARTESIAN_POINT('Ctrl Pts',(1.96975916169,-36.3112466293,-1.64655058747));
#66313=CARTESIAN_POINT('Ctrl Pts',(1.93742957283,-36.3857400536,-1.57893971761));
#66314=CARTESIAN_POINT('Ctrl Pts',(1.92136706958,-36.4799878332,-1.54534820173));
#66315=CARTESIAN_POINT('Ctrl Pts',(1.92136706958,-36.5742356128,-1.54534820173));
#66316=CARTESIAN_POINT('Ctrl Pts',(1.46621585586,-36.2742356128,-2.03976910007));
#66317=CARTESIAN_POINT('Ctrl Pts',(1.43612509201,-36.2742356128,-1.95024888238));
#66318=CARTESIAN_POINT('Ctrl Pts',(1.40603432816,-36.3112466293,-1.86072866468));
#66319=CARTESIAN_POINT('Ctrl Pts',(1.38225059583,-36.3857400536,-1.78997190419));
#66320=CARTESIAN_POINT('Ctrl Pts',(1.37043397969,-36.4799878332,-1.75481739701));
#66321=CARTESIAN_POINT('Ctrl Pts',(1.37043397969,-36.5742356128,-1.75481739701));
#66322=CARTESIAN_POINT('Ctrl Pts',(1.20096079265,-36.2742356128,-2.12158773605));
#66323=CARTESIAN_POINT('Ctrl Pts',(1.17485210137,-36.2742356128,-2.03091619783));
#66324=CARTESIAN_POINT('Ctrl Pts',(1.14874341008,-36.3112466293,-1.9402446596));
#66325=CARTESIAN_POINT('Ctrl Pts',(1.1281071041,-36.3857400536,-1.86857789613));
#66326=CARTESIAN_POINT('Ctrl Pts',(1.11785424713,-36.4799878332,-1.83297126593));
#66327=CARTESIAN_POINT('Ctrl Pts',(1.11785424713,-36.5742356128,-1.83297126593));
#66328=CARTESIAN_POINT('Ctrl Pts',(0.933912767205,-36.2742356128,-2.18966247475));
#66329=CARTESIAN_POINT('Ctrl Pts',(0.911433093068,-36.2742356128,-2.09806650676));
#66330=CARTESIAN_POINT('Ctrl Pts',(0.888953418932,-36.3112466293,-2.00647053877));
#66331=CARTESIAN_POINT('Ctrl Pts',(0.871185490918,-36.3857400536,-1.93407310555));
#66332=CARTESIAN_POINT('Ctrl Pts',(0.862357742047,-36.4799878332,-1.89810345328));
#66333=CARTESIAN_POINT('Ctrl Pts',(0.862357742047,-36.5742356128,-1.89810345328));
#66334=CARTESIAN_POINT('Ctrl Pts',(0.665819006916,-36.2742356128,-2.24488956153));
#66335=CARTESIAN_POINT('Ctrl Pts',(0.646803823438,-36.2742356128,-2.1525799373));
#66336=CARTESIAN_POINT('Ctrl Pts',(0.62778863996,-36.3112466293,-2.06027031307));
#66337=CARTESIAN_POINT('Ctrl Pts',(0.61275904312,-36.3857400536,-1.98730880637));
#66338=CARTESIAN_POINT('Ctrl Pts',(0.60529179803,-36.4799878332,-1.9510589017));
#66339=CARTESIAN_POINT('Ctrl Pts',(0.60529179803,-36.5742356128,-1.9510589017));
#66340=CARTESIAN_POINT('',(0.605290655172242,-36.5742356128,-1.95105912937464));
#66341=CARTESIAN_POINT('Origin',(0.665390956717112,-36.5721143394352,-2.24281192044095));
#66342=CARTESIAN_POINT('Ctrl Pts',(4.39146896866,-36.5742356128,1.85520291202));
#66343=CARTESIAN_POINT('Ctrl Pts',(4.37092196604576,-36.5742356128,1.78912657731079));
#66344=CARTESIAN_POINT('Ctrl Pts',(4.34954081826218,-36.5742356128,1.72337655738574));
#66345=CARTESIAN_POINT('Ctrl Pts',(4.32735621433135,-36.5742356128,1.65805460794794));
#66346=CARTESIAN_POINT('Ctrl Pts',(4.30394651649965,-36.5742356128,1.58912540358241));
#66347=CARTESIAN_POINT('Ctrl Pts',(4.27964214656061,-36.5742356128,1.52067245888467));
#66348=CARTESIAN_POINT('Ctrl Pts',(4.25446325957601,-36.5742356128,1.45275525337923));
#66349=CARTESIAN_POINT('Ctrl Pts',(4.22739691464107,-36.5742356128,1.37974684310469));
#66350=CARTESIAN_POINT('Ctrl Pts',(4.19931999946701,-36.5742356128,1.30735692636008));
#66351=CARTESIAN_POINT('Ctrl Pts',(4.17024000686726,-36.5742356128,1.23559918194585));
#66352=CARTESIAN_POINT('Ctrl Pts',(4.14145877587494,-36.5742356128,1.16457866120843));
#66353=CARTESIAN_POINT('Ctrl Pts',(4.11169470089405,-36.5742356128,1.09417596395447));
#66354=CARTESIAN_POINT('Ctrl Pts',(4.08094114779705,-36.5742356128,1.02436413798126));
#66355=CARTESIAN_POINT('Ctrl Pts',(4.05224188440922,-36.5742356128,0.959215633843538));
#66356=CARTESIAN_POINT('Ctrl Pts',(4.02268063301999,-36.5742356128,0.894580469895503));
#66357=CARTESIAN_POINT('Ctrl Pts',(3.99224395132627,-36.5742356128,0.830420695088611));
#66358=CARTESIAN_POINT('Ctrl Pts',(3.97438465138359,-36.5742356128,0.792773731005568));
#66359=CARTESIAN_POINT('Ctrl Pts',(3.95622027870181,-36.5742356128,0.755282652752562));
#66360=CARTESIAN_POINT('Ctrl Pts',(3.9377422209914,-36.5742356128,0.717930475626564));
#66361=CARTESIAN_POINT('Ctrl Pts',(3.89734005075921,-36.5742356128,0.6362601484505));
#66362=CARTESIAN_POINT('Ctrl Pts',(3.8554424832124,-36.5742356128,0.555257996223974));
#66363=CARTESIAN_POINT('Ctrl Pts',(3.81197125901739,-36.5742356128,0.474816458033809));
#66364=CARTESIAN_POINT('Ctrl Pts',(3.80028137999852,-36.5742356128,0.453184864561387));
#66365=CARTESIAN_POINT('Ctrl Pts',(3.78847763386018,-36.5742356128,0.43159407411124));
#66366=CARTESIAN_POINT('Ctrl Pts',(3.77655836304664,-36.5742356128,0.410042706612038));
#66367=CARTESIAN_POINT('Ctrl Pts',(3.74584468184793,-36.5742356128,0.354508954495743));
#66368=CARTESIAN_POINT('Ctrl Pts',(3.71436491605534,-36.5742356128,0.299232780038763));
#66369=CARTESIAN_POINT('Ctrl Pts',(3.68208980817337,-36.5742356128,0.244210156230315));
#66370=CARTESIAN_POINT('Ctrl Pts',(3.64900348421455,-36.5742356128,0.187804570754112));
#66371=CARTESIAN_POINT('Ctrl Pts',(3.61508141465514,-36.5742356128,0.131665655865529));
#66372=CARTESIAN_POINT('Ctrl Pts',(3.58027857454058,-36.5742356128,0.0758427834194556));
#66373=CARTESIAN_POINT('Ctrl Pts',(3.54514722605774,-36.5742356128,0.0194929918863461));
#66374=CARTESIAN_POINT('Ctrl Pts',(3.50911845896627,-36.5742356128,-0.0365343947094508));
#66375=CARTESIAN_POINT('Ctrl Pts',(3.47213137149065,-36.5742356128,-0.0921391827048448));
#66376=CARTESIAN_POINT('Ctrl Pts',(3.43827624511192,-36.5742356128,-0.143035515812656));
#66377=CARTESIAN_POINT('Ctrl Pts',(3.40361565818781,-36.5742356128,-0.193580240571943));
#66378=CARTESIAN_POINT('Ctrl Pts',(3.3681038842297,-36.5742356128,-0.243648133987124));
#66379=CARTESIAN_POINT('Ctrl Pts',(3.32237639859336,-36.5742356128,-0.308119114222706));
#66380=CARTESIAN_POINT('Ctrl Pts',(3.27523990322948,-36.5742356128,-0.371798238816327));
#66381=CARTESIAN_POINT('Ctrl Pts',(3.22658364237517,-36.5742356128,-0.434351343972338));
#66382=CARTESIAN_POINT('Ctrl Pts',(3.1891805104024,-36.5742356128,-0.482437284124252));
#66383=CARTESIAN_POINT('Ctrl Pts',(3.15087884016424,-36.5742356128,-0.529856326762846));
#66384=CARTESIAN_POINT('Ctrl Pts',(3.11161932172789,-36.5742356128,-0.576438135300435));
#66385=CARTESIAN_POINT('Ctrl Pts',(3.07634816132177,-36.5742356128,-0.618287717424055));
#66386=CARTESIAN_POINT('Ctrl Pts',(3.04030401646786,-36.5742356128,-0.659457592247737));
#66387=CARTESIAN_POINT('Ctrl Pts',(3.00347671654498,-36.5742356128,-0.699843781432812));
#66388=CARTESIAN_POINT('Ctrl Pts',(2.95584798283857,-36.5742356128,-0.752075225338318));
#66389=CARTESIAN_POINT('Ctrl Pts',(2.90690574095255,-36.5742356128,-0.802997650979128));
#66390=CARTESIAN_POINT('Ctrl Pts',(2.85663353129263,-36.5742356128,-0.852444677426488));
#66391=CARTESIAN_POINT('Ctrl Pts',(2.80616628734769,-36.5742356128,-0.902083536807286));
#66392=CARTESIAN_POINT('Ctrl Pts',(2.75435852744095,-36.5742356128,-0.950235664741411));
#66393=CARTESIAN_POINT('Ctrl Pts',(2.70121735198846,-36.5742356128,-0.996779778325614));
#66394=CARTESIAN_POINT('Ctrl Pts',(2.64787457427578,-36.5742356128,-1.04350046682405));
#66395=CARTESIAN_POINT('Ctrl Pts',(2.59318803634864,-36.5742356128,-1.08860107508899));
#66396=CARTESIAN_POINT('Ctrl Pts',(2.5371919504335,-36.5742356128,-1.13200401281568));
#66397=CARTESIAN_POINT('Ctrl Pts',(2.48088732176473,-36.5742356128,-1.17564610407788));
#66398=CARTESIAN_POINT('Ctrl Pts',(2.42325845763622,-36.5742356128,-1.2175719302296));
#66399=CARTESIAN_POINT('Ctrl Pts',(2.36437063367713,-36.5742356128,-1.25774567927551));
#66400=CARTESIAN_POINT('Ctrl Pts',(2.30532530357416,-36.5742356128,-1.29802688028471));
#66401=CARTESIAN_POINT('Ctrl Pts',(2.24501407262125,-36.5742356128,-1.33654682218278));
#66402=CARTESIAN_POINT('Ctrl Pts',(2.18353641291566,-36.5742356128,-1.37330977651211));
#66403=CARTESIAN_POINT('Ctrl Pts',(2.1218304847959,-36.5742356128,-1.41020923280533));
#66404=CARTESIAN_POINT('Ctrl Pts',(2.05894925274633,-36.5742356128,-1.44533884235053));
#66405=CARTESIAN_POINT('Ctrl Pts',(1.99503015932727,-36.5742356128,-1.47874042189916));
#66406=CARTESIAN_POINT('Ctrl Pts',(1.94867287876171,-36.5742356128,-1.5029648955524));
#66407=CARTESIAN_POINT('Ctrl Pts',(1.90177045743172,-36.5742356128,-1.52628124306212));
#66408=CARTESIAN_POINT('Ctrl Pts',(1.85438824548848,-36.5742356128,-1.54871668750062));
#66409=CARTESIAN_POINT('Ctrl Pts',(1.80557874502425,-36.5742356128,-1.57182795206227));
#66410=CARTESIAN_POINT('Ctrl Pts',(1.75626193134941,-36.5742356128,-1.59400511597658));
#66411=CARTESIAN_POINT('Ctrl Pts',(1.70652627741759,-36.5742356128,-1.61529464396692));
#66412=CARTESIAN_POINT('Ctrl Pts',(1.6654769857331,-36.5742356128,-1.63286594292879));
#66413=CARTESIAN_POINT('Ctrl Pts',(1.62415059395768,-36.5742356128,-1.64982906877745));
#66414=CARTESIAN_POINT('Ctrl Pts',(1.58259075611606,-36.5742356128,-1.66621171622079));
#66415=CARTESIAN_POINT('Ctrl Pts',(1.50335243862315,-36.5742356128,-1.69744700218212));
#66416=CARTESIAN_POINT('Ctrl Pts',(1.4232675352806,-36.5742356128,-1.72657363957852));
#66417=CARTESIAN_POINT('Ctrl Pts',(1.34258681478873,-36.5742356128,-1.75377965505486));
#66418=CARTESIAN_POINT('Ctrl Pts',(1.26331159092117,-36.5742356128,-1.78051172876817));
#66419=CARTESIAN_POINT('Ctrl Pts',(1.18346058848082,-36.5742356128,-1.80539021068333));
#66420=CARTESIAN_POINT('Ctrl Pts',(1.1032221367378,-36.5742356128,-1.82857498991327));
#66421=CARTESIAN_POINT('Ctrl Pts',(1.02084982398067,-36.5742356128,-1.85237634505469));
#66422=CARTESIAN_POINT('Ctrl Pts',(0.938068982789468,-36.5742356128,-1.8743936397323));
#66423=CARTESIAN_POINT('Ctrl Pts',(0.85503576346161,-36.5742356128,-1.89476771454273));
#66424=CARTESIAN_POINT('Ctrl Pts',(0.772002544133753,-36.5742356128,-1.91514178935316));
#66425=CARTESIAN_POINT('Ctrl Pts',(0.688716543213015,-36.5742356128,-1.93387344834334));
#66426=CARTESIAN_POINT('Ctrl Pts',(0.60529179803,-36.5742356128,-1.9510589017));
#66427=CARTESIAN_POINT('Ctrl Pts',(0.605291698516,-37.9742356128,-1.9510589194));
#66428=CARTESIAN_POINT('Ctrl Pts',(0.605291702509,-38.0684833924,-1.9510589186));
#66429=CARTESIAN_POINT('Ctrl Pts',(0.612758907916,-38.162731172,-1.98730883125));
#66430=CARTESIAN_POINT('Ctrl Pts',(0.627788420004,-38.2372245963,-2.06027035501));
#66431=CARTESIAN_POINT('Ctrl Pts',(0.64680349383,-38.2742356128,-2.15258000132));
#66432=CARTESIAN_POINT('Ctrl Pts',(0.665818566089,-38.2742356128,-2.24488964795));
#66433=CARTESIAN_POINT('Ctrl Pts',(0.919213880749,-37.9742356128,-1.88639136854));
#66434=CARTESIAN_POINT('Ctrl Pts',(0.919213677207,-38.0684833929,-1.88639140934));
#66435=CARTESIAN_POINT('Ctrl Pts',(0.928343625497,-38.162731173,-1.9222988207));
#66436=CARTESIAN_POINT('Ctrl Pts',(0.946720057801,-38.2372245974,-1.99457092792));
#66437=CARTESIAN_POINT('Ctrl Pts',(0.969969721523,-38.2742356135,-2.0860083113));
#66438=CARTESIAN_POINT('Ctrl Pts',(0.993219464992,-38.2742356128,-2.17744567841));
#66439=CARTESIAN_POINT('Ctrl Pts',(1.23048109925,-37.9742356128,-1.80341900309));
#66440=CARTESIAN_POINT('Ctrl Pts',(1.23048134587,-38.0684833489,-1.8034189616));
#66441=CARTESIAN_POINT('Ctrl Pts',(1.24137540827,-38.162731085,-1.83884940092));
#66442=CARTESIAN_POINT('Ctrl Pts',(1.26330197813,-38.2372244937,-1.91016159119));
#66443=CARTESIAN_POINT('Ctrl Pts',(1.29104294839,-38.2742355444,-2.00038457075));
#66444=CARTESIAN_POINT('Ctrl Pts',(1.31878382917,-38.2742356128,-2.09060759247));
#66445=CARTESIAN_POINT('Ctrl Pts',(1.53827172349,-37.9742356128,-1.70133851312));
#66446=CARTESIAN_POINT('Ctrl Pts',(1.53827165445,-38.0684833944,-1.70133852637));
#66447=CARTESIAN_POINT('Ctrl Pts',(1.55116199328,-38.1627311759,-1.73618774441));
#66448=CARTESIAN_POINT('Ctrl Pts',(1.577106932,-38.2372246008,-1.80633002242));
#66449=CARTESIAN_POINT('Ctrl Pts',(1.60993205855,-38.2742356158,-1.8950727983));
#66450=CARTESIAN_POINT('Ctrl Pts',(1.64275721303,-38.2742356128,-1.98381556726));
#66451=CARTESIAN_POINT('Ctrl Pts',(2.08916968394,-37.9742356128,-1.4617720322));
#66452=CARTESIAN_POINT('Ctrl Pts',(2.08916974353,-38.0684833908,-1.46177202076));
#66453=CARTESIAN_POINT('Ctrl Pts',(2.10696029946,-38.1627311688,-1.49456736992));
#66454=CARTESIAN_POINT('Ctrl Pts',(2.14276792726,-38.2372245925,-1.56057578049));
#66455=CARTESIAN_POINT('Ctrl Pts',(2.18807107629,-38.2742356103,-1.64408847689));
#66456=CARTESIAN_POINT('Ctrl Pts',(2.23337420121,-38.2742356128,-1.72760117925));
#66457=CARTESIAN_POINT('Ctrl Pts',(2.57507298908,-37.9742356128,-1.12324782371));
#66458=CARTESIAN_POINT('Ctrl Pts',(2.57507293765,-38.0684833939,-1.12324783358));
#66459=CARTESIAN_POINT('Ctrl Pts',(2.5981428301,-38.1627311749,-1.15242255957));
#66460=CARTESIAN_POINT('Ctrl Pts',(2.64457651027,-38.2372245997,-1.21114358345));
#66461=CARTESIAN_POINT('Ctrl Pts',(2.7033236223,-38.2742356151,-1.28543639078));
#66462=CARTESIAN_POINT('Ctrl Pts',(2.76207075515,-38.2742356128,-1.35972919295));
#66463=CARTESIAN_POINT('Ctrl Pts',(2.7836528701,-37.9742356128,-0.943576895053));
#66464=CARTESIAN_POINT('Ctrl Pts',(2.78365286427,-38.0684833991,-0.943576903287));
#66465=CARTESIAN_POINT('Ctrl Pts',(2.80899055527,-38.1627311853,-0.970778224792));
#66466=CARTESIAN_POINT('Ctrl Pts',(2.85998865839,-38.237224612,-1.02552730908));
#66467=CARTESIAN_POINT('Ctrl Pts',(2.92451056942,-38.2742356233,-1.09479488721));
#66468=CARTESIAN_POINT('Ctrl Pts',(2.98903247965,-38.2742356128,-1.16406245943));
#66469=CARTESIAN_POINT('Ctrl Pts',(3.16286118659,-37.9742356128,-0.547454755393));
#66470=CARTESIAN_POINT('Ctrl Pts',(3.16286119234,-38.0684833859,-0.547454747271));
#66471=CARTESIAN_POINT('Ctrl Pts',(3.19188224207,-38.162731159,-0.57069685876));
#66472=CARTESIAN_POINT('Ctrl Pts',(3.25029396105,-38.2372245809,-0.617477115127));
#66473=CARTESIAN_POINT('Ctrl Pts',(3.32419544657,-38.2742356026,-0.676662685237));
#66474=CARTESIAN_POINT('Ctrl Pts',(3.39809693287,-38.2742356128,-0.735848261173));
#66475=CARTESIAN_POINT('Ctrl Pts',(3.48018648031,-37.9742356128,-0.0953176293782));
#66476=CARTESIAN_POINT('Ctrl Pts',(3.48018647464,-38.0684833989,-0.0953176373891));
#66477=CARTESIAN_POINT('Ctrl Pts',(3.51119197157,-38.162731185,-0.115616438491));
#66478=CARTESIAN_POINT('Ctrl Pts',(3.57359787491,-38.2372246116,-0.156472565458));
#66479=CARTESIAN_POINT('Ctrl Pts',(3.65255273532,-38.274235623,-0.208163017913));
#66480=CARTESIAN_POINT('Ctrl Pts',(3.73150759497,-38.2742356128,-0.25985346462));
#66481=CARTESIAN_POINT('Ctrl Pts',(3.62537652215,-37.9742356128,0.135235517809));
#66482=CARTESIAN_POINT('Ctrl Pts',(3.62537652521,-38.0684833915,0.135235523567));
#66483=CARTESIAN_POINT('Ctrl Pts',(3.65702258613,-38.1627311701,0.115978596807));
#66484=CARTESIAN_POINT('Ctrl Pts',(3.72071777861,-38.237224594,0.0772195150144));
#66485=CARTESIAN_POINT('Ctrl Pts',(3.80130381638,-38.2742356113,0.0281821786018));
#66486=CARTESIAN_POINT('Ctrl Pts',(3.88188985347,-38.2742356128,-0.0208551603171));
#66487=CARTESIAN_POINT('Ctrl Pts',(3.89322431128,-37.9742356128,0.603415611262));
#66488=CARTESIAN_POINT('Ctrl Pts',(3.89322430822,-38.0684833934,0.603415605503));
#66489=CARTESIAN_POINT('Ctrl Pts',(3.92618569708,-38.162731174,0.586451536215));
#66490=CARTESIAN_POINT('Ctrl Pts',(3.9925282778,-38.2372245987,0.552307296845));
#66491=CARTESIAN_POINT('Ctrl Pts',(4.07646375994,-38.2742356144,0.509108624308));
#66492=CARTESIAN_POINT('Ctrl Pts',(4.16039924278,-38.2742356128,0.465909954278));
#66493=CARTESIAN_POINT('Ctrl Pts',(4.11688435895,-37.9742356128,1.08932953896));
#66494=CARTESIAN_POINT('Ctrl Pts',(4.116884362,-38.0684833915,1.08932954472));
#66495=CARTESIAN_POINT('Ctrl Pts',(4.15092281005,-38.1627311701,1.0747166191));
#66496=CARTESIAN_POINT('Ctrl Pts',(4.21943324733,-38.237224594,1.04530468777));
#66497=CARTESIAN_POINT('Ctrl Pts',(4.3061114488,-38.2742356113,1.00809320298));
#66498=CARTESIAN_POINT('Ctrl Pts',(4.39278964957,-38.2742356128,0.970881715692));
#66499=CARTESIAN_POINT('Ctrl Pts',(4.21879577195,-37.9742356128,1.33879606859));
#66500=CARTESIAN_POINT('Ctrl Pts',(4.21879576946,-38.0684833923,1.33879606025));
#66501=CARTESIAN_POINT('Ctrl Pts',(4.25334110804,-38.1627311718,1.32542139016));
#66502=CARTESIAN_POINT('Ctrl Pts',(4.32287172004,-38.237224596,1.29850153552));
#66503=CARTESIAN_POINT('Ctrl Pts',(4.4108406614,-38.2742356126,1.26444308661));
#66504=CARTESIAN_POINT('Ctrl Pts',(4.49880960361,-38.2742356128,1.23038464024));
#66505=CARTESIAN_POINT('Ctrl Pts',(4.31054313212,-37.9742356128,1.59495655094));
#66506=CARTESIAN_POINT('Ctrl Pts',(4.31054313212,-38.0684833924,1.59495655094));
#66507=CARTESIAN_POINT('Ctrl Pts',(4.34551178853,-38.1627311721,1.58276691751));
#66508=CARTESIAN_POINT('Ctrl Pts',(4.41589451694,-38.2372245963,1.55823251586));
#66509=CARTESIAN_POINT('Ctrl Pts',(4.50494150016,-38.2742356128,1.52719196862));
#66510=CARTESIAN_POINT('Ctrl Pts',(4.59398848352,-38.2742356128,1.49615142185));
#66511=CARTESIAN_POINT('Ctrl Pts',(4.39146896866,-37.9742356128,1.85520291202));
#66512=CARTESIAN_POINT('Ctrl Pts',(4.39146896866,-38.0684833924,1.85520291202));
#66513=CARTESIAN_POINT('Ctrl Pts',(4.42681071743,-38.1627311721,1.84421309233));
#66514=CARTESIAN_POINT('Ctrl Pts',(4.49794434558,-38.2372245963,1.82209348097));
#66515=CARTESIAN_POINT('Ctrl Pts',(4.5879413698,-38.2742356128,1.79410813493));
#66516=CARTESIAN_POINT('Ctrl Pts',(4.67793839402,-38.2742356128,1.76612278889));
#66517=CARTESIAN_POINT('',(0.605290084208,-37.9742356128,-1.95105924441));
#66518=CARTESIAN_POINT('Ctrl Pts',(4.39146896866,-37.9742356128,1.85520291202));
#66519=CARTESIAN_POINT('Ctrl Pts',(4.32479970425,-37.9742356128,1.64080372629));
#66520=CARTESIAN_POINT('Ctrl Pts',(4.25081929042,-37.9742356128,1.42932711758));
#66521=CARTESIAN_POINT('Ctrl Pts',(4.17005920267,-37.9742356128,1.2223938778));
#66522=CARTESIAN_POINT('Ctrl Pts',(3.99422837986,-37.9742356128,0.815818314863));
#66523=CARTESIAN_POINT('Ctrl Pts',(3.78982855046,-37.9742356128,0.424030803924));
#66524=CARTESIAN_POINT('Ctrl Pts',(3.67898467854,-37.9742356128,0.229105997103));
#66525=CARTESIAN_POINT('Ctrl Pts',(3.50079208815,-37.9742356128,-0.0598766153727));
#66526=CARTESIAN_POINT('Ctrl Pts',(3.3007785305,-37.9742356128,-0.339537614852));
#66527=CARTESIAN_POINT('Ctrl Pts',(3.23140437767,-37.9742356128,-0.431505525867));
#66528=CARTESIAN_POINT('Ctrl Pts',(2.94231272615,-37.9742356128,-0.791436832827));
#66529=CARTESIAN_POINT('Ctrl Pts',(2.60717935657,-37.9742356128,-1.11036965749));
#66530=CARTESIAN_POINT('Ctrl Pts',(2.32835178279,-37.9742356128,-1.31285318023));
#66531=CARTESIAN_POINT('Ctrl Pts',(1.82071765691,-37.9742356128,-1.59091161501));
#66532=CARTESIAN_POINT('Ctrl Pts',(1.27370365618,-37.9742356128,-1.78402347955));
#66533=CARTESIAN_POINT('Ctrl Pts',(1.05241756576,-37.9742356128,-1.84948999718));
#66534=CARTESIAN_POINT('Ctrl Pts',(0.829282811325,-37.9742356128,-1.90491676645));
#66535=CARTESIAN_POINT('Ctrl Pts',(0.605290084208,-37.9742356128,-1.95105924441));
#66536=CARTESIAN_POINT('Origin',(0.66539024333551,-37.9763568939093,-2.24281205713374));
#66537=CARTESIAN_POINT('Ctrl Pts',(4.39146896866,-37.9742356128,1.85520291202));
#66538=CARTESIAN_POINT('Ctrl Pts',(4.39146896866,-36.2942356128,1.85520291202));
#66539=CARTESIAN_POINT('Ctrl Pts',(4.32479970425,-37.9742356128,1.64080372629));
#66540=CARTESIAN_POINT('Ctrl Pts',(4.32479970425,-36.2942356128,1.64080372629));
#66541=CARTESIAN_POINT('Ctrl Pts',(4.25081929042,-37.9742356128,1.42932711758));
#66542=CARTESIAN_POINT('Ctrl Pts',(4.25081929042,-36.2942356128,1.42932711758));
#66543=CARTESIAN_POINT('Ctrl Pts',(4.17005920267,-37.9742356128,1.2223938778));
#66544=CARTESIAN_POINT('Ctrl Pts',(4.17005920267,-36.2942356128,1.2223938778));
#66545=CARTESIAN_POINT('Ctrl Pts',(3.99422837986,-37.9742356128,0.815818314863));
#66546=CARTESIAN_POINT('Ctrl Pts',(3.99422837986,-36.2942356128,0.815818314863));
#66547=CARTESIAN_POINT('Ctrl Pts',(3.78982855046,-37.9742356128,0.424030803924));
#66548=CARTESIAN_POINT('Ctrl Pts',(3.78982855046,-36.2942356128,0.424030803924));
#66549=CARTESIAN_POINT('Ctrl Pts',(3.67898467854,-37.9742356128,0.229105997103));
#66550=CARTESIAN_POINT('Ctrl Pts',(3.67898467854,-36.2942356128,0.229105997103));
#66551=CARTESIAN_POINT('Ctrl Pts',(3.50079208815,-37.9742356128,-0.0598766153727));
#66552=CARTESIAN_POINT('Ctrl Pts',(3.50079208815,-36.2942356128,-0.0598766153727));
#66553=CARTESIAN_POINT('Ctrl Pts',(3.3007785305,-37.9742356128,-0.339537614852));
#66554=CARTESIAN_POINT('Ctrl Pts',(3.3007785305,-36.2942356128,-0.339537614852));
#66555=CARTESIAN_POINT('Ctrl Pts',(3.23140437767,-37.9742356128,-0.431505525867));
#66556=CARTESIAN_POINT('Ctrl Pts',(3.23140437767,-36.2942356128,-0.431505525867));
#66557=CARTESIAN_POINT('Ctrl Pts',(2.94231272615,-37.9742356128,-0.791436832827));
#66558=CARTESIAN_POINT('Ctrl Pts',(2.94231272615,-36.2942356128,-0.791436832827));
#66559=CARTESIAN_POINT('Ctrl Pts',(2.60717935657,-37.9742356128,-1.11036965749));
#66560=CARTESIAN_POINT('Ctrl Pts',(2.60717935657,-36.2942356128,-1.11036965749));
#66561=CARTESIAN_POINT('Ctrl Pts',(2.32835178279,-37.9742356128,-1.31285318023));
#66562=CARTESIAN_POINT('Ctrl Pts',(2.32835178279,-36.2942356128,-1.31285318023));
#66563=CARTESIAN_POINT('Ctrl Pts',(1.82071765691,-37.9742356128,-1.59091161501));
#66564=CARTESIAN_POINT('Ctrl Pts',(1.82071765691,-36.2942356128,-1.59091161501));
#66565=CARTESIAN_POINT('Ctrl Pts',(1.27370365618,-37.9742356128,-1.78402347955));
#66566=CARTESIAN_POINT('Ctrl Pts',(1.27370365618,-36.2942356128,-1.78402347955));
#66567=CARTESIAN_POINT('Ctrl Pts',(1.05241756576,-37.9742356128,-1.84948999718));
#66568=CARTESIAN_POINT('Ctrl Pts',(1.05241756576,-36.2942356128,-1.84948999718));
#66569=CARTESIAN_POINT('Ctrl Pts',(0.829282811325,-37.9742356128,-1.90491676645));
#66570=CARTESIAN_POINT('Ctrl Pts',(0.829282811325,-36.2942356128,-1.90491676645));
#66571=CARTESIAN_POINT('Ctrl Pts',(0.605290084208,-37.9742356128,-1.95105924441));
#66572=CARTESIAN_POINT('Ctrl Pts',(0.605290084208,-36.2942356128,-1.95105924441));
#66573=CARTESIAN_POINT('',(0.605290084208,-37.2742356128,-1.95105924441));
#66574=CARTESIAN_POINT('Ctrl Pts',(0.665819092629,-36.2742356128,-2.2448895341));
#66575=CARTESIAN_POINT('Ctrl Pts',(0.64680334381,-36.2742356128,-2.15258002616));
#66576=CARTESIAN_POINT('Ctrl Pts',(0.627787594992,-36.3112466293,-2.06027051821));
#66577=CARTESIAN_POINT('Ctrl Pts',(0.612757551307,-36.3857400536,-1.98730910342));
#66578=CARTESIAN_POINT('Ctrl Pts',(0.605290084208,-36.4799878332,-1.95105924441));
#66579=CARTESIAN_POINT('Ctrl Pts',(0.605290084208,-36.5742356128,-1.95105924441));
#66580=CARTESIAN_POINT('Ctrl Pts',(0.534429719062,-36.2742356128,-2.27195573108));
#66581=CARTESIAN_POINT('Ctrl Pts',(0.519212546478,-36.2742356128,-2.17886371683));
#66582=CARTESIAN_POINT('Ctrl Pts',(0.503995373894,-36.3112466293,-2.08577170258));
#66583=CARTESIAN_POINT('Ctrl Pts',(0.491967724046,-36.3857400536,-2.01219179502));
#66584=CARTESIAN_POINT('Ctrl Pts',(0.48599195433,-36.4799878332,-1.97563464648));
#66585=CARTESIAN_POINT('Ctrl Pts',(0.48599195433,-36.5742356128,-1.97563464648));
#66586=CARTESIAN_POINT('Ctrl Pts',(0.401708001693,-36.2742356128,-2.29225119574));
#66587=CARTESIAN_POINT('Ctrl Pts',(0.390294367497,-36.2742356128,-2.19857933068));
#66588=CARTESIAN_POINT('Ctrl Pts',(0.3788807333,-36.3112466293,-2.10490746561));
#66589=CARTESIAN_POINT('Ctrl Pts',(0.369859399314,-36.3857400536,-2.03086924402));
#66590=CARTESIAN_POINT('Ctrl Pts',(0.365377275672,-36.4799878332,-1.99408438867));
#66591=CARTESIAN_POINT('Ctrl Pts',(0.365377275672,-36.5742356128,-1.99408438867));
#66592=CARTESIAN_POINT('Ctrl Pts',(0.268094966815,-36.2742356128,-2.30577886056));
#66593=CARTESIAN_POINT('Ctrl Pts',(0.260489352365,-36.2742356128,-2.21172355227));
#66594=CARTESIAN_POINT('Ctrl Pts',(0.252883737915,-36.3112466293,-2.11766824397));
#66595=CARTESIAN_POINT('Ctrl Pts',(0.246872116974,-36.3857400536,-2.0433269187));
#66596=CARTESIAN_POINT('Ctrl Pts',(0.243885544115,-36.4799878332,-2.00639151578));
#66597=CARTESIAN_POINT('Ctrl Pts',(0.243885544115,-36.5742356128,-2.00639151578));
#66598=CARTESIAN_POINT('Ctrl Pts',(5.76690590749E-6,-36.2742356128,-2.31931022318));
#66599=CARTESIAN_POINT('Ctrl Pts',(1.95516921384E-6,-36.2742356128,-2.2248691397));
#66600=CARTESIAN_POINT('Ctrl Pts',(-1.85656748074E-6,-36.3112466293,-2.13042805622));
#66601=CARTESIAN_POINT('Ctrl Pts',(-4.72441517072E-6,-36.3857400536,-2.05578187487));
#66602=CARTESIAN_POINT('Ctrl Pts',(-6.36622882408E-6,-36.4799878332,-2.01869491784));
#66603=CARTESIAN_POINT('Ctrl Pts',(-6.36622882421E-6,-36.5742356128,-2.01869491784));
#66604=CARTESIAN_POINT('Ctrl Pts',(-0.268106045432,-36.2742356128,-2.30577884111));
#66605=CARTESIAN_POINT('Ctrl Pts',(-0.260493021619,-36.2742356128,-2.21172353811));
#66606=CARTESIAN_POINT('Ctrl Pts',(-0.252879997805,-36.3112466293,-2.11766823512));
#66607=CARTESIAN_POINT('Ctrl Pts',(-0.246862810402,-36.3857400536,-2.04332691403));
#66608=CARTESIAN_POINT('Ctrl Pts',(-0.243873037996,-36.4799878332,-2.00639151319));
#66609=CARTESIAN_POINT('Ctrl Pts',(-0.243873037996,-36.5742356128,-2.00639151319));
#66610=CARTESIAN_POINT('Ctrl Pts',(-0.401685240587,-36.2742356128,-2.29225613481));
#66611=CARTESIAN_POINT('Ctrl Pts',(-0.390286664018,-36.2742356128,-2.19858115746));
#66612=CARTESIAN_POINT('Ctrl Pts',(-0.378888087449,-36.3112466293,-2.10490618011));
#66613=CARTESIAN_POINT('Ctrl Pts',(-0.369878075217,-36.3857400536,-2.03086561975));
#66614=CARTESIAN_POINT('Ctrl Pts',(-0.365402444484,-36.4799878332,-1.99407942103));
#66615=CARTESIAN_POINT('Ctrl Pts',(-0.365402444484,-36.5742356128,-1.99407942103));
#66616=CARTESIAN_POINT('Ctrl Pts',(-0.53444473621,-36.2742356128,-2.27195243343));
#66617=CARTESIAN_POINT('Ctrl Pts',(-0.519217514301,-36.2742356128,-2.17886250595));
#66618=CARTESIAN_POINT('Ctrl Pts',(-0.503990292391,-36.3112466293,-2.08577257847));
#66619=CARTESIAN_POINT('Ctrl Pts',(-0.491955086087,-36.3857400536,-2.0121942395));
#66620=CARTESIAN_POINT('Ctrl Pts',(-0.485974983482,-36.4799878332,-1.97563799122));
#66621=CARTESIAN_POINT('Ctrl Pts',(-0.485974983482,-36.5742356128,-1.97563799122));
#66622=CARTESIAN_POINT('Ctrl Pts',(-0.665818883669,-36.2742356128,-2.24488957828));
#66623=CARTESIAN_POINT('Ctrl Pts',(-0.646803200563,-36.2742356128,-2.1525800567));
#66624=CARTESIAN_POINT('Ctrl Pts',(-0.627787517457,-36.3112466293,-2.06027053512));
#66625=CARTESIAN_POINT('Ctrl Pts',(-0.612757525711,-36.3857400536,-1.98730910956));
#66626=CARTESIAN_POINT('Ctrl Pts',(-0.605290084417,-36.4799878332,-1.9510592452));
#66627=CARTESIAN_POINT('Ctrl Pts',(-0.605290084417,-36.5742356128,-1.9510592452));
#66628=CARTESIAN_POINT('',(-0.605290084208,-36.5742356128,-1.95105924441));
#66629=CARTESIAN_POINT('Origin',(-0.665390756021192,-36.5721143232865,-2.24281194064002));
#66630=CARTESIAN_POINT('Origin',(3.40005801291454E-15,-36.5742356128,0.240847787955639));
#66631=CARTESIAN_POINT('Ctrl Pts',(-0.605290082239,-37.9742356128,-1.95105923702));
#66632=CARTESIAN_POINT('Ctrl Pts',(-0.605290082237,-38.0684833924,-1.95105923702));
#66633=CARTESIAN_POINT('Ctrl Pts',(-0.612757635964,-38.1627311719,-1.98730907779));
#66634=CARTESIAN_POINT('Ctrl Pts',(-0.627787854008,-38.2372245962,-2.06027045589));
#66635=CARTESIAN_POINT('Ctrl Pts',(-0.646803823428,-38.2742356128,-2.15257991743));
#66636=CARTESIAN_POINT('Ctrl Pts',(-0.665819792855,-38.2742356128,-2.24488937901));
#66637=CARTESIAN_POINT('Ctrl Pts',(-0.485962182438,-37.9742356128,-1.97564071896));
#66638=CARTESIAN_POINT('Ctrl Pts',(-0.485962182542,-38.0684833923,-1.97564071893));
#66639=CARTESIAN_POINT('Ctrl Pts',(-0.491944923867,-38.1627311718,-2.0121964271));
#66640=CARTESIAN_POINT('Ctrl Pts',(-0.503985876403,-38.237224596,-2.08577358875));
#66641=CARTESIAN_POINT('Ctrl Pts',(-0.519220185478,-38.2742356126,-2.17886206466));
#66642=CARTESIAN_POINT('Ctrl Pts',(-0.534454494532,-38.2742356128,-2.27195054066));
#66643=CARTESIAN_POINT('Ctrl Pts',(-0.365419065041,-37.9742356128,-1.99407581982));
#66644=CARTESIAN_POINT('Ctrl Pts',(-0.365419081723,-38.0684833948,-1.99407581622));
#66645=CARTESIAN_POINT('Ctrl Pts',(-0.369890629768,-38.1627311768,-2.03086284972));
#66646=CARTESIAN_POINT('Ctrl Pts',(-0.378891751271,-38.2372246019,-2.10490523008));
#66647=CARTESIAN_POINT('Ctrl Pts',(-0.390279343346,-38.2742356166,-2.19858245447));
#66648=CARTESIAN_POINT('Ctrl Pts',(-0.40166692858,-38.2742356128,-2.29225967882));
#66649=CARTESIAN_POINT('Ctrl Pts',(-0.243866233741,-37.9742356128,-2.0063927176));
#66650=CARTESIAN_POINT('Ctrl Pts',(-0.24386627647,-38.0684833946,-2.00639271368));
#66651=CARTESIAN_POINT('Ctrl Pts',(-0.246856907969,-38.1627311764,-2.04332784119));
#66652=CARTESIAN_POINT('Ctrl Pts',(-0.252876527386,-38.2372246015,-2.11766870518));
#66653=CARTESIAN_POINT('Ctrl Pts',(-0.260492285044,-38.2742356162,-2.21172339427));
#66654=CARTESIAN_POINT('Ctrl Pts',(-0.268108025841,-38.2742356128,-2.3057780836));
#66655=CARTESIAN_POINT('Ctrl Pts',(-9.79524459687E-6,-37.9742356128,-2.01869408534));
#66656=CARTESIAN_POINT('Ctrl Pts',(-9.85391250738E-6,-38.0684833926,-2.01869408524));
#66657=CARTESIAN_POINT('Ctrl Pts',(-7.45742464767E-6,-38.1627311723,-2.05578125539));
#66658=CARTESIAN_POINT('Ctrl Pts',(-2.24378715802E-6,-38.2372245966,-2.1304277776));
#66659=CARTESIAN_POINT('Ctrl Pts',(4.25428334891E-6,-38.2742356131,-2.22486932944));
#66660=CARTESIAN_POINT('Ctrl Pts',(1.07753114626E-5,-38.2742356128,-2.31931088122));
#66661=CARTESIAN_POINT('Ctrl Pts',(0.24388974966,-37.9742356128,-2.00639262475));
#66662=CARTESIAN_POINT('Ctrl Pts',(0.243889710559,-38.06848339,-2.00639262888));
#66663=CARTESIAN_POINT('Ctrl Pts',(0.246875395247,-38.1627311672,-2.04332774367));
#66664=CARTESIAN_POINT('Ctrl Pts',(0.252884521209,-38.2372245906,-2.11766857213));
#66665=CARTESIAN_POINT('Ctrl Pts',(0.26048731995,-38.274235609,-2.21172321325));
#66666=CARTESIAN_POINT('Ctrl Pts',(0.268090134128,-38.2742356128,-2.30577785428));
#66667=CARTESIAN_POINT('Ctrl Pts',(0.365375386943,-37.9742356128,-1.99408468454));
#66668=CARTESIAN_POINT('Ctrl Pts',(0.365375378581,-38.0684833912,-1.99408468674));
#66669=CARTESIAN_POINT('Ctrl Pts',(0.369856652983,-38.1627311695,-2.03086969573));
#66670=CARTESIAN_POINT('Ctrl Pts',(0.378878655381,-38.2372245932,-2.10490773566));
#66671=CARTESIAN_POINT('Ctrl Pts',(0.390292146263,-38.2742356108,-2.19857957522));
#66672=CARTESIAN_POINT('Ctrl Pts',(0.401705640577,-38.2742356128,-2.29225141461));
#66673=CARTESIAN_POINT('Ctrl Pts',(0.485990680767,-37.9742356128,-1.97563490883));
#66674=CARTESIAN_POINT('Ctrl Pts',(0.485990680767,-38.0684833924,-1.97563490883));
#66675=CARTESIAN_POINT('Ctrl Pts',(0.491966958449,-38.1627311721,-2.01219195263));
#66676=CARTESIAN_POINT('Ctrl Pts',(0.50399405237,-38.2372245964,-2.08577197488));
#66677=CARTESIAN_POINT('Ctrl Pts',(0.519211184386,-38.2742356128,-2.17886399742));
#66678=CARTESIAN_POINT('Ctrl Pts',(0.534428316418,-38.2742356128,-2.27195602003));
#66679=CARTESIAN_POINT('Ctrl Pts',(0.605290084208,-37.9742356128,-1.95105924441));
#66680=CARTESIAN_POINT('Ctrl Pts',(0.605290084208,-38.0684833924,-1.95105924441));
#66681=CARTESIAN_POINT('Ctrl Pts',(0.612757551307,-38.1627311721,-1.98730910342));
#66682=CARTESIAN_POINT('Ctrl Pts',(0.627787594992,-38.2372245963,-2.06027051821));
#66683=CARTESIAN_POINT('Ctrl Pts',(0.64680334381,-38.2742356128,-2.15258002616));
#66684=CARTESIAN_POINT('Ctrl Pts',(0.665819092629,-38.2742356128,-2.2448895341));
#66685=CARTESIAN_POINT('',(-0.605290084208,-37.9742356128,-1.95105924441));
#66686=CARTESIAN_POINT('Origin',(0.,-37.9742356128,0.240847787949066));
#66687=CARTESIAN_POINT('Origin',(-0.665392224177974,-37.9763569242406,-2.24281160936468));
#66688=CARTESIAN_POINT('Ctrl Pts',(0.605290084208,-37.9742356128,-1.95105924441));
#66689=CARTESIAN_POINT('Ctrl Pts',(0.605290084208,-36.2942356128,-1.95105924441));
#66690=CARTESIAN_POINT('Ctrl Pts',(0.366514216845,-37.9742356128,-2.00024704769));
#66691=CARTESIAN_POINT('Ctrl Pts',(0.366514216845,-36.2942356128,-2.00024704769));
#66692=CARTESIAN_POINT('Ctrl Pts',(0.122728100002,-37.9742356128,-2.02484094933));
#66693=CARTESIAN_POINT('Ctrl Pts',(0.122728100002,-36.2942356128,-2.02484094933));
#66694=CARTESIAN_POINT('Ctrl Pts',(-0.122728100002,-37.9742356128,-2.02484094933));
#66695=CARTESIAN_POINT('Ctrl Pts',(-0.122728100002,-36.2942356128,-2.02484094933));
#66696=CARTESIAN_POINT('Ctrl Pts',(-0.366514216845,-37.9742356128,-2.00024704769));
#66697=CARTESIAN_POINT('Ctrl Pts',(-0.366514216845,-36.2942356128,-2.00024704769));
#66698=CARTESIAN_POINT('Ctrl Pts',(-0.605290084208,-37.9742356128,-1.95105924441));
#66699=CARTESIAN_POINT('Ctrl Pts',(-0.605290084208,-36.2942356128,-1.95105924441));
#66700=CARTESIAN_POINT('',(-0.605290084208,-37.2742356128,-1.95105924441));
#66701=CARTESIAN_POINT('Ctrl Pts',(-0.665819092629,-36.2742356128,-2.2448895341));
#66702=CARTESIAN_POINT('Ctrl Pts',(-0.64680334381,-36.2742356128,-2.15258002616));
#66703=CARTESIAN_POINT('Ctrl Pts',(-0.627787594992,-36.3112466293,-2.06027051821));
#66704=CARTESIAN_POINT('Ctrl Pts',(-0.612757551307,-36.3857400536,-1.98730910342));
#66705=CARTESIAN_POINT('Ctrl Pts',(-0.605290084208,-36.4799878332,-1.95105924441));
#66706=CARTESIAN_POINT('Ctrl Pts',(-0.605290084208,-36.5742356128,-1.95105924441));
#66707=CARTESIAN_POINT('Ctrl Pts',(-0.993149878416,-36.2742356128,-2.17745942705));
#66708=CARTESIAN_POINT('Ctrl Pts',(-0.969939828056,-36.2742356128,-2.08601394477));
#66709=CARTESIAN_POINT('Ctrl Pts',(-0.946729777696,-36.3112466293,-1.9945684625));
#66710=CARTESIAN_POINT('Ctrl Pts',(-0.928384559091,-36.3857400536,-1.92228997336));
#66711=CARTESIAN_POINT('Ctrl Pts',(-0.919269993533,-36.4799878332,-1.88637941649));
#66712=CARTESIAN_POINT('Ctrl Pts',(-0.919269993533,-36.5742356128,-1.88637941649));
#66713=CARTESIAN_POINT('Ctrl Pts',(-1.31927689012,-36.2742356128,-2.09049838771));
#66714=CARTESIAN_POINT('Ctrl Pts',(-1.29146795967,-36.2742356128,-2.00028752065));
#66715=CARTESIAN_POINT('Ctrl Pts',(-1.26365902922,-36.3112466293,-1.91007665359));
#66716=CARTESIAN_POINT('Ctrl Pts',(-1.24167885673,-36.3857400536,-1.83877400414));
#66717=CARTESIAN_POINT('Ctrl Pts',(-1.23075831525,-36.4799878332,-1.80334827944));
#66718=CARTESIAN_POINT('Ctrl Pts',(-1.23075831525,-36.5742356128,-1.80334827944));
#66719=CARTESIAN_POINT('Ctrl Pts',(-1.64288399014,-36.2742356128,-1.98376552099));
#66720=CARTESIAN_POINT('Ctrl Pts',(-1.6100782863,-36.2742356128,-1.89502207335));
#66721=CARTESIAN_POINT('Ctrl Pts',(-1.57727258247,-36.3112466293,-1.80627862572));
#66722=CARTESIAN_POINT('Ctrl Pts',(-1.551342962,-36.3857400536,-1.73613582402));
#66723=CARTESIAN_POINT('Ctrl Pts',(-1.53846019159,-36.4799878332,-1.70128635382));
#66724=CARTESIAN_POINT('Ctrl Pts',(-1.53846019159,-36.5742356128,-1.70128635382));
#66725=CARTESIAN_POINT('Ctrl Pts',(-2.20014530314,-36.2742356128,-1.7420059745));
#66726=CARTESIAN_POINT('Ctrl Pts',(-2.15552738159,-36.2742356128,-1.65820058714));
#66727=CARTESIAN_POINT('Ctrl Pts',(-2.11090946003,-36.3112466293,-1.57439519979));
#66728=CARTESIAN_POINT('Ctrl Pts',(-2.07564346457,-36.3857400536,-1.50815544015));
#66729=CARTESIAN_POINT('Ctrl Pts',(-2.05812204783,-36.4799878332,-1.47524514139));
#66730=CARTESIAN_POINT('Ctrl Pts',(-2.05812204783,-36.5742356128,-1.47524514139));
#66731=CARTESIAN_POINT('Ctrl Pts',(-2.70184643694,-36.2742356128,-1.40107771811));
#66732=CARTESIAN_POINT('Ctrl Pts',(-2.64463417724,-36.2742356128,-1.32575196136));
#66733=CARTESIAN_POINT('Ctrl Pts',(-2.58742191754,-36.3112466293,-1.2504262046));
#66734=CARTESIAN_POINT('Ctrl Pts',(-2.54220135981,-36.3857400536,-1.19088874298));
#66735=CARTESIAN_POINT('Ctrl Pts',(-2.51973415821,-36.4799878332,-1.16130838751));
#66736=CARTESIAN_POINT('Ctrl Pts',(-2.51973415821,-36.5742356128,-1.16130838751));
#66737=CARTESIAN_POINT('Ctrl Pts',(-2.90464199721,-36.2742356128,-1.23493234649));
#66738=CARTESIAN_POINT('Ctrl Pts',(-2.84222259825,-36.2742356128,-1.16389392384));
#66739=CARTESIAN_POINT('Ctrl Pts',(-2.77980319928,-36.3112466293,-1.09285550119));
#66740=CARTESIAN_POINT('Ctrl Pts',(-2.73046692003,-36.3857400536,-1.03670674729));
#66741=CARTESIAN_POINT('Ctrl Pts',(-2.70595487941,-36.4799878332,-1.00881002421));
#66742=CARTESIAN_POINT('Ctrl Pts',(-2.70595487941,-36.5742356128,-1.00881002421));
#66743=CARTESIAN_POINT('Ctrl Pts',(-3.33998426273,-36.2742356128,-0.811260038282));
#66744=CARTESIAN_POINT('Ctrl Pts',(-3.26725361199,-36.2742356128,-0.750410980921));
#66745=CARTESIAN_POINT('Ctrl Pts',(-3.19452296125,-36.3112466293,-0.68956192356));
#66746=CARTESIAN_POINT('Ctrl Pts',(-3.13703667098,-36.3857400536,-0.64146684195));
#66747=CARTESIAN_POINT('Ctrl Pts',(-3.10847541114,-36.4799878332,-0.617571473053));
#66748=CARTESIAN_POINT('Ctrl Pts',(-3.10847541114,-36.5742356128,-0.617571473053));
#66749=CARTESIAN_POINT('Ctrl Pts',(-3.69323929211,-36.2742356128,-0.324903072136));
#66750=CARTESIAN_POINT('Ctrl Pts',(-3.61456370902,-36.2742356128,-0.272640413673));
#66751=CARTESIAN_POINT('Ctrl Pts',(-3.53588812594,-36.3112466293,-0.220377755209));
#66752=CARTESIAN_POINT('Ctrl Pts',(-3.47370296218,-36.3857400536,-0.17906936204));
#66753=CARTESIAN_POINT('Ctrl Pts',(-3.44280713313,-36.4799878332,-0.158545863464));
#66754=CARTESIAN_POINT('Ctrl Pts',(-3.44280713313,-36.5742356128,-0.158545863464));
#66755=CARTESIAN_POINT('Ctrl Pts',(-3.87117184632,-36.2742356128,-0.0435637631917));
#66756=CARTESIAN_POINT('Ctrl Pts',(-3.79075207379,-36.2742356128,0.00579319803729));
#66757=CARTESIAN_POINT('Ctrl Pts',(-3.71033230126,-36.3112466293,0.0551501592663));
#66758=CARTESIAN_POINT('Ctrl Pts',(-3.64676853057,-36.3857400536,0.0941618898987));
#66759=CARTESIAN_POINT('Ctrl Pts',(-3.6151877599,-36.4799878332,0.11354432392));
#66760=CARTESIAN_POINT('Ctrl Pts',(-3.6151877599,-36.5742356128,0.11354432392));
#66761=CARTESIAN_POINT('Ctrl Pts',(-4.16626079964,-36.2742356128,0.473398136763));
#66762=CARTESIAN_POINT('Ctrl Pts',(-4.0822299908,-36.2742356128,0.516477026574));
#66763=CARTESIAN_POINT('Ctrl Pts',(-3.99819918195,-36.3112466293,0.559555916386));
#66764=CARTESIAN_POINT('Ctrl Pts',(-3.93178124925,-36.3857400536,0.593605461971));
#66765=CARTESIAN_POINT('Ctrl Pts',(-3.89878242765,-36.4799878332,0.610522501891));
#66766=CARTESIAN_POINT('Ctrl Pts',(-3.89878242765,-36.5742356128,0.610522501891));
#66767=CARTESIAN_POINT('Ctrl Pts',(-4.40933595991,-36.2742356128,1.0118987705));
#66768=CARTESIAN_POINT('Ctrl Pts',(-4.32247527463,-36.2742356128,1.04863663853));
#66769=CARTESIAN_POINT('Ctrl Pts',(-4.23561458935,-36.3112466293,1.08537450657));
#66770=CARTESIAN_POINT('Ctrl Pts',(-4.16695992269,-36.3857400536,1.11441210894));
#66771=CARTESIAN_POINT('Ctrl Pts',(-4.13284981146,-36.4799878332,1.12883903643));
#66772=CARTESIAN_POINT('Ctrl Pts',(-4.13284981146,-36.5742356128,1.12883903643));
#66773=CARTESIAN_POINT('Ctrl Pts',(-4.50885918571,-36.2742356128,1.25857748739));
#66774=CARTESIAN_POINT('Ctrl Pts',(-4.42076765288,-36.2742356128,1.29228565071));
#66775=CARTESIAN_POINT('Ctrl Pts',(-4.33267612006,-36.3112466293,1.32599381403));
#66776=CARTESIAN_POINT('Ctrl Pts',(-4.26304859229,-36.3857400536,1.35263674045));
#66777=CARTESIAN_POINT('Ctrl Pts',(-4.22845512783,-36.4799878332,1.36587390368));
#66778=CARTESIAN_POINT('Ctrl Pts',(-4.22845512783,-36.5742356128,1.36587390368));
#66779=CARTESIAN_POINT('Ctrl Pts',(-4.59842586631,-36.2742356128,1.51040085421));
#66780=CARTESIAN_POINT('Ctrl Pts',(-4.50933622176,-36.2742356128,1.54130452507));
#66781=CARTESIAN_POINT('Ctrl Pts',(-4.42024657721,-36.3112466293,1.57220819593));
#66782=CARTESIAN_POINT('Ctrl Pts',(-4.34983014146,-36.3857400536,1.59663444954));
#66783=CARTESIAN_POINT('Ctrl Pts',(-4.31484472014,-36.4799878332,1.60877029375));
#66784=CARTESIAN_POINT('Ctrl Pts',(-4.31484472014,-36.5742356128,1.60877029375));
#66785=CARTESIAN_POINT('Ctrl Pts',(-4.67790780735,-36.2742356128,1.7660244085));
#66786=CARTESIAN_POINT('Ctrl Pts',(-4.58791007919,-36.2742356128,1.79400748948));
#66787=CARTESIAN_POINT('Ctrl Pts',(-4.49791235104,-36.3112466293,1.82199057046));
#66788=CARTESIAN_POINT('Ctrl Pts',(-4.42677816649,-36.3857400536,1.84410839151));
#66789=CARTESIAN_POINT('Ctrl Pts',(-4.39143614129,-36.4799878332,1.85509732172));
#66790=CARTESIAN_POINT('Ctrl Pts',(-4.39143614129,-36.5742356128,1.85509732172));
#66791=CARTESIAN_POINT('Ctrl Pts',(-0.605290084208,-36.5742356128,-1.95105924441));
#66792=CARTESIAN_POINT('Ctrl Pts',(-0.829298136681,-36.5742356128,-1.90491360943));
#66793=CARTESIAN_POINT('Ctrl Pts',(-1.05244809907,-36.5742356128,-1.84948241265));
#66794=CARTESIAN_POINT('Ctrl Pts',(-1.27374925479,-36.5742356128,-1.78401007325));
#66795=CARTESIAN_POINT('Ctrl Pts',(-1.82079921196,-36.5742356128,-1.59087876764));
#66796=CARTESIAN_POINT('Ctrl Pts',(-2.32845991742,-36.5742356128,-1.31278717238));
#66797=CARTESIAN_POINT('Ctrl Pts',(-2.60729776969,-36.5742356128,-1.11027831961));
#66798=CARTESIAN_POINT('Ctrl Pts',(-2.94243947089,-36.5742356128,-0.791306229273));
#66799=CARTESIAN_POINT('Ctrl Pts',(-3.23153488576,-36.5742356128,-0.431337329712));
#66800=CARTESIAN_POINT('Ctrl Pts',(-3.30090973533,-36.5742356128,-0.339360369535));
#66801=CARTESIAN_POINT('Ctrl Pts',(-3.5009243649,-36.5742356128,-0.0596747683079));
#66802=CARTESIAN_POINT('Ctrl Pts',(-3.67911538599,-36.5742356128,0.229327428773));
#66803=CARTESIAN_POINT('Ctrl Pts',(-3.7899456945,-36.5742356128,0.424245491898));
#66804=CARTESIAN_POINT('Ctrl Pts',(-3.99431489394,-36.5742356128,0.816003179174));
#66805=CARTESIAN_POINT('Ctrl Pts',(-4.17012108382,-36.5742356128,1.22254846374));
#66806=CARTESIAN_POINT('Ctrl Pts',(-4.25088448198,-36.5742356128,1.42950202983));
#66807=CARTESIAN_POINT('Ctrl Pts',(-4.32485281869,-36.5742356128,1.64095842297));
#66808=CARTESIAN_POINT('Ctrl Pts',(-4.39143626207,-36.5742356128,1.85509771048));
#66809=CARTESIAN_POINT('Ctrl Pts',(-4.39143629673,-37.9742356128,1.85509783551));
#66810=CARTESIAN_POINT('Ctrl Pts',(-4.39143629608,-38.0684833924,1.85509783338));
#66811=CARTESIAN_POINT('Ctrl Pts',(-4.4267783216,-38.162731172,1.84410890455));
#66812=CARTESIAN_POINT('Ctrl Pts',(-4.49791250759,-38.2372245963,1.82199108888));
#66813=CARTESIAN_POINT('Ctrl Pts',(-4.58791023798,-38.2742356128,1.794008016));
#66814=CARTESIAN_POINT('Ctrl Pts',(-4.67790796861,-38.2742356128,1.76602494395));
#66815=CARTESIAN_POINT('Ctrl Pts',(-4.32501378909,-37.9742356128,1.64147451647));
#66816=CARTESIAN_POINT('Ctrl Pts',(-4.32501382176,-38.0684833927,1.64147462346));
#66817=CARTESIAN_POINT('Ctrl Pts',(-4.36004662084,-38.1627311725,1.62949113947));
#66818=CARTESIAN_POINT('Ctrl Pts',(-4.43055837533,-38.2372245969,1.60537141509));
#66819=CARTESIAN_POINT('Ctrl Pts',(-4.51976859564,-38.2742356132,1.57485549503));
#66820=CARTESIAN_POINT('Ctrl Pts',(-4.608978803,-38.2742356128,1.54433953306));
#66821=CARTESIAN_POINT('Ctrl Pts',(-4.25125101365,-37.9742356128,1.4305487941));
#66822=CARTESIAN_POINT('Ctrl Pts',(-4.25125097569,-38.0684833922,1.43054866879));
#66823=CARTESIAN_POINT('Ctrl Pts',(-4.28594766261,-38.1627311716,1.41760586681));
#66824=CARTESIAN_POINT('Ctrl Pts',(-4.35578299682,-38.2372245958,1.39155556675));
#66825=CARTESIAN_POINT('Ctrl Pts',(-4.44413746573,-38.2742356125,1.35859725952));
#66826=CARTESIAN_POINT('Ctrl Pts',(-4.53249194964,-38.2742356128,1.32563900137));
#66827=CARTESIAN_POINT('Ctrl Pts',(-4.17047868854,-37.9742356128,1.22369574326));
#66828=CARTESIAN_POINT('Ctrl Pts',(-4.17047869492,-38.0684833917,1.22369577109));
#66829=CARTESIAN_POINT('Ctrl Pts',(-4.2047722621,-38.1627311705,1.20973057696));
#66830=CARTESIAN_POINT('Ctrl Pts',(-4.27379616937,-38.2372245945,1.18162228786));
#66831=CARTESIAN_POINT('Ctrl Pts',(-4.36112400783,-38.2742356116,1.14606015377));
#66832=CARTESIAN_POINT('Ctrl Pts',(-4.44845184422,-38.2742356128,1.11049800854));
#66833=CARTESIAN_POINT('Ctrl Pts',(-3.93989107509,-37.9742356128,0.689524409198));
#66834=CARTESIAN_POINT('Ctrl Pts',(-3.93989106463,-38.0684833937,0.689524363603));
#66835=CARTESIAN_POINT('Ctrl Pts',(-3.97309480476,-38.1627311746,0.672998474686));
#66836=CARTESIAN_POINT('Ctrl Pts',(-4.03992519733,-38.2372245994,0.639736268972));
#66837=CARTESIAN_POINT('Ctrl Pts',(-4.12447784909,-38.2742356149,0.597653535716));
#66838=CARTESIAN_POINT('Ctrl Pts',(-4.20903050423,-38.2742356128,0.555570820727));
#66839=CARTESIAN_POINT('Ctrl Pts',(-3.65912020129,-37.9742356128,0.180829797996));
#66840=CARTESIAN_POINT('Ctrl Pts',(-3.65912021842,-38.0684833903,0.180829872687));
#66841=CARTESIAN_POINT('Ctrl Pts',(-3.69090252358,-38.1627311678,0.161760353725));
#66842=CARTESIAN_POINT('Ctrl Pts',(-3.75487190895,-38.2372245914,0.123378347174));
#66843=CARTESIAN_POINT('Ctrl Pts',(-3.83580484849,-38.2742356095,0.0748180560692));
#66844=CARTESIAN_POINT('Ctrl Pts',(-3.91673778248,-38.2742356128,0.0262577350419));
#66845=CARTESIAN_POINT('Ctrl Pts',(-3.46498418373,-37.9742356128,-0.132403747894));
#66846=CARTESIAN_POINT('Ctrl Pts',(-3.46498418837,-38.0684833888,-0.132403740127));
#66847=CARTESIAN_POINT('Ctrl Pts',(-3.49608533501,-38.1627311648,-0.152658499093));
#66848=CARTESIAN_POINT('Ctrl Pts',(-3.55868374308,-38.2372245878,-0.193425999957));
#66849=CARTESIAN_POINT('Ctrl Pts',(-3.63788215363,-38.2742356071,-0.245004336915));
#66850=CARTESIAN_POINT('Ctrl Pts',(-3.71708056344,-38.2742356128,-0.296582679048));
#66851=CARTESIAN_POINT('Ctrl Pts',(-3.0835957445,-37.9742356128,-0.658993075077));
#66852=CARTESIAN_POINT('Ctrl Pts',(-3.083595741,-38.0684833952,-0.658993080934));
#66853=CARTESIAN_POINT('Ctrl Pts',(-3.11202351027,-38.1627311775,-0.683181209926));
#66854=CARTESIAN_POINT('Ctrl Pts',(-3.16924112354,-38.2372246028,-0.731865533214));
#66855=CARTESIAN_POINT('Ctrl Pts',(-3.2416318504,-38.2742356171,-0.793460084306));
#66856=CARTESIAN_POINT('Ctrl Pts',(-3.31402257782,-38.2742356128,-0.855054631493));
#66857=CARTESIAN_POINT('Ctrl Pts',(-2.61204098849,-37.9742356128,-1.09317303329));
#66858=CARTESIAN_POINT('Ctrl Pts',(-2.61204099113,-38.0684833904,-1.09317302887));
#66859=CARTESIAN_POINT('Ctrl Pts',(-2.63556888179,-38.1627311679,-1.12196789197));
#66860=CARTESIAN_POINT('Ctrl Pts',(-2.68292432324,-38.2372245915,-1.17992437049));
#66861=CARTESIAN_POINT('Ctrl Pts',(-2.74283759961,-38.2742356096,-1.25324989821));
#66862=CARTESIAN_POINT('Ctrl Pts',(-2.80275087556,-38.2742356128,-1.32657542887));
#66863=CARTESIAN_POINT('Ctrl Pts',(-2.39238741385,-37.9742356128,-1.25827080622));
#66864=CARTESIAN_POINT('Ctrl Pts',(-2.3923874135,-38.0684833927,-1.2582708065));
#66865=CARTESIAN_POINT('Ctrl Pts',(-2.41346117499,-38.1627311726,-1.28891123921));
#66866=CARTESIAN_POINT('Ctrl Pts',(-2.45587704856,-38.2372245969,-1.3505823687));
#66867=CARTESIAN_POINT('Ctrl Pts',(-2.50954089479,-38.2742356132,-1.4286075996));
#66868=CARTESIAN_POINT('Ctrl Pts',(-2.56320474031,-38.2742356128,-1.50663283058));
#66869=CARTESIAN_POINT('Ctrl Pts',(-1.92260910415,-37.9742356128,-1.54188431467));
#66870=CARTESIAN_POINT('Ctrl Pts',(-1.9226091045,-38.0684833922,-1.54188431439));
#66871=CARTESIAN_POINT('Ctrl Pts',(-1.93875777533,-38.1627311716,-1.57542603916));
#66872=CARTESIAN_POINT('Ctrl Pts',(-1.97126085078,-38.2372245957,-1.6429366818));
#66873=CARTESIAN_POINT('Ctrl Pts',(-2.01238315046,-38.2742356124,-1.72834997312));
#66874=CARTESIAN_POINT('Ctrl Pts',(-2.05350545084,-38.2742356128,-1.81376326435));
#66875=CARTESIAN_POINT('Ctrl Pts',(-1.4052886958,-37.9742356128,-1.74401925817));
#66876=CARTESIAN_POINT('Ctrl Pts',(-1.40528869546,-38.0684833927,-1.74401925844));
#66877=CARTESIAN_POINT('Ctrl Pts',(-1.4173138436,-38.1627311726,-1.77911246411));
#66878=CARTESIAN_POINT('Ctrl Pts',(-1.4415172419,-38.2372245969,-1.84974585166));
#66879=CARTESIAN_POINT('Ctrl Pts',(-1.47213898278,-38.2742356132,-1.93910997524));
#66880=CARTESIAN_POINT('Ctrl Pts',(-1.50276072296,-38.2742356128,-2.0284740989));
#66881=CARTESIAN_POINT('Ctrl Pts',(-1.14123834365,-37.9742356128,-1.82695117915));
#66882=CARTESIAN_POINT('Ctrl Pts',(-1.14123836074,-38.0684834104,-1.82695117356));
#66883=CARTESIAN_POINT('Ctrl Pts',(-1.15164521742,-38.162731208,-1.86251803088));
#66884=CARTESIAN_POINT('Ctrl Pts',(-1.17259168066,-38.2372246386,-1.9341047041));
#66885=CARTESIAN_POINT('Ctrl Pts',(-1.19909267267,-38.274235641,-2.0246749291));
#66886=CARTESIAN_POINT('Ctrl Pts',(-1.22559365574,-38.2742356128,-2.11524514549));
#66887=CARTESIAN_POINT('Ctrl Pts',(-0.874174535988,-37.9742356128,-1.89566907595));
#66888=CARTESIAN_POINT('Ctrl Pts',(-0.874174535988,-38.0684833924,-1.89566907595));
#66889=CARTESIAN_POINT('Ctrl Pts',(-0.88305258586,-38.1627311721,-1.93162835504));
#66890=CARTESIAN_POINT('Ctrl Pts',(-0.900921611695,-38.2372245963,-2.00400493982));
#66891=CARTESIAN_POINT('Ctrl Pts',(-0.923529254725,-38.2742356128,-2.09557451794));
#66892=CARTESIAN_POINT('Ctrl Pts',(-0.946136897282,-38.2742356128,-2.18714409616));
#66893=CARTESIAN_POINT('Ctrl Pts',(-0.605290084208,-37.9742356128,-1.95105924441));
#66894=CARTESIAN_POINT('Ctrl Pts',(-0.605290084208,-38.0684833924,-1.95105924441));
#66895=CARTESIAN_POINT('Ctrl Pts',(-0.612757551307,-38.1627311721,-1.98730910342));
#66896=CARTESIAN_POINT('Ctrl Pts',(-0.627787594992,-38.2372245963,-2.06027051821));
#66897=CARTESIAN_POINT('Ctrl Pts',(-0.64680334381,-38.2742356128,-2.15258002616));
#66898=CARTESIAN_POINT('Ctrl Pts',(-0.665819092629,-38.2742356128,-2.2448895341));
#66899=CARTESIAN_POINT('Ctrl Pts',(-0.605290084208,-37.9742356128,-1.95105924441));
#66900=CARTESIAN_POINT('Ctrl Pts',(-0.829298136681,-37.9742356128,-1.90491360943));
#66901=CARTESIAN_POINT('Ctrl Pts',(-1.05244809907,-37.9742356128,-1.84948241265));
#66902=CARTESIAN_POINT('Ctrl Pts',(-1.27374925479,-37.9742356128,-1.78401007325));
#66903=CARTESIAN_POINT('Ctrl Pts',(-1.82079921196,-37.9742356128,-1.59087876764));
#66904=CARTESIAN_POINT('Ctrl Pts',(-2.32845991742,-37.9742356128,-1.31278717238));
#66905=CARTESIAN_POINT('Ctrl Pts',(-2.60729776969,-37.9742356128,-1.11027831961));
#66906=CARTESIAN_POINT('Ctrl Pts',(-2.94243947089,-37.9742356128,-0.791306229273));
#66907=CARTESIAN_POINT('Ctrl Pts',(-3.23153488576,-37.9742356128,-0.431337329712));
#66908=CARTESIAN_POINT('Ctrl Pts',(-3.30090973533,-37.9742356128,-0.339360369535));
#66909=CARTESIAN_POINT('Ctrl Pts',(-3.5009243649,-37.9742356128,-0.0596747683079));
#66910=CARTESIAN_POINT('Ctrl Pts',(-3.67911538599,-37.9742356128,0.229327428773));
#66911=CARTESIAN_POINT('Ctrl Pts',(-3.7899456945,-37.9742356128,0.424245491898));
#66912=CARTESIAN_POINT('Ctrl Pts',(-3.99431489394,-37.9742356128,0.816003179174));
#66913=CARTESIAN_POINT('Ctrl Pts',(-4.17012108382,-37.9742356128,1.22254846374));
#66914=CARTESIAN_POINT('Ctrl Pts',(-4.25088448198,-37.9742356128,1.42950202983));
#66915=CARTESIAN_POINT('Ctrl Pts',(-4.32485281869,-37.9742356128,1.64095842297));
#66916=CARTESIAN_POINT('Ctrl Pts',(-4.39143626207,-37.9742356128,1.85509771048));
#66917=CARTESIAN_POINT('Ctrl Pts',(-0.605290084208,-37.9742356128,-1.95105924441));
#66918=CARTESIAN_POINT('Ctrl Pts',(-0.605290084208,-36.2942356128,-1.95105924441));
#66919=CARTESIAN_POINT('Ctrl Pts',(-0.829298136681,-37.9742356128,-1.90491360943));
#66920=CARTESIAN_POINT('Ctrl Pts',(-0.829298136681,-36.2942356128,-1.90491360943));
#66921=CARTESIAN_POINT('Ctrl Pts',(-1.05244809907,-37.9742356128,-1.84948241265));
#66922=CARTESIAN_POINT('Ctrl Pts',(-1.05244809907,-36.2942356128,-1.84948241265));
#66923=CARTESIAN_POINT('Ctrl Pts',(-1.27374925479,-37.9742356128,-1.78401007325));
#66924=CARTESIAN_POINT('Ctrl Pts',(-1.27374925479,-36.2942356128,-1.78401007325));
#66925=CARTESIAN_POINT('Ctrl Pts',(-1.82079921196,-37.9742356128,-1.59087876764));
#66926=CARTESIAN_POINT('Ctrl Pts',(-1.82079921196,-36.2942356128,-1.59087876764));
#66927=CARTESIAN_POINT('Ctrl Pts',(-2.32845991742,-37.9742356128,-1.31278717238));
#66928=CARTESIAN_POINT('Ctrl Pts',(-2.32845991742,-36.2942356128,-1.31278717238));
#66929=CARTESIAN_POINT('Ctrl Pts',(-2.60729776969,-37.9742356128,-1.11027831961));
#66930=CARTESIAN_POINT('Ctrl Pts',(-2.60729776969,-36.2942356128,-1.11027831961));
#66931=CARTESIAN_POINT('Ctrl Pts',(-2.94243947089,-37.9742356128,-0.791306229273));
#66932=CARTESIAN_POINT('Ctrl Pts',(-2.94243947089,-36.2942356128,-0.791306229273));
#66933=CARTESIAN_POINT('Ctrl Pts',(-3.23153488576,-37.9742356128,-0.431337329712));
#66934=CARTESIAN_POINT('Ctrl Pts',(-3.23153488576,-36.2942356128,-0.431337329712));
#66935=CARTESIAN_POINT('Ctrl Pts',(-3.30090973533,-37.9742356128,-0.339360369535));
#66936=CARTESIAN_POINT('Ctrl Pts',(-3.30090973533,-36.2942356128,-0.339360369535));
#66937=CARTESIAN_POINT('Ctrl Pts',(-3.5009243649,-37.9742356128,-0.0596747683079));
#66938=CARTESIAN_POINT('Ctrl Pts',(-3.5009243649,-36.2942356128,-0.0596747683079));
#66939=CARTESIAN_POINT('Ctrl Pts',(-3.67911538599,-37.9742356128,0.229327428773));
#66940=CARTESIAN_POINT('Ctrl Pts',(-3.67911538599,-36.2942356128,0.229327428773));
#66941=CARTESIAN_POINT('Ctrl Pts',(-3.7899456945,-37.9742356128,0.424245491898));
#66942=CARTESIAN_POINT('Ctrl Pts',(-3.7899456945,-36.2942356128,0.424245491898));
#66943=CARTESIAN_POINT('Ctrl Pts',(-3.99431489394,-37.9742356128,0.816003179174));
#66944=CARTESIAN_POINT('Ctrl Pts',(-3.99431489394,-36.2942356128,0.816003179174));
#66945=CARTESIAN_POINT('Ctrl Pts',(-4.17012108382,-37.9742356128,1.22254846374));
#66946=CARTESIAN_POINT('Ctrl Pts',(-4.17012108382,-36.2942356128,1.22254846374));
#66947=CARTESIAN_POINT('Ctrl Pts',(-4.25088448198,-37.9742356128,1.42950202983));
#66948=CARTESIAN_POINT('Ctrl Pts',(-4.25088448198,-36.2942356128,1.42950202983));
#66949=CARTESIAN_POINT('Ctrl Pts',(-4.32485281869,-37.9742356128,1.64095842297));
#66950=CARTESIAN_POINT('Ctrl Pts',(-4.32485281869,-36.2942356128,1.64095842297));
#66951=CARTESIAN_POINT('Ctrl Pts',(-4.39143626207,-37.9742356128,1.85509771048));
#66952=CARTESIAN_POINT('Ctrl Pts',(-4.39143626207,-36.2942356128,1.85509771048));
#66953=CARTESIAN_POINT('Ctrl Pts',(6.2749628032,-36.2742356128,2.72284536858));
#66954=CARTESIAN_POINT('Ctrl Pts',(6.35795872238,-36.2742356128,2.67818754328));
#66955=CARTESIAN_POINT('Ctrl Pts',(6.44095464156,-36.3112466293,2.63352971799));
#66956=CARTESIAN_POINT('Ctrl Pts',(6.50655459783,-36.3857400536,2.59823218269));
#66957=CARTESIAN_POINT('Ctrl Pts',(6.53914701908,-36.4799878332,2.5806950957));
#66958=CARTESIAN_POINT('Ctrl Pts',(6.53914701908,-36.5742356128,2.5806950957));
#66959=CARTESIAN_POINT('Ctrl Pts',(6.38937869213,-36.2742356128,2.93548563502));
#66960=CARTESIAN_POINT('Ctrl Pts',(6.46749860928,-36.2742356128,2.88176583084));
#66961=CARTESIAN_POINT('Ctrl Pts',(6.54561852644,-36.3112466293,2.82804602666));
#66962=CARTESIAN_POINT('Ctrl Pts',(6.60736449151,-36.3857400536,2.78558590522));
#66963=CARTESIAN_POINT('Ctrl Pts',(6.63804211152,-36.4799878332,2.76449018748));
#66964=CARTESIAN_POINT('Ctrl Pts',(6.63804211152,-36.5742356128,2.76449018748));
#66965=CARTESIAN_POINT('Ctrl Pts',(6.53170263971,-36.2742356128,3.13005192025));
#66966=CARTESIAN_POINT('Ctrl Pts',(6.60399596908,-36.2742356128,3.06855847302));
#66967=CARTESIAN_POINT('Ctrl Pts',(6.67628929845,-36.3112466293,3.0070650258));
#66968=CARTESIAN_POINT('Ctrl Pts',(6.7334299304,-36.3857400536,2.95846061908));
#66969=CARTESIAN_POINT('Ctrl Pts',(6.76181945414,-36.4799878332,2.93431219838));
#66970=CARTESIAN_POINT('Ctrl Pts',(6.76181945414,-36.5742356128,2.93431219838));
#66971=CARTESIAN_POINT('Ctrl Pts',(6.69660480532,-36.2742356128,3.30689976551));
#66972=CARTESIAN_POINT('Ctrl Pts',(6.76285398311,-36.2742356128,3.23884417488));
#66973=CARTESIAN_POINT('Ctrl Pts',(6.82910316091,-36.3112466293,3.17078858425));
#66974=CARTESIAN_POINT('Ctrl Pts',(6.88146649653,-36.3857400536,3.11699746158));
#66975=CARTESIAN_POINT('Ctrl Pts',(6.90748248775,-36.4799878332,3.09027209244));
#66976=CARTESIAN_POINT('Ctrl Pts',(6.90748248775,-36.5742356128,3.09027209244));
#66977=CARTESIAN_POINT('Ctrl Pts',(7.04173998877,-36.2742356128,3.59638619596));
#66978=CARTESIAN_POINT('Ctrl Pts',(7.09364765321,-36.2742356128,3.5158611957));
#66979=CARTESIAN_POINT('Ctrl Pts',(7.14555531764,-36.3112466293,3.43533619543));
#66980=CARTESIAN_POINT('Ctrl Pts',(7.18658312387,-36.3857400536,3.37168925288));
#66981=CARTESIAN_POINT('Ctrl Pts',(7.20696721636,-36.4799878332,3.34006715926));
#66982=CARTESIAN_POINT('Ctrl Pts',(7.20696721636,-36.5742356128,3.34006715926));
#66983=CARTESIAN_POINT('Ctrl Pts',(7.47286173787,-36.2742356128,3.78624010848));
#66984=CARTESIAN_POINT('Ctrl Pts',(7.50303684285,-36.2742356128,3.69590303443));
#66985=CARTESIAN_POINT('Ctrl Pts',(7.53321194782,-36.3112466293,3.60556596038));
#66986=CARTESIAN_POINT('Ctrl Pts',(7.55706234467,-36.3857400536,3.53416355611));
#66987=CARTESIAN_POINT('Ctrl Pts',(7.56891208017,-36.4799878332,3.49868827089));
#66988=CARTESIAN_POINT('Ctrl Pts',(7.56891208017,-36.5742356128,3.49868827089));
#66989=CARTESIAN_POINT('Ctrl Pts',(7.68849344064,-36.2742356128,3.84462968135));
#66990=CARTESIAN_POINT('Ctrl Pts',(7.70659023707,-36.2742356128,3.7507417713));
#66991=CARTESIAN_POINT('Ctrl Pts',(7.7246870335,-36.3112466293,3.65685386124));
#66992=CARTESIAN_POINT('Ctrl Pts',(7.73899073929,-36.3857400536,3.58264487732));
#66993=CARTESIAN_POINT('Ctrl Pts',(7.74609733275,-36.4799878332,3.54577518171));
#66994=CARTESIAN_POINT('Ctrl Pts',(7.74609733275,-36.5742356128,3.54577518171));
#66995=CARTESIAN_POINT('Ctrl Pts',(8.13777558599,-36.2742356128,3.88392944679));
#66996=CARTESIAN_POINT('Ctrl Pts',(8.12954327989,-36.2742356128,3.78776614015));
#66997=CARTESIAN_POINT('Ctrl Pts',(8.12131097379,-36.3112466293,3.6916028335));
#66998=CARTESIAN_POINT('Ctrl Pts',(8.11480416094,-36.3857400536,3.61559537748));
#66999=CARTESIAN_POINT('Ctrl Pts',(8.11157134181,-36.4799878332,3.57783213485));
#67000=CARTESIAN_POINT('Ctrl Pts',(8.11157134181,-36.5742356128,3.57783213485));
#67001=CARTESIAN_POINT('Ctrl Pts',(8.57834470762,-36.2742356128,3.76769789992));
#67002=CARTESIAN_POINT('Ctrl Pts',(8.54396564062,-36.2742356128,3.67834598136));
#67003=CARTESIAN_POINT('Ctrl Pts',(8.50958657363,-36.3112466293,3.5889940628));
#67004=CARTESIAN_POINT('Ctrl Pts',(8.48241336454,-36.3857400536,3.51837032565));
#67005=CARTESIAN_POINT('Ctrl Pts',(8.4689127386,-36.4799878332,3.48328190964));
#67006=CARTESIAN_POINT('Ctrl Pts',(8.4689127386,-36.5742356128,3.48328190964));
#67007=CARTESIAN_POINT('Ctrl Pts',(8.78308533434,-36.2742356128,3.66972997816));
#67008=CARTESIAN_POINT('Ctrl Pts',(8.73702748426,-36.2742356128,3.58626986161));
#67009=CARTESIAN_POINT('Ctrl Pts',(8.69096963417,-36.3112466293,3.50280974507));
#67010=CARTESIAN_POINT('Ctrl Pts',(8.65456547339,-36.3857400536,3.43684296027));
#67011=CARTESIAN_POINT('Ctrl Pts',(8.63647864415,-36.4799878332,3.40406817618));
#67012=CARTESIAN_POINT('Ctrl Pts',(8.63647864415,-36.5742356128,3.40406817618));
#67013=CARTESIAN_POINT('Ctrl Pts',(9.14359313033,-36.2742356128,3.42239438786));
#67014=CARTESIAN_POINT('Ctrl Pts',(9.07931134809,-36.2742356128,3.35190041238));
#67015=CARTESIAN_POINT('Ctrl Pts',(9.01502956586,-36.3112466293,3.28140643689));
#67016=CARTESIAN_POINT('Ctrl Pts',(8.96422130469,-36.3857400536,3.22568794017));
#67017=CARTESIAN_POINT('Ctrl Pts',(8.93897786246,-36.4799878332,3.19800509473));
#67018=CARTESIAN_POINT('Ctrl Pts',(8.93897786246,-36.5742356128,3.19800509473));
#67019=CARTESIAN_POINT('Ctrl Pts',(9.41617922373,-36.2742356128,3.11420778463));
#67020=CARTESIAN_POINT('Ctrl Pts',(9.34219142116,-36.2742356128,3.05525548641));
#67021=CARTESIAN_POINT('Ctrl Pts',(9.2682036186,-36.3112466293,2.99630318818));
#67022=CARTESIAN_POINT('Ctrl Pts',(9.20972363117,-36.3857400536,2.94970737964));
#67023=CARTESIAN_POINT('Ctrl Pts',(9.1806687336,-36.4799878332,2.92655679125));
#67024=CARTESIAN_POINT('Ctrl Pts',(9.1806687336,-36.5742356128,2.92655679125));
#67025=CARTESIAN_POINT('Ctrl Pts',(9.53134305607,-36.2742356128,2.95704414661));
#67026=CARTESIAN_POINT('Ctrl Pts',(9.45451736556,-36.2742356128,2.90229899704));
#67027=CARTESIAN_POINT('Ctrl Pts',(9.37769167505,-36.3112466293,2.84755384746));
#67028=CARTESIAN_POINT('Ctrl Pts',(9.31696884576,-36.3857400536,2.80428299887));
#67029=CARTESIAN_POINT('Ctrl Pts',(9.28679928804,-36.4799878332,2.78278492331));
#67030=CARTESIAN_POINT('Ctrl Pts',(9.28679928804,-36.5742356128,2.78278492331));
#67031=CARTESIAN_POINT('Ctrl Pts',(9.6338483591,-36.2742356128,2.80329114362));
#67032=CARTESIAN_POINT('Ctrl Pts',(9.55502306,-36.2742356128,2.75153288562));
#67033=CARTESIAN_POINT('Ctrl Pts',(9.47619776089,-36.3112466293,2.69977462761));
#67034=CARTESIAN_POINT('Ctrl Pts',(9.41389414223,-36.3857400536,2.65886510846));
#67035=CARTESIAN_POINT('Ctrl Pts',(9.38293963923,-36.4799878332,2.63853949148));
#67036=CARTESIAN_POINT('Ctrl Pts',(9.38293963923,-36.5742356128,2.63853949148));
#67037=CARTESIAN_POINT('Ctrl Pts',(9.7282927137,-36.2742356128,2.648549352));
#67038=CARTESIAN_POINT('Ctrl Pts',(9.64784505651,-36.2742356128,2.59944926648));
#67039=CARTESIAN_POINT('Ctrl Pts',(9.56739739932,-36.3112466293,2.55034918096));
#67040=CARTESIAN_POINT('Ctrl Pts',(9.50381158876,-36.3857400536,2.51154048417));
#67041=CARTESIAN_POINT('Ctrl Pts',(9.47221986766,-36.4799878332,2.49225892567));
#67042=CARTESIAN_POINT('Ctrl Pts',(9.47221986766,-36.5742356128,2.49225892567));
#67043=CARTESIAN_POINT('',(6.53914700256713,-36.5742356128,2.58069506468878));
#67044=CARTESIAN_POINT('Origin',(6.27683091638159,-36.5721143212222,2.72184035982094));
#67045=CARTESIAN_POINT('',(9.47221976654,-36.5742356128,2.49225909299));
#67046=CARTESIAN_POINT('Origin',(9.72648221077142,-36.572114319087,2.64744392713833));
#67047=CARTESIAN_POINT('Ctrl Pts',(6.53914701908,-36.5742356128,2.5806950957));
#67048=CARTESIAN_POINT('Ctrl Pts',(6.64407030457,-36.5742356128,2.77569349664));
#67049=CARTESIAN_POINT('Ctrl Pts',(6.77645737493,-36.5742356128,2.95406352232));
#67050=CARTESIAN_POINT('Ctrl Pts',(6.93248240874,-36.5742356128,3.11682904882));
#67051=CARTESIAN_POINT('Ctrl Pts',(7.16744129772,-36.5742356128,3.30480694269));
#67052=CARTESIAN_POINT('Ctrl Pts',(7.4430743744,-36.5742356128,3.43661441301));
#67053=CARTESIAN_POINT('Ctrl Pts',(7.51591788103,-36.5742356128,3.46603879043));
#67054=CARTESIAN_POINT('Ctrl Pts',(7.74013214217,-36.5742356128,3.53951961667));
#67055=CARTESIAN_POINT('Ctrl Pts',(7.97806372235,-36.5742356128,3.56548871191));
#67056=CARTESIAN_POINT('Ctrl Pts',(8.1397340384,-36.5742356128,3.5585372531));
#67057=CARTESIAN_POINT('Ctrl Pts',(8.37641925249,-36.5742356128,3.50886242158));
#67058=CARTESIAN_POINT('Ctrl Pts',(8.59150582736,-36.5742356128,3.41174862899));
#67059=CARTESIAN_POINT('Ctrl Pts',(8.65978894936,-36.5742356128,3.37495922004));
#67060=CARTESIAN_POINT('Ctrl Pts',(8.78922597568,-36.5742356128,3.29398598988));
#67061=CARTESIAN_POINT('Ctrl Pts',(8.90717355699,-36.5742356128,3.19917508688));
#67062=CARTESIAN_POINT('Ctrl Pts',(8.9630009386,-36.5742356128,3.14917335528));
#67063=CARTESIAN_POINT('Ctrl Pts',(9.06741515882,-36.5742356128,3.04621714461));
#67064=CARTESIAN_POINT('Ctrl Pts',(9.16069630403,-36.5742356128,2.93809779909));
#67065=CARTESIAN_POINT('Ctrl Pts',(9.20593013024,-36.5742356128,2.88194354511));
#67066=CARTESIAN_POINT('Ctrl Pts',(9.28925382834,-36.5742356128,2.77218463031));
#67067=CARTESIAN_POINT('Ctrl Pts',(9.36584102959,-36.5742356128,2.66040353433));
#67068=CARTESIAN_POINT('Ctrl Pts',(9.40258508843,-36.5742356128,2.60436998551));
#67069=CARTESIAN_POINT('Ctrl Pts',(9.43799021757,-36.5742356128,2.54834207942));
#67070=CARTESIAN_POINT('Ctrl Pts',(9.47221976654,-36.5742356128,2.49225909299));
#67071=CARTESIAN_POINT('Ctrl Pts',(9.47221982595,-37.9742356128,2.49225899398));
#67072=CARTESIAN_POINT('Ctrl Pts',(9.47221982473,-38.0684833924,2.49225899599));
#67073=CARTESIAN_POINT('Ctrl Pts',(9.50381157396,-38.1627311721,2.51154050833));
#67074=CARTESIAN_POINT('Ctrl Pts',(9.56739744262,-38.2372245963,2.55034910979));
#67075=CARTESIAN_POINT('Ctrl Pts',(9.64784517406,-38.2742356128,2.59944907346));
#67076=CARTESIAN_POINT('Ctrl Pts',(9.72829290598,-38.2742356128,2.64854903634));
#67077=CARTESIAN_POINT('Ctrl Pts',(9.30084216856,-37.9742356128,2.77305159559));
#67078=CARTESIAN_POINT('Ctrl Pts',(9.3008424815,-38.068483393,2.77305108007));
#67079=CARTESIAN_POINT('Ctrl Pts',(9.33120668218,-38.1627311731,2.79434389726));
#67080=CARTESIAN_POINT('Ctrl Pts',(9.39232167794,-38.2372245976,2.83720095717));
#67081=CARTESIAN_POINT('Ctrl Pts',(9.46964300891,-38.2742356137,2.89142344603));
#67082=CARTESIAN_POINT('Ctrl Pts',(9.54696421793,-38.2742356128,2.94564613514));
#67083=CARTESIAN_POINT('Ctrl Pts',(9.10325384448,-37.9742356128,3.047828936));
#67084=CARTESIAN_POINT('Ctrl Pts',(9.10325331016,-38.0684833792,3.04782978338));
#67085=CARTESIAN_POINT('Ctrl Pts',(9.13195333701,-38.1627311456,3.07124731643));
#67086=CARTESIAN_POINT('Ctrl Pts',(9.18971922197,-38.2372245651,3.1183802048));
#67087=CARTESIAN_POINT('Ctrl Pts',(9.26280409441,-38.274235592,3.17801114289));
#67088=CARTESIAN_POINT('Ctrl Pts',(9.33588918162,-38.2742356128,3.23764175597));
#67089=CARTESIAN_POINT('Ctrl Pts',(8.85947148585,-37.9742356128,3.32105398427));
#67090=CARTESIAN_POINT('Ctrl Pts',(8.85947171177,-38.0684834033,3.32105376337));
#67091=CARTESIAN_POINT('Ctrl Pts',(8.88406421364,-38.1627311937,3.35144391715));
#67092=CARTESIAN_POINT('Ctrl Pts',(8.93356227407,-38.2372246218,3.41261140709));
#67093=CARTESIAN_POINT('Ctrl Pts',(8.99618617025,-38.2742356298,3.4899996429));
#67094=CARTESIAN_POINT('Ctrl Pts',(9.05880997629,-38.2742356128,3.56738795876));
#67095=CARTESIAN_POINT('Ctrl Pts',(8.34379427784,-37.9742356128,3.58073008166));
#67096=CARTESIAN_POINT('Ctrl Pts',(8.34379415155,-38.0684833864,3.58073020515));
#67097=CARTESIAN_POINT('Ctrl Pts',(8.35368722351,-38.16273116,3.61862172685));
#67098=CARTESIAN_POINT('Ctrl Pts',(8.37359947265,-38.2372245821,3.69488730857));
#67099=CARTESIAN_POINT('Ctrl Pts',(8.39879220242,-38.2742356033,3.79137708216));
#67100=CARTESIAN_POINT('Ctrl Pts',(8.42398498258,-38.2742356128,3.88786681101));
#67101=CARTESIAN_POINT('Ctrl Pts',(7.79117707007,-37.9742356128,3.55728735353));
#67102=CARTESIAN_POINT('Ctrl Pts',(7.79117714067,-38.0684833958,3.5572872845));
#67103=CARTESIAN_POINT('Ctrl Pts',(7.78531841592,-38.1627311788,3.59445498488));
#67104=CARTESIAN_POINT('Ctrl Pts',(7.77352628455,-38.2372246043,3.66926381121));
#67105=CARTESIAN_POINT('Ctrl Pts',(7.75860703219,-38.2742356182,3.76391069234));
#67106=CARTESIAN_POINT('Ctrl Pts',(7.74368775165,-38.2742356128,3.85855759847));
#67107=CARTESIAN_POINT('Ctrl Pts',(7.59728307538,-37.9742356128,3.51091223408));
#67108=CARTESIAN_POINT('Ctrl Pts',(7.59728306128,-38.0684833949,3.51091223533));
#67109=CARTESIAN_POINT('Ctrl Pts',(7.58611021357,-38.1627311769,3.54668881381));
#67110=CARTESIAN_POINT('Ctrl Pts',(7.56362209461,-38.2372246021,3.61869738931));
#67111=CARTESIAN_POINT('Ctrl Pts',(7.53517058683,-38.2742356167,3.70980148529));
#67112=CARTESIAN_POINT('Ctrl Pts',(7.50671908595,-38.2742356128,3.8009055795));
#67113=CARTESIAN_POINT('Ctrl Pts',(7.21880270622,-37.9742356128,3.34989273073));
#67114=CARTESIAN_POINT('Ctrl Pts',(7.2188027215,-38.0684833898,3.34989272938));
#67115=CARTESIAN_POINT('Ctrl Pts',(7.19863591146,-38.1627311668,3.38170520801));
#67116=CARTESIAN_POINT('Ctrl Pts',(7.15804556552,-38.2372245901,3.44573561926));
#67117=CARTESIAN_POINT('Ctrl Pts',(7.10669129595,-38.2742356087,3.526745664));
#67118=CARTESIAN_POINT('Ctrl Pts',(7.05533701891,-38.2742356128,3.60775571067));
#67119=CARTESIAN_POINT('Ctrl Pts',(6.90753935367,-37.9742356128,3.09037088304));
#67120=CARTESIAN_POINT('Ctrl Pts',(6.90753933711,-38.0684833953,3.09037088451));
#67121=CARTESIAN_POINT('Ctrl Pts',(6.88153012601,-38.1627311778,3.11710058783));
#67122=CARTESIAN_POINT('Ctrl Pts',(6.82918029907,-38.237224603,3.17090013782));
#67123=CARTESIAN_POINT('Ctrl Pts',(6.76294829019,-38.2742356173,3.23896651325));
#67124=CARTESIAN_POINT('Ctrl Pts',(6.69671628941,-38.2742356128,3.30703288659));
#67125=CARTESIAN_POINT('Ctrl Pts',(6.76187341966,-37.9742356128,2.93438141705));
#67126=CARTESIAN_POINT('Ctrl Pts',(6.76187343027,-38.0684833881,2.93438143099));
#67127=CARTESIAN_POINT('Ctrl Pts',(6.7334846788,-38.1627311634,2.9585308759));
#67128=CARTESIAN_POINT('Ctrl Pts',(6.67634622409,-38.2372245862,3.00713850853));
#67129=CARTESIAN_POINT('Ctrl Pts',(6.60405537332,-38.2742356061,3.06863553104));
#67130=CARTESIAN_POINT('Ctrl Pts',(6.53176451731,-38.2742356128,3.13013255146));
#67131=CARTESIAN_POINT('Ctrl Pts',(6.63807025716,-37.9742356128,2.76454249575));
#67132=CARTESIAN_POINT('Ctrl Pts',(6.63807025716,-38.0684833924,2.76454249575));
#67133=CARTESIAN_POINT('Ctrl Pts',(6.60739332257,-38.1627311721,2.78563948738));
#67134=CARTESIAN_POINT('Ctrl Pts',(6.54564831339,-38.2372245963,2.82810138523));
#67135=CARTESIAN_POINT('Ctrl Pts',(6.46752978445,-38.2742356128,2.88182376944));
#67136=CARTESIAN_POINT('Ctrl Pts',(6.38941125501,-38.2742356128,2.93554615267));
#67137=CARTESIAN_POINT('Ctrl Pts',(6.53914701908,-37.9742356128,2.5806950957));
#67138=CARTESIAN_POINT('Ctrl Pts',(6.53914701908,-38.0684833924,2.5806950957));
#67139=CARTESIAN_POINT('Ctrl Pts',(6.50655459783,-38.1627311721,2.59823218269));
#67140=CARTESIAN_POINT('Ctrl Pts',(6.44095464156,-38.2372245963,2.63352971799));
#67141=CARTESIAN_POINT('Ctrl Pts',(6.35795872238,-38.2742356128,2.67818754328));
#67142=CARTESIAN_POINT('Ctrl Pts',(6.2749628032,-38.2742356128,2.72284536858));
#67143=CARTESIAN_POINT('',(6.53914701908,-37.9742356128,2.5806950957));
#67144=CARTESIAN_POINT('Origin',(6.27683084777394,-37.9763569039502,2.72184023891299));
#67145=CARTESIAN_POINT('',(9.47221976654,-37.9742356128,2.49225909299));
#67146=CARTESIAN_POINT('Ctrl Pts',(6.53914701908,-37.9742356128,2.5806950957));
#67147=CARTESIAN_POINT('Ctrl Pts',(6.63807025716,-37.9742356128831,2.76454249575));
#67148=CARTESIAN_POINT('Ctrl Pts',(6.76187341966,-37.9742356128831,2.93438141705));
#67149=CARTESIAN_POINT('Ctrl Pts',(6.90753935367,-37.9742356128831,3.09037088304));
#67150=CARTESIAN_POINT('Ctrl Pts',(7.21880270622,-37.9742356128831,3.34989273073));
#67151=CARTESIAN_POINT('Ctrl Pts',(7.59728307538,-37.9742356128831,3.51091223408));
#67152=CARTESIAN_POINT('Ctrl Pts',(7.79117707007001,-37.9742356128831,3.55728735353));
#67153=CARTESIAN_POINT('Ctrl Pts',(8.34379427784,-37.9742356128831,3.58073008166));
#67154=CARTESIAN_POINT('Ctrl Pts',(8.85947148585001,-37.9742356128831,3.32105398427));
#67155=CARTESIAN_POINT('Ctrl Pts',(9.10325384448,-37.9742356128831,3.047828936));
#67156=CARTESIAN_POINT('Ctrl Pts',(9.30084216856,-37.9742356128831,2.77305159559));
#67157=CARTESIAN_POINT('Ctrl Pts',(9.47221976654,-37.9742356128,2.49225909299));
#67158=CARTESIAN_POINT('Origin',(9.72648242188683,-37.9763569039244,2.64744358737807));
#67159=CARTESIAN_POINT('Ctrl Pts',(6.53914701908,-37.9742356128,2.5806950957));
#67160=CARTESIAN_POINT('Ctrl Pts',(6.53914701908,-36.2942356128,2.5806950957));
#67161=CARTESIAN_POINT('Ctrl Pts',(6.64407030457,-37.9742356128,2.77569349664));
#67162=CARTESIAN_POINT('Ctrl Pts',(6.64407030457,-36.2942356128,2.77569349664));
#67163=CARTESIAN_POINT('Ctrl Pts',(6.77645737493,-37.9742356128,2.95406352232));
#67164=CARTESIAN_POINT('Ctrl Pts',(6.77645737493,-36.2942356128,2.95406352232));
#67165=CARTESIAN_POINT('Ctrl Pts',(6.93248240874,-37.9742356128,3.11682904882));
#67166=CARTESIAN_POINT('Ctrl Pts',(6.93248240874,-36.2942356128,3.11682904882));
#67167=CARTESIAN_POINT('Ctrl Pts',(7.16744129772,-37.9742356128,3.30480694269));
#67168=CARTESIAN_POINT('Ctrl Pts',(7.16744129772,-36.2942356128,3.30480694269));
#67169=CARTESIAN_POINT('Ctrl Pts',(7.4430743744,-37.9742356128,3.43661441301));
#67170=CARTESIAN_POINT('Ctrl Pts',(7.4430743744,-36.2942356128,3.43661441301));
#67171=CARTESIAN_POINT('Ctrl Pts',(7.51591788103,-37.9742356128,3.46603879043));
#67172=CARTESIAN_POINT('Ctrl Pts',(7.51591788103,-36.2942356128,3.46603879043));
#67173=CARTESIAN_POINT('Ctrl Pts',(7.74013214217,-37.9742356128,3.53951961667));
#67174=CARTESIAN_POINT('Ctrl Pts',(7.74013214217,-36.2942356128,3.53951961667));
#67175=CARTESIAN_POINT('Ctrl Pts',(7.97806372235,-37.9742356128,3.56548871191));
#67176=CARTESIAN_POINT('Ctrl Pts',(7.97806372235,-36.2942356128,3.56548871191));
#67177=CARTESIAN_POINT('Ctrl Pts',(8.1397340384,-37.9742356128,3.5585372531));
#67178=CARTESIAN_POINT('Ctrl Pts',(8.1397340384,-36.2942356128,3.5585372531));
#67179=CARTESIAN_POINT('Ctrl Pts',(8.37641925249,-37.9742356128,3.50886242158));
#67180=CARTESIAN_POINT('Ctrl Pts',(8.37641925249,-36.2942356128,3.50886242158));
#67181=CARTESIAN_POINT('Ctrl Pts',(8.59150582736,-37.9742356128,3.41174862899));
#67182=CARTESIAN_POINT('Ctrl Pts',(8.59150582736,-36.2942356128,3.41174862899));
#67183=CARTESIAN_POINT('Ctrl Pts',(8.65978894936,-37.9742356128,3.37495922004));
#67184=CARTESIAN_POINT('Ctrl Pts',(8.65978894936,-36.2942356128,3.37495922004));
#67185=CARTESIAN_POINT('Ctrl Pts',(8.78922597568,-37.9742356128,3.29398598988));
#67186=CARTESIAN_POINT('Ctrl Pts',(8.78922597568,-36.2942356128,3.29398598988));
#67187=CARTESIAN_POINT('Ctrl Pts',(8.90717355699,-37.9742356128,3.19917508688));
#67188=CARTESIAN_POINT('Ctrl Pts',(8.90717355699,-36.2942356128,3.19917508688));
#67189=CARTESIAN_POINT('Ctrl Pts',(8.9630009386,-37.9742356128,3.14917335528));
#67190=CARTESIAN_POINT('Ctrl Pts',(8.9630009386,-36.2942356128,3.14917335528));
#67191=CARTESIAN_POINT('Ctrl Pts',(9.06741515882,-37.9742356128,3.04621714461));
#67192=CARTESIAN_POINT('Ctrl Pts',(9.06741515882,-36.2942356128,3.04621714461));
#67193=CARTESIAN_POINT('Ctrl Pts',(9.16069630403,-37.9742356128,2.93809779909));
#67194=CARTESIAN_POINT('Ctrl Pts',(9.16069630403,-36.2942356128,2.93809779909));
#67195=CARTESIAN_POINT('Ctrl Pts',(9.20593013024,-37.9742356128,2.88194354511));
#67196=CARTESIAN_POINT('Ctrl Pts',(9.20593013024,-36.2942356128,2.88194354511));
#67197=CARTESIAN_POINT('Ctrl Pts',(9.28925382834,-37.9742356128,2.77218463031));
#67198=CARTESIAN_POINT('Ctrl Pts',(9.28925382834,-36.2942356128,2.77218463031));
#67199=CARTESIAN_POINT('Ctrl Pts',(9.36584102959,-37.9742356128,2.66040353433));
#67200=CARTESIAN_POINT('Ctrl Pts',(9.36584102959,-36.2942356128,2.66040353433));
#67201=CARTESIAN_POINT('Ctrl Pts',(9.40258508843,-37.9742356128,2.60436998551));
#67202=CARTESIAN_POINT('Ctrl Pts',(9.40258508843,-36.2942356128,2.60436998551));
#67203=CARTESIAN_POINT('Ctrl Pts',(9.43799021757,-37.9742356128,2.54834207942));
#67204=CARTESIAN_POINT('Ctrl Pts',(9.43799021757,-36.2942356128,2.54834207942));
#67205=CARTESIAN_POINT('Ctrl Pts',(9.47221976654,-37.9742356128,2.49225909299));
#67206=CARTESIAN_POINT('Ctrl Pts',(9.47221976654,-36.2942356128,2.49225909299));
#67207=CARTESIAN_POINT('',(6.53914701908,-37.2742356128,2.5806950957));
#67208=CARTESIAN_POINT('',(9.47221976654,-37.2742356128,2.49225909299));
#67209=CARTESIAN_POINT('Ctrl Pts',(9.72829242121,-36.2742356128,2.64854983337));
#67210=CARTESIAN_POINT('Ctrl Pts',(9.64784482414,-36.2742356128,2.59944964919));
#67211=CARTESIAN_POINT('Ctrl Pts',(9.56739722707,-36.3112466293,2.55034946501));
#67212=CARTESIAN_POINT('Ctrl Pts',(9.50381146403,-36.3857400536,2.51154069022));
#67213=CARTESIAN_POINT('Ctrl Pts',(9.47221976654,-36.4799878332,2.49225909299));
#67214=CARTESIAN_POINT('Ctrl Pts',(9.47221976654,-36.5742356128,2.49225909299));
#67215=CARTESIAN_POINT('Ctrl Pts',(9.83429336167,-36.2742356128,2.47487388713));
#67216=CARTESIAN_POINT('Ctrl Pts',(9.75202069903,-36.2742356128,2.42876395934));
#67217=CARTESIAN_POINT('Ctrl Pts',(9.6697480364,-36.3112466293,2.38265403155));
#67218=CARTESIAN_POINT('Ctrl Pts',(9.60471974085,-36.3857400536,2.34620875598));
#67219=CARTESIAN_POINT('Ctrl Pts',(9.57241134287,-36.4799878332,2.32810142846));
#67220=CARTESIAN_POINT('Ctrl Pts',(9.57241134287,-36.5742356128,2.32810142846));
#67221=CARTESIAN_POINT('Ctrl Pts',(9.94000897933,-36.2742356128,2.28349205546));
#67222=CARTESIAN_POINT('Ctrl Pts',(9.85470074764,-36.2742356128,2.24265773253));
#67223=CARTESIAN_POINT('Ctrl Pts',(9.76939251595,-36.3112466293,2.20182340959));
#67224=CARTESIAN_POINT('Ctrl Pts',(9.70196490975,-36.3857400536,2.16954796843));
#67225=CARTESIAN_POINT('Ctrl Pts',(9.66846444414,-36.4799878332,2.15351236861));
#67226=CARTESIAN_POINT('Ctrl Pts',(9.66846444414,-36.5742356128,2.15351236861));
#67227=CARTESIAN_POINT('Ctrl Pts',(10.0256761637,-36.2742356128,2.08591224558));
#67228=CARTESIAN_POINT('Ctrl Pts',(9.93799442834,-36.2742356128,2.05066882697));
#67229=CARTESIAN_POINT('Ctrl Pts',(9.850312693,-36.3112466293,2.01542540835));
#67230=CARTESIAN_POINT('Ctrl Pts',(9.78100906698,-36.3857400536,1.98756902385));
#67231=CARTESIAN_POINT('Ctrl Pts',(9.74657653172,-36.4799878332,1.97372895991));
#67232=CARTESIAN_POINT('Ctrl Pts',(9.74657653172,-36.5742356128,1.97372895991));
#67233=CARTESIAN_POINT('Ctrl Pts',(10.1679814537,-36.2742356128,1.67805871095));
#67234=CARTESIAN_POINT('Ctrl Pts',(10.0767341523,-36.2742356128,1.65334546287));
#67235=CARTESIAN_POINT('Ctrl Pts',(9.98548685082,-36.3112466293,1.6286322148));
#67236=CARTESIAN_POINT('Ctrl Pts',(9.91336500486,-36.3857400536,1.60909886441));
#67237=CARTESIAN_POINT('Ctrl Pts',(9.87753227234,-36.4799878332,1.59939399912));
#67238=CARTESIAN_POINT('Ctrl Pts',(9.87753227234,-36.5742356128,1.59939399912));
#67239=CARTESIAN_POINT('Ctrl Pts',(10.2564553552,-36.2742356128,1.27104287483));
#67240=CARTESIAN_POINT('Ctrl Pts',(10.1638603619,-36.2742356128,1.25314895056));
#67241=CARTESIAN_POINT('Ctrl Pts',(10.0712653686,-36.3112466293,1.23525502628));
#67242=CARTESIAN_POINT('Ctrl Pts',(9.9980783059,-36.3857400536,1.22111167566));
#67243=CARTESIAN_POINT('Ctrl Pts',(9.96171633739,-36.4799878332,1.21408474484));
#67244=CARTESIAN_POINT('Ctrl Pts',(9.96171633739,-36.5742356128,1.21408474484));
#67245=CARTESIAN_POINT('Ctrl Pts',(10.2903320276,-36.2742356128,1.07432966245));
#67246=CARTESIAN_POINT('Ctrl Pts',(10.1974823607,-36.2742356128,1.05822737274));
#67247=CARTESIAN_POINT('Ctrl Pts',(10.1046326938,-36.3112466293,1.04212508303));
#67248=CARTESIAN_POINT('Ctrl Pts',(10.0312443404,-36.3857400536,1.02939781947));
#67249=CARTESIAN_POINT('Ctrl Pts',(9.99478235867,-36.4799878332,1.0230744824));
#67250=CARTESIAN_POINT('Ctrl Pts',(9.99478235867,-36.5742356128,1.0230744824));
#67251=CARTESIAN_POINT('Ctrl Pts',(10.3230522443,-36.2742356128,0.886587027226));
#67252=CARTESIAN_POINT('Ctrl Pts',(10.2301339285,-36.2742356128,0.870763630221));
#67253=CARTESIAN_POINT('Ctrl Pts',(10.1372156126,-36.3112466293,0.854940233215));
#67254=CARTESIAN_POINT('Ctrl Pts',(10.0637729945,-36.3857400536,0.842433434875));
#67255=CARTESIAN_POINT('Ctrl Pts',(10.0272840589,-36.4799878332,0.836219590227));
#67256=CARTESIAN_POINT('Ctrl Pts',(10.0272840589,-36.5742356128,0.836219590227));
#67257=CARTESIAN_POINT('Ctrl Pts',(10.3535102277,-36.2742356128,0.692259222377));
#67258=CARTESIAN_POINT('Ctrl Pts',(10.2603991896,-36.2742356128,0.677665438197));
#67259=CARTESIAN_POINT('Ctrl Pts',(10.1672881515,-36.3112466293,0.663071654016));
#67260=CARTESIAN_POINT('Ctrl Pts',(10.0936932074,-36.3857400536,0.651536730209));
#67261=CARTESIAN_POINT('Ctrl Pts',(10.0571285882,-36.4799878332,0.645805764563));
#67262=CARTESIAN_POINT('Ctrl Pts',(10.0571285882,-36.5742356128,0.645805764563));
#67263=CARTESIAN_POINT('',(10.0571285787,-36.5742356128,0.645805825719));
#67264=CARTESIAN_POINT('Origin',(10.3514145697721,-36.5721143181575,0.691930438083593));
#67265=CARTESIAN_POINT('Ctrl Pts',(9.47221976654,-36.5742356128,2.49225909299));
#67266=CARTESIAN_POINT('Ctrl Pts',(9.49100335387814,-36.5742356128,2.46148335373255));
#67267=CARTESIAN_POINT('Ctrl Pts',(9.50966311070764,-36.5742356128,2.43017846158239));
#67268=CARTESIAN_POINT('Ctrl Pts',(9.52801493081839,-36.5742356128,2.3984226649754));
#67269=CARTESIAN_POINT('Ctrl Pts',(9.54694614840981,-36.5742356128,2.36566428505843));
#67270=CARTESIAN_POINT('Ctrl Pts',(9.56554966655066,-36.5742356128,2.3324260390245));
#67271=CARTESIAN_POINT('Ctrl Pts',(9.58367847726007,-36.5742356128,2.29878225207235));
#67272=CARTESIAN_POINT('Ctrl Pts',(9.60236832147365,-36.5742356128,2.26409728861998));
#67273=CARTESIAN_POINT('Ctrl Pts',(9.62055378540715,-36.5742356128,2.22898119776554));
#67274=CARTESIAN_POINT('Ctrl Pts',(9.6381303125254,-36.5742356128,2.19350437114792));
#67275=CARTESIAN_POINT('Ctrl Pts',(9.65647984089947,-36.5742356128,2.15646730277473));
#67276=CARTESIAN_POINT('Ctrl Pts',(9.67416597091401,-36.5742356128,2.11903691913793));
#67277=CARTESIAN_POINT('Ctrl Pts',(9.69112721593196,-36.5742356128,2.08128335236617));
#67278=CARTESIAN_POINT('Ctrl Pts',(9.7086699786747,-36.5742356128,2.04223540135382));
#67279=CARTESIAN_POINT('Ctrl Pts',(9.72543795349894,-36.5742356128,2.00284146974368));
#67280=CARTESIAN_POINT('Ctrl Pts',(9.74141594767243,-36.5742356128,1.96317193046071));
#67281=CARTESIAN_POINT('Ctrl Pts',(9.7473379496166,-36.5742356128,1.94846901555118));
#67282=CARTESIAN_POINT('Ctrl Pts',(9.753149081602,-36.5742356128,1.93373509071006));
#67283=CARTESIAN_POINT('Ctrl Pts',(9.75884843233648,-36.5742356128,1.91897879964869));
#67284=CARTESIAN_POINT('Ctrl Pts',(9.78146372811979,-36.5742356128,1.86042513229877));
#67285=CARTESIAN_POINT('Ctrl Pts',(9.80232906854629,-36.5742356128,1.80148249645081));
#67286=CARTESIAN_POINT('Ctrl Pts',(9.82163170395721,-36.5742356128,1.74221229626608));
#67287=CARTESIAN_POINT('Ctrl Pts',(9.83683901853849,-36.5742356128,1.69551708805662));
#67288=CARTESIAN_POINT('Ctrl Pts',(9.8510796488562,-36.5742356128,1.64861775959349));
#67289=CARTESIAN_POINT('Ctrl Pts',(9.86444910264375,-36.5742356128,1.60155197403731));
#67290=CARTESIAN_POINT('Ctrl Pts',(9.86975108101274,-36.5742356128,1.58288690507463));
#67291=CARTESIAN_POINT('Ctrl Pts',(9.87491647744565,-36.5742356128,1.56419286401259));
#67292=CARTESIAN_POINT('Ctrl Pts',(9.87994527922462,-36.5742356128,1.54550492739863));
#67293=CARTESIAN_POINT('Ctrl Pts',(9.89160864620356,-36.5742356128,1.50216174697751));
#67294=CARTESIAN_POINT('Ctrl Pts',(9.90254290076312,-36.5742356128,1.45883011528504));
#67295=CARTESIAN_POINT('Ctrl Pts',(9.9128529548188,-36.5742356128,1.41562279736822));
#67296=CARTESIAN_POINT('Ctrl Pts',(9.92340473074946,-36.5742356128,1.37140247274521));
#67297=CARTESIAN_POINT('Ctrl Pts',(9.93330375339725,-36.5742356128,1.3273124158088));
#67298=CARTESIAN_POINT('Ctrl Pts',(9.94268006616696,-36.5742356128,1.28342079104392));
#67299=CARTESIAN_POINT('Ctrl Pts',(9.95209125516463,-36.5742356128,1.23936590654693));
#67300=CARTESIAN_POINT('Ctrl Pts',(9.96097693578902,-36.5742356128,1.19551086044026));
#67301=CARTESIAN_POINT('Ctrl Pts',(9.96946965611493,-36.5742356128,1.15187246591498));
#67302=CARTESIAN_POINT('Ctrl Pts',(9.97777858955746,-36.5742356128,1.10917842893572));
#67303=CARTESIAN_POINT('Ctrl Pts',(9.98571230740096,-36.5742356128,1.06669153948227));
#67304=CARTESIAN_POINT('Ctrl Pts',(9.99338108832957,-36.5742356128,1.0243803099396));
#67305=CARTESIAN_POINT('Ctrl Pts',(10.0007892024458,-36.5742356128,0.983507266392404));
#67306=CARTESIAN_POINT('Ctrl Pts',(10.0079507534458,-36.5742356128,0.942797893372109));
#67307=CARTESIAN_POINT('Ctrl Pts',(10.0149407365958,-36.5742356128,0.902182838501823));
#67308=CARTESIAN_POINT('Ctrl Pts',(10.021739685914,-36.5742356128,0.862677779090897));
#67309=CARTESIAN_POINT('Ctrl Pts',(10.0283768648537,-36.5742356128,0.823261802762564));
#67310=CARTESIAN_POINT('Ctrl Pts',(10.0348890100693,-36.5742356128,0.783834456310485));
#67311=CARTESIAN_POINT('Ctrl Pts',(10.0411561913072,-36.5742356128,0.745890227832604));
#67312=CARTESIAN_POINT('Ctrl Pts',(10.0473079284116,-36.5742356128,0.707935302701744));
#67313=CARTESIAN_POINT('Ctrl Pts',(10.0533402808925,-36.5742356128,0.669848094635844));
#67314=CARTESIAN_POINT('Ctrl Pts',(10.0546085605217,-36.5742356128,0.661840401074247));
#67315=CARTESIAN_POINT('Ctrl Pts',(10.0558714185436,-36.5742356128,0.653826748065928));
#67316=CARTESIAN_POINT('Ctrl Pts',(10.0571285786168,-36.5742356128,0.645805825705952));
#67317=CARTESIAN_POINT('Ctrl Pts',(10.0571274572,-37.9742356128,0.645813040595));
#67318=CARTESIAN_POINT('Ctrl Pts',(10.0571274557,-38.0684833925,0.645813050795));
#67319=CARTESIAN_POINT('Ctrl Pts',(10.0936920943,-38.1627311721,0.651543892692));
#67320=CARTESIAN_POINT('Ctrl Pts',(10.1672870793,-38.2372245964,0.663078554957));
#67321=CARTESIAN_POINT('Ctrl Pts',(10.2603981703,-38.2742356129,0.677672002041));
#67322=CARTESIAN_POINT('Ctrl Pts',(10.3535092619,-38.2742356128,0.692265445118));
#67323=CARTESIAN_POINT('Ctrl Pts',(10.0275848223,-37.9742356128,0.834300487763));
#67324=CARTESIAN_POINT('Ctrl Pts',(10.0275848525,-38.0684833923,0.834300292231));
#67325=CARTESIAN_POINT('Ctrl Pts',(10.064074095,-38.1627311719,0.840512185837));
#67326=CARTESIAN_POINT('Ctrl Pts',(10.137517286,-38.2372245961,0.853015346359));
#67327=CARTESIAN_POINT('Ctrl Pts',(10.2304363115,-38.2742356127,0.868834238919));
#67328=CARTESIAN_POINT('Ctrl Pts',(10.3233553253,-38.2742356128,0.884653208084));
#67329=CARTESIAN_POINT('Ctrl Pts',(9.99543705094,-37.9742356128,1.01939883766));
#67330=CARTESIAN_POINT('Ctrl Pts',(9.99543699511,-38.068483393,1.01939919322));
#67331=CARTESIAN_POINT('Ctrl Pts',(10.0319005469,-38.1627311731,1.0257074941));
#67332=CARTESIAN_POINT('Ctrl Pts',(10.1052921414,-38.2372245976,1.03840398068));
#67333=CARTESIAN_POINT('Ctrl Pts',(10.1981459373,-38.2742356137,1.05446714823));
#67334=CARTESIAN_POINT('Ctrl Pts',(10.2909997548,-38.2742356128,1.07053017617));
#67335=CARTESIAN_POINT('Ctrl Pts',(9.96252976109,-37.9742356128,1.2093437222));
#67336=CARTESIAN_POINT('Ctrl Pts',(9.96252977135,-38.0684833842,1.20934363522));
#67337=CARTESIAN_POINT('Ctrl Pts',(9.99889469961,-38.1627311555,1.21634966752));
#67338=CARTESIAN_POINT('Ctrl Pts',(10.0720874448,-38.2372245768,1.23045149981));
#67339=CARTESIAN_POINT('Ctrl Pts',(10.1646897356,-38.2742355998,1.24829276368));
#67340=CARTESIAN_POINT('Ctrl Pts',(10.2572920266,-38.2742356128,1.26613406435));
#67341=CARTESIAN_POINT('Ctrl Pts',(9.87888878289,-37.9742356128,1.59411409567));
#67342=CARTESIAN_POINT('Ctrl Pts',(9.87888877269,-38.0684834007,1.59411418207));
#67343=CARTESIAN_POINT('Ctrl Pts',(9.91473293696,-38.1627311885,1.60376825103));
#67344=CARTESIAN_POINT('Ctrl Pts',(9.98687806745,-38.2372246158,1.62319881203));
#67345=CARTESIAN_POINT('Ctrl Pts',(10.0781547196,-38.2742356258,1.64778214762));
#67346=CARTESIAN_POINT('Ctrl Pts',(10.1694313716,-38.2742356128,1.67236544666));
#67347=CARTESIAN_POINT('Ctrl Pts',(9.74871613381,-37.9742356128,1.96892463554));
#67348=CARTESIAN_POINT('Ctrl Pts',(9.74871614394,-38.0684833843,1.96892454973));
#67349=CARTESIAN_POINT('Ctrl Pts',(9.78317347076,-38.1627311557,1.9827075095));
#67350=CARTESIAN_POINT('Ctrl Pts',(9.85252671964,-38.237224577,2.01044951275));
#67351=CARTESIAN_POINT('Ctrl Pts',(9.94027134576,-38.2742356,2.04554808074));
#67352=CARTESIAN_POINT('Ctrl Pts',(10.028015972,-38.2742356128,2.08064668506));
#67353=CARTESIAN_POINT('Ctrl Pts',(9.67022825048,-37.9742356128,2.15028225121));
#67354=CARTESIAN_POINT('Ctrl Pts',(9.67022826459,-38.0684834011,2.15028222716));
#67355=CARTESIAN_POINT('Ctrl Pts',(9.70375002899,-38.1627311893,2.16628166859));
#67356=CARTESIAN_POINT('Ctrl Pts',(9.77122151877,-38.2372246167,2.19848267331));
#67357=CARTESIAN_POINT('Ctrl Pts',(9.85658482135,-38.2742356264,2.23922355047));
#67358=CARTESIAN_POINT('Ctrl Pts',(9.94194811633,-38.2742356128,2.27996443036));
#67359=CARTESIAN_POINT('Ctrl Pts',(9.57333706543,-37.9742356128,2.32658468963));
#67360=CARTESIAN_POINT('Ctrl Pts',(9.57333706543,-38.0684833924,2.32658468963));
#67361=CARTESIAN_POINT('Ctrl Pts',(9.60565231336,-38.1627311721,2.34468079402));
#67362=CARTESIAN_POINT('Ctrl Pts',(9.67069370749,-38.2372245963,2.38110460825));
#67363=CARTESIAN_POINT('Ctrl Pts',(9.75298323463,-38.2742356128,2.42718690466));
#67364=CARTESIAN_POINT('Ctrl Pts',(9.83527276,-38.2742356128,2.4732692039));
#67365=CARTESIAN_POINT('Ctrl Pts',(9.47221976654,-37.9742356128,2.49225909299));
#67366=CARTESIAN_POINT('Ctrl Pts',(9.47221976654,-38.0684833924,2.49225909299));
#67367=CARTESIAN_POINT('Ctrl Pts',(9.50381146403,-38.1627311721,2.51154069022));
#67368=CARTESIAN_POINT('Ctrl Pts',(9.56739722707,-38.2372245963,2.55034946501));
#67369=CARTESIAN_POINT('Ctrl Pts',(9.64784482414,-38.2742356128,2.59944964919));
#67370=CARTESIAN_POINT('Ctrl Pts',(9.72829242121,-38.2742356128,2.64854983337));
#67371=CARTESIAN_POINT('',(10.0571285787,-37.9742356128,0.645805825719));
#67372=CARTESIAN_POINT('Ctrl Pts',(9.47221976654,-37.9742356128,2.49225909299));
#67373=CARTESIAN_POINT('Ctrl Pts',(9.57333706543,-37.9742356128,2.32658468963));
#67374=CARTESIAN_POINT('Ctrl Pts',(9.67022825048,-37.9742356128,2.15028225121));
#67375=CARTESIAN_POINT('Ctrl Pts',(9.74871613381,-37.9742356128,1.96892463554));
#67376=CARTESIAN_POINT('Ctrl Pts',(9.87888878289,-37.9742356128,1.59411409567));
#67377=CARTESIAN_POINT('Ctrl Pts',(9.96252976109,-37.9742356128,1.2093437222));
#67378=CARTESIAN_POINT('Ctrl Pts',(9.99543705094,-37.9742356128,1.01939883766));
#67379=CARTESIAN_POINT('Ctrl Pts',(10.0275848223,-37.9742356128,0.834300487763));
#67380=CARTESIAN_POINT('Ctrl Pts',(10.0571285787,-37.9742356128,0.645805825719));
#67381=CARTESIAN_POINT('Origin',(10.3514120849986,-37.9763568300317,0.691946523729006));
#67382=CARTESIAN_POINT('Ctrl Pts',(9.47221976654,-37.9742356128,2.49225909299));
#67383=CARTESIAN_POINT('Ctrl Pts',(9.47221976654,-36.2942356128,2.49225909299));
#67384=CARTESIAN_POINT('Ctrl Pts',(9.53312961496,-37.9742356128,2.39246209578));
#67385=CARTESIAN_POINT('Ctrl Pts',(9.53312961496,-36.2942356128,2.39246209578));
#67386=CARTESIAN_POINT('Ctrl Pts',(9.59357915013,-37.9742356128,2.28708022821));
#67387=CARTESIAN_POINT('Ctrl Pts',(9.59357915013,-36.2942356128,2.28708022821));
#67388=CARTESIAN_POINT('Ctrl Pts',(9.64855478712,-37.9742356128,2.17984420246));
#67389=CARTESIAN_POINT('Ctrl Pts',(9.64855478712,-36.2942356128,2.17984420246));
#67390=CARTESIAN_POINT('Ctrl Pts',(9.7321123512,-37.9742356128,1.99616841131));
#67391=CARTESIAN_POINT('Ctrl Pts',(9.7321123512,-36.2942356128,1.99616841131));
#67392=CARTESIAN_POINT('Ctrl Pts',(9.80156823449,-37.9742356128,1.80635994999));
#67393=CARTESIAN_POINT('Ctrl Pts',(9.80156823449,-36.2942356128,1.80635994999));
#67394=CARTESIAN_POINT('Ctrl Pts',(9.82673775568,-37.9742356128,1.73070069002));
#67395=CARTESIAN_POINT('Ctrl Pts',(9.82673775568,-36.2942356128,1.73070069002));
#67396=CARTESIAN_POINT('Ctrl Pts',(9.90758702482,-37.9742356128,1.4638885651));
#67397=CARTESIAN_POINT('Ctrl Pts',(9.90758702482,-36.2942356128,1.4638885651));
#67398=CARTESIAN_POINT('Ctrl Pts',(9.9650475466,-37.9742356128,1.19577528243));
#67399=CARTESIAN_POINT('Ctrl Pts',(9.9650475466,-36.2942356128,1.19577528243));
#67400=CARTESIAN_POINT('Ctrl Pts',(9.9971133399,-37.9742356128,1.00951164249));
#67401=CARTESIAN_POINT('Ctrl Pts',(9.9971133399,-36.2942356128,1.00951164249));
#67402=CARTESIAN_POINT('Ctrl Pts',(10.0282717836,-37.9742356128,0.829917483849));
#67403=CARTESIAN_POINT('Ctrl Pts',(10.0282717836,-36.2942356128,0.829917483849));
#67404=CARTESIAN_POINT('Ctrl Pts',(10.0571285787,-37.9742356128,0.645805825719));
#67405=CARTESIAN_POINT('Ctrl Pts',(10.0571285787,-36.2942356128,0.645805825719));
#67406=CARTESIAN_POINT('',(10.0571285787,-37.2742356128,0.645805825719));
#67407=CARTESIAN_POINT('Ctrl Pts',(10.3535102065,-36.2742356128,0.692259352582));
#67408=CARTESIAN_POINT('Ctrl Pts',(10.2603991647,-36.2742356128,0.677665591985));
#67409=CARTESIAN_POINT('Ctrl Pts',(10.1672881228,-36.3112466293,0.663071831389));
#67410=CARTESIAN_POINT('Ctrl Pts',(10.0936931758,-36.3857400536,0.651536926221));
#67411=CARTESIAN_POINT('Ctrl Pts',(10.0571285552,-36.4799878332,0.645805969836));
#67412=CARTESIAN_POINT('Ctrl Pts',(10.0571285552,-36.5742356128,0.645805969836));
#67413=CARTESIAN_POINT('Ctrl Pts',(10.4654705253,-36.2742356128,-0.0220720388961));
#67414=CARTESIAN_POINT('Ctrl Pts',(10.3716407596,-36.2742356128,-0.0320801618586));
#67415=CARTESIAN_POINT('Ctrl Pts',(10.277810994,-36.3112466293,-0.042088284821));
#67416=CARTESIAN_POINT('Ctrl Pts',(10.2036479782,-36.3857400536,-0.0499987690501));
#67417=CARTESIAN_POINT('Ctrl Pts',(10.166801105,-36.4799878332,-0.0539288837071));
#67418=CARTESIAN_POINT('Ctrl Pts',(10.166801105,-36.5742356128,-0.0539288837071));
#67419=CARTESIAN_POINT('Ctrl Pts',(10.5332451587,-36.2742356128,-0.750280139625));
#67420=CARTESIAN_POINT('Ctrl Pts',(10.4390773883,-36.2742356128,-0.755397580353));
#67421=CARTESIAN_POINT('Ctrl Pts',(10.3449096179,-36.3112466293,-0.760515021082));
#67422=CARTESIAN_POINT('Ctrl Pts',(10.2704794173,-36.3857400536,-0.764559746152));
#67423=CARTESIAN_POINT('Ctrl Pts',(10.233499836,-36.4799878332,-0.766569459383));
#67424=CARTESIAN_POINT('Ctrl Pts',(10.233499836,-36.5742356128,-0.766569459383));
#67425=CARTESIAN_POINT('Ctrl Pts',(10.5621553524,-36.2742356128,-1.50355379103));
#67426=CARTESIAN_POINT('Ctrl Pts',(10.4669083702,-36.2742356128,-1.50048091028));
#67427=CARTESIAN_POINT('Ctrl Pts',(10.3716613881,-36.3112466293,-1.49740802953));
#67428=CARTESIAN_POINT('Ctrl Pts',(10.2963781981,-36.3857400536,-1.49497925029));
#67429=CARTESIAN_POINT('Ctrl Pts',(10.2589747918,-36.4799878332,-1.49377250781));
#67430=CARTESIAN_POINT('Ctrl Pts',(10.2589747918,-36.5742356128,-1.49377250781));
#67431=CARTESIAN_POINT('Ctrl Pts',(10.3656725489,-36.2742356128,-3.00545759266));
#67432=CARTESIAN_POINT('Ctrl Pts',(10.2732133718,-36.2742356128,-2.97798651849));
#67433=CARTESIAN_POINT('Ctrl Pts',(10.1807541948,-36.3112466293,-2.95051544432));
#67434=CARTESIAN_POINT('Ctrl Pts',(10.1076744778,-36.3857400536,-2.92880228958));
#67435=CARTESIAN_POINT('Ctrl Pts',(10.0713658476,-36.4799878332,-2.91801444773));
#67436=CARTESIAN_POINT('Ctrl Pts',(10.0713658476,-36.5742356128,-2.91801444773));
#67437=CARTESIAN_POINT('Ctrl Pts',(9.69612739523,-36.2742356128,-4.35866925271));
#67438=CARTESIAN_POINT('Ctrl Pts',(9.61531257083,-36.2742356128,-4.30797829153));
#67439=CARTESIAN_POINT('Ctrl Pts',(9.53449774643,-36.3112466293,-4.25728733035));
#67440=CARTESIAN_POINT('Ctrl Pts',(9.47062173065,-36.3857400536,-4.21722122832));
#67441=CARTESIAN_POINT('Ctrl Pts',(9.43888581966,-36.4799878332,-4.19731491187));
#67442=CARTESIAN_POINT('Ctrl Pts',(9.43888581966,-36.5742356128,-4.19731491187));
#67443=CARTESIAN_POINT('Ctrl Pts',(9.26520718698,-36.2742356128,-4.94839957983));
#67444=CARTESIAN_POINT('Ctrl Pts',(9.19061499526,-36.2742356128,-4.89024734488));
#67445=CARTESIAN_POINT('Ctrl Pts',(9.11602280354,-36.3112466293,-4.83209510993));
#67446=CARTESIAN_POINT('Ctrl Pts',(9.05706515172,-36.3857400536,-4.786131596));
#67447=CARTESIAN_POINT('Ctrl Pts',(9.02777286642,-36.4799878332,-4.76329526695));
#67448=CARTESIAN_POINT('Ctrl Pts',(9.02777286642,-36.5742356128,-4.76329526695));
#67449=CARTESIAN_POINT('Ctrl Pts',(8.51941071769,-36.2742356128,-5.80420810357));
#67450=CARTESIAN_POINT('Ctrl Pts',(8.45166351695,-36.2742356128,-5.73829733091));
#67451=CARTESIAN_POINT('Ctrl Pts',(8.38391631621,-36.3112466293,-5.67238655825));
#67452=CARTESIAN_POINT('Ctrl Pts',(8.33036894361,-36.3857400536,-5.62029069807));
#67453=CARTESIAN_POINT('Ctrl Pts',(8.30376468012,-36.4799878332,-5.59440759813));
#67454=CARTESIAN_POINT('Ctrl Pts',(8.30376468012,-36.5742356128,-5.59440759813));
#67455=CARTESIAN_POINT('Ctrl Pts',(7.6907047662,-36.2742356128,-6.55696420405));
#67456=CARTESIAN_POINT('Ctrl Pts',(7.62878309025,-36.2742356128,-6.48585146265));
#67457=CARTESIAN_POINT('Ctrl Pts',(7.5668614143,-36.3112466293,-6.41473872125));
#67458=CARTESIAN_POINT('Ctrl Pts',(7.51791853524,-36.3857400536,-6.3585312261));
#67459=CARTESIAN_POINT('Ctrl Pts',(7.49360194996,-36.4799878332,-6.33060531784));
#67460=CARTESIAN_POINT('Ctrl Pts',(7.49360194996,-36.5742356128,-6.33060531784));
#67461=CARTESIAN_POINT('Ctrl Pts',(7.38240736043,-36.2742356128,-6.81809919305));
#67462=CARTESIAN_POINT('Ctrl Pts',(7.32245884674,-36.2742356128,-6.74530491911));
#67463=CARTESIAN_POINT('Ctrl Pts',(7.26251033305,-36.3112466293,-6.67251064518));
#67464=CARTESIAN_POINT('Ctrl Pts',(7.21512704103,-36.3857400536,-6.61497406707));
#67465=CARTESIAN_POINT('Ctrl Pts',(7.19158531474,-36.4799878332,-6.58638782254));
#67466=CARTESIAN_POINT('Ctrl Pts',(7.19158531474,-36.5742356128,-6.58638782254));
#67467=CARTESIAN_POINT('Ctrl Pts',(6.75638043023,-36.2742356128,-7.31209369426));
#67468=CARTESIAN_POINT('Ctrl Pts',(6.70059555154,-36.2742356128,-7.23599823691));
#67469=CARTESIAN_POINT('Ctrl Pts',(6.64481067285,-36.3112466293,-7.15990277955));
#67470=CARTESIAN_POINT('Ctrl Pts',(6.60071831701,-36.3857400536,-7.09975694677));
#67471=CARTESIAN_POINT('Ctrl Pts',(6.57881164637,-36.4799878332,-7.06987433056));
#67472=CARTESIAN_POINT('Ctrl Pts',(6.57881164637,-36.5742356128,-7.06987433056));
#67473=CARTESIAN_POINT('Ctrl Pts',(6.0972721915,-36.2742356128,-7.7567769733));
#67474=CARTESIAN_POINT('Ctrl Pts',(6.04641537362,-36.2742356128,-7.67734201787));
#67475=CARTESIAN_POINT('Ctrl Pts',(5.99555855575,-36.3112466293,-7.59790706245));
#67476=CARTESIAN_POINT('Ctrl Pts',(5.95536133804,-36.3857400536,-7.53512169118));
#67477=CARTESIAN_POINT('Ctrl Pts',(5.9353899124,-36.4799878332,-7.5039276571));
#67478=CARTESIAN_POINT('Ctrl Pts',(5.9353899124,-36.5742356128,-7.5039276571));
#67479=CARTESIAN_POINT('Ctrl Pts',(5.75944878037,-36.2742356128,-7.96542127963));
#67480=CARTESIAN_POINT('Ctrl Pts',(5.71128828785,-36.2742356128,-7.88430555692));
#67481=CARTESIAN_POINT('Ctrl Pts',(5.66312779532,-36.3112466293,-7.80318983421));
#67482=CARTESIAN_POINT('Ctrl Pts',(5.62506175357,-36.3857400536,-7.73907598465));
#67483=CARTESIAN_POINT('Ctrl Pts',(5.60614917143,-36.4799878332,-7.70722191499));
#67484=CARTESIAN_POINT('Ctrl Pts',(5.60614917143,-36.5742356128,-7.70722191499));
#67485=CARTESIAN_POINT('Ctrl Pts',(4.87204527197,-36.2742356128,-8.46122850376));
#67486=CARTESIAN_POINT('Ctrl Pts',(4.83133074222,-36.2742356128,-8.37594391451));
#67487=CARTESIAN_POINT('Ctrl Pts',(4.79061621246,-36.3112466293,-8.29065932525));
#67488=CARTESIAN_POINT('Ctrl Pts',(4.75843545558,-36.3857400536,-8.22325040493));
#67489=CARTESIAN_POINT('Ctrl Pts',(4.74244689865,-36.4799878332,-8.18975922478));
#67490=CARTESIAN_POINT('Ctrl Pts',(4.74244689865,-36.5742356128,-8.18975922478));
#67491=CARTESIAN_POINT('Ctrl Pts',(3.93242931341,-36.2742356128,-8.85131842638));
#67492=CARTESIAN_POINT('Ctrl Pts',(3.90015750464,-36.2742356128,-8.76249452435));
#67493=CARTESIAN_POINT('Ctrl Pts',(3.86788569587,-36.3112466293,-8.67367062233));
#67494=CARTESIAN_POINT('Ctrl Pts',(3.8423780677,-36.3857400536,-8.60346422925));
#67495=CARTESIAN_POINT('Ctrl Pts',(3.82970495564,-36.4799878332,-8.56858316493));
#67496=CARTESIAN_POINT('Ctrl Pts',(3.82970495564,-36.5742356128,-8.56858316493));
#67497=CARTESIAN_POINT('Ctrl Pts',(3.34143335628,-36.2742356128,-9.04615827202));
#67498=CARTESIAN_POINT('Ctrl Pts',(3.31453785178,-36.2742356128,-8.95559501717));
#67499=CARTESIAN_POINT('Ctrl Pts',(3.28764234728,-36.3112466293,-8.86503176232));
#67500=CARTESIAN_POINT('Ctrl Pts',(3.26638413696,-36.3857400536,-8.79345058727));
#67501=CARTESIAN_POINT('Ctrl Pts',(3.25582230651,-36.4799878332,-8.75788647858));
#67502=CARTESIAN_POINT('Ctrl Pts',(3.25582230651,-36.5742356128,-8.75788647858));
#67503=CARTESIAN_POINT('Ctrl Pts',(2.73487315883,-36.2742356128,-9.19878073852));
#67504=CARTESIAN_POINT('Ctrl Pts',(2.71303985614,-36.2742356128,-9.10695943353));
#67505=CARTESIAN_POINT('Ctrl Pts',(2.69120655346,-36.3112466293,-9.01513812855));
#67506=CARTESIAN_POINT('Ctrl Pts',(2.67394952213,-36.3857400536,-8.94256258815));
#67507=CARTESIAN_POINT('Ctrl Pts',(2.66537559789,-36.4799878332,-8.90650444712));
#67508=CARTESIAN_POINT('Ctrl Pts',(2.66537559789,-36.5742356128,-8.90650444712));
#67509=CARTESIAN_POINT('Ctrl Pts',(2.11954062634,-36.2742356128,-9.3109005156));
#67510=CARTESIAN_POINT('Ctrl Pts',(2.10264593306,-36.2742356128,-9.21817935467));
#67511=CARTESIAN_POINT('Ctrl Pts',(2.08575123979,-36.3112466293,-9.12545819374));
#67512=CARTESIAN_POINT('Ctrl Pts',(2.07239767794,-36.3857400536,-9.05217140853));
#67513=CARTESIAN_POINT('Ctrl Pts',(2.0657631474,-36.4799878332,-9.01575989378));
#67514=CARTESIAN_POINT('Ctrl Pts',(2.0657631474,-36.5742356128,-9.01575989378));
#67515=CARTESIAN_POINT('',(2.06576130589928,-36.5742356128,-9.01576016580056));
#67516=CARTESIAN_POINT('Origin',(2.11916252104135,-36.5721144925218,-9.30881332409375));
#67517=CARTESIAN_POINT('Ctrl Pts',(10.05712857781,-36.5742356128,0.6458058255795));
#67518=CARTESIAN_POINT('Ctrl Pts',(10.0712039868866,-36.5742356128,0.556001631246168));
#67519=CARTESIAN_POINT('Ctrl Pts',(10.0844399589943,-36.5742356128,0.465906648280757));
#67520=CARTESIAN_POINT('Ctrl Pts',(10.096815487886,-36.5742356128,0.375515259159162));
#67521=CARTESIAN_POINT('Ctrl Pts',(10.1096992535075,-36.5742356128,0.281411687356653));
#67522=CARTESIAN_POINT('Ctrl Pts',(10.1216501586595,-36.5742356128,0.186986742025295));
#67523=CARTESIAN_POINT('Ctrl Pts',(10.1325881279532,-36.5742356128,0.0922479639907768));
#67524=CARTESIAN_POINT('Ctrl Pts',(10.1440788860828,-36.5742356128,-0.00727877215709816));
#67525=CARTESIAN_POINT('Ctrl Pts',(10.1544513400351,-36.5742356128,-0.107152044637042));
#67526=CARTESIAN_POINT('Ctrl Pts',(10.1635569310268,-36.5742356128,-0.207345680516345));
#67527=CARTESIAN_POINT('Ctrl Pts',(10.1737217027471,-36.5742356128,-0.319194042414421));
#67528=CARTESIAN_POINT('Ctrl Pts',(10.1823074911306,-36.5742356128,-0.431442176761078));
#67529=CARTESIAN_POINT('Ctrl Pts',(10.1890441337368,-36.5742356128,-0.544026357573112));
#67530=CARTESIAN_POINT('Ctrl Pts',(10.1952277414681,-36.5742356128,-0.647368103838791));
#67531=CARTESIAN_POINT('Ctrl Pts',(10.1998516599983,-36.5742356128,-0.750992719348358));
#67532=CARTESIAN_POINT('Ctrl Pts',(10.2026740714779,-36.5742356128,-0.854828666481071));
#67533=CARTESIAN_POINT('Ctrl Pts',(10.2048949078542,-36.5742356128,-0.936532787309225));
#67534=CARTESIAN_POINT('Ctrl Pts',(10.205999733603,-36.5742356128,-1.0183732282939));
#67535=CARTESIAN_POINT('Ctrl Pts',(10.205863143892,-36.5742356128,-1.10030594452211));
#67536=CARTESIAN_POINT('Ctrl Pts',(10.205657265768,-36.5742356128,-1.22380099984055));
#67537=CARTESIAN_POINT('Ctrl Pts',(10.2026292581837,-36.5742356128,-1.34750320034936));
#67538=CARTESIAN_POINT('Ctrl Pts',(10.1963512550468,-36.5742356128,-1.47120077077042));
#67539=CARTESIAN_POINT('Ctrl Pts',(10.1906356816034,-36.5742356128,-1.58381660308251));
#67540=CARTESIAN_POINT('Ctrl Pts',(10.1822248381961,-36.5742356128,-1.69642811272033));
#67541=CARTESIAN_POINT('Ctrl Pts',(10.1708230621608,-36.5742356128,-1.80884147526655));
#67542=CARTESIAN_POINT('Ctrl Pts',(10.1613744104428,-36.5742356128,-1.90199842799534));
#67543=CARTESIAN_POINT('Ctrl Pts',(10.1498715920879,-36.5742356128,-1.99501987510408));
#67544=CARTESIAN_POINT('Ctrl Pts',(10.1361734313148,-36.5742356128,-2.08777433560733));
#67545=CARTESIAN_POINT('Ctrl Pts',(10.1220621877022,-36.5742356128,-2.18332590709162));
#67546=CARTESIAN_POINT('Ctrl Pts',(10.1056205209072,-36.5742356128,-2.27859219750304));
#67547=CARTESIAN_POINT('Ctrl Pts',(10.0867343290288,-36.5742356128,-2.37341022121783));
#67548=CARTESIAN_POINT('Ctrl Pts',(10.0687364534174,-36.5742356128,-2.46376845794081));
#67549=CARTESIAN_POINT('Ctrl Pts',(10.0485182997365,-36.5742356128,-2.55371948411574));
#67550=CARTESIAN_POINT('Ctrl Pts',(10.0260250787213,-36.5742356128,-2.64310710082733));
#67551=CARTESIAN_POINT('Ctrl Pts',(10.0035318577062,-36.5742356128,-2.73249471753892));
#67552=CARTESIAN_POINT('Ctrl Pts',(9.97876296228436,-36.5742356128,-2.8213189237817));
#67553=CARTESIAN_POINT('Ctrl Pts',(9.95171582592092,-36.5742356128,-2.90940871914367));
#67554=CARTESIAN_POINT('Ctrl Pts',(9.92993931817063,-36.5742356128,-2.98033260866914));
#67555=CARTESIAN_POINT('Ctrl Pts',(9.90668774965613,-36.5742356128,-3.05077824731584));
#67556=CARTESIAN_POINT('Ctrl Pts',(9.88198479747963,-36.5742356128,-3.12067979234165));
#67557=CARTESIAN_POINT('Ctrl Pts',(9.86393211972182,-36.5742356128,-3.17176316319174));
#67558=CARTESIAN_POINT('Ctrl Pts',(9.84510545075928,-36.5742356128,-3.22255392981329));
#67559=CARTESIAN_POINT('Ctrl Pts',(9.82552203036848,-36.5742356128,-3.2730254094436));
#67560=CARTESIAN_POINT('Ctrl Pts',(9.78978496975496,-36.5742356128,-3.36512894860115));
#67561=CARTESIAN_POINT('Ctrl Pts',(9.75152280716754,-36.5742356128,-3.45617574805749));
#67562=CARTESIAN_POINT('Ctrl Pts',(9.7108497121987,-36.5742356128,-3.54609410175546));
#67563=CARTESIAN_POINT('Ctrl Pts',(9.6680049279269,-36.5742356128,-3.64081353407836));
#67564=CARTESIAN_POINT('Ctrl Pts',(9.62248519040241,-36.5742356128,-3.73428099545919));
#67565=CARTESIAN_POINT('Ctrl Pts',(9.57446091577429,-36.5742356128,-3.82645728198402));
#67566=CARTESIAN_POINT('Ctrl Pts',(9.52073520041125,-36.5742356128,-3.92957673503985));
#67567=CARTESIAN_POINT('Ctrl Pts',(9.4638752272999,-36.5742356128,-4.03108018727272));
#67568=CARTESIAN_POINT('Ctrl Pts',(9.4041607234943,-36.5742356128,-4.13096672981027));
#67569=CARTESIAN_POINT('Ctrl Pts',(9.3371221756021,-36.5742356128,-4.24310445748008));
#67570=CARTESIAN_POINT('Ctrl Pts',(9.2664869431227,-36.5742356128,-4.35320477522716));
#67571=CARTESIAN_POINT('Ctrl Pts',(9.19268999051769,-36.5742356128,-4.46132811226467));
#67572=CARTESIAN_POINT('Ctrl Pts',(9.13418828270235,-36.5742356128,-4.54704167695946));
#67573=CARTESIAN_POINT('Ctrl Pts',(9.07370082500083,-36.5742356128,-4.6315144538525));
#67574=CARTESIAN_POINT('Ctrl Pts',(9.01145050633955,-36.5742356128,-4.71479444137142));
#67575=CARTESIAN_POINT('Ctrl Pts',(8.9668168326544,-36.5742356128,-4.7745064535725));
#67576=CARTESIAN_POINT('Ctrl Pts',(8.92128231296221,-36.5742356128,-4.83359844391629));
#67577=CARTESIAN_POINT('Ctrl Pts',(8.87493145664548,-36.5742356128,-4.89208723168315));
#67578=CARTESIAN_POINT('Ctrl Pts',(8.79441053195804,-36.5742356128,-4.99369422773634));
#67579=CARTESIAN_POINT('Ctrl Pts',(8.71142780300561,-36.5742356128,-5.09348285810377));
#67580=CARTESIAN_POINT('Ctrl Pts',(8.6263979916159,-36.5742356128,-5.19154646335235));
#67581=CARTESIAN_POINT('Ctrl Pts',(8.54993426376687,-36.5742356128,-5.2797309330233));
#67582=CARTESIAN_POINT('Ctrl Pts',(8.47181575924716,-36.5742356128,-5.36652132950478));
#67583=CARTESIAN_POINT('Ctrl Pts',(8.39230621820942,-36.5742356128,-5.45196981180327));
#67584=CARTESIAN_POINT('Ctrl Pts',(8.31988794127727,-36.5742356128,-5.52979735015603));
#67585=CARTESIAN_POINT('Ctrl Pts',(8.24631587368035,-36.5742356128,-5.60651203021272));
#67586=CARTESIAN_POINT('Ctrl Pts',(8.17175117079795,-36.5742356128,-5.68213159754941));
#67587=CARTESIAN_POINT('Ctrl Pts',(8.13847955968082,-36.5742356128,-5.71587390107927));
#67588=CARTESIAN_POINT('Ctrl Pts',(8.10500975983473,-36.5742356128,-5.74939782796711));
#67589=CARTESIAN_POINT('Ctrl Pts',(8.07135317616891,-36.5742356128,-5.78270311230429));
#67590=CARTESIAN_POINT('Ctrl Pts',(7.98726197733494,-36.5742356128,-5.86591658742194));
#67591=CARTESIAN_POINT('Ctrl Pts',(7.90200681957206,-36.5742356128,-5.94776768512651));
#67592=CARTESIAN_POINT('Ctrl Pts',(7.81579962946374,-36.5742356128,-6.02827359551016));
#67593=CARTESIAN_POINT('Ctrl Pts',(7.7303665176099,-36.5742356128,-6.10805662101023));
#67594=CARTESIAN_POINT('Ctrl Pts',(7.64399912169157,-36.5742356128,-6.18651730248495));
#67595=CARTESIAN_POINT('Ctrl Pts',(7.5568608474066,-36.5742356128,-6.26364586505813));
#67596=CARTESIAN_POINT('Ctrl Pts',(7.47440298385371,-36.5742356128,-6.3366316631001));
#67597=CARTESIAN_POINT('Ctrl Pts',(7.39125503861802,-36.5742356128,-6.40842359127944));
#67598=CARTESIAN_POINT('Ctrl Pts',(7.30751084820958,-36.5742356128,-6.47900555413623));
#67599=CARTESIAN_POINT('Ctrl Pts',(7.23643171398355,-36.5742356128,-6.53891305085173));
#67600=CARTESIAN_POINT('Ctrl Pts',(7.16492249745893,-36.5742356128,-6.59794848505397));
#67601=CARTESIAN_POINT('Ctrl Pts',(7.09301131809069,-36.5742356128,-6.65610476540732));
#67602=CARTESIAN_POINT('Ctrl Pts',(7.007007109353,-36.5742356128,-6.72565841365588));
#67603=CARTESIAN_POINT('Ctrl Pts',(6.92043185960323,-36.5742356128,-6.79395229394742));
#67604=CARTESIAN_POINT('Ctrl Pts',(6.83324562170684,-36.5742356128,-6.86101265125115));
#67605=CARTESIAN_POINT('Ctrl Pts',(6.75618323322322,-36.5742356128,-6.92028612641282));
#67606=CARTESIAN_POINT('Ctrl Pts',(6.67864568902824,-36.5742356128,-6.97859342329466));
#67607=CARTESIAN_POINT('Ctrl Pts',(6.60056822518713,-36.5742356128,-7.03596299746881));
#67608=CARTESIAN_POINT('Ctrl Pts',(6.59031102317183,-36.5742356128,-7.04349976010027));
#67609=CARTESIAN_POINT('Ctrl Pts',(6.58004443577428,-36.5742356128,-7.05102037001382));
#67610=CARTESIAN_POINT('Ctrl Pts',(6.56976825429465,-36.5742356128,-7.05852492132114));
#67611=CARTESIAN_POINT('Ctrl Pts',(6.45579354456556,-36.5742356128,-7.14175905440781));
#67612=CARTESIAN_POINT('Ctrl Pts',(6.34063476844058,-36.5742356128,-7.22302068405111));
#67613=CARTESIAN_POINT('Ctrl Pts',(6.22422868607061,-36.5742356128,-7.30221428504094));
#67614=CARTESIAN_POINT('Ctrl Pts',(6.13966758898243,-36.5742356128,-7.359743046818));
#67615=CARTESIAN_POINT('Ctrl Pts',(6.05444938322057,-36.5742356128,-7.4161795741547));
#67616=CARTESIAN_POINT('Ctrl Pts',(5.96856201827064,-36.5742356128,-7.47147912409491));
#67617=CARTESIAN_POINT('Ctrl Pts',(5.88578700122719,-36.5742356128,-7.52477475368448));
#67618=CARTESIAN_POINT('Ctrl Pts',(5.80238971411301,-36.5742356128,-7.57701442935241));
#67619=CARTESIAN_POINT('Ctrl Pts',(5.71838751084297,-36.5742356128,-7.62814299484061));
#67620=CARTESIAN_POINT('Ctrl Pts',(5.57771899649851,-36.5742356128,-7.71376193181858));
#67621=CARTESIAN_POINT('Ctrl Pts',(5.43534417855391,-36.5742356128,-7.79626894567029));
#67622=CARTESIAN_POINT('Ctrl Pts',(5.29130214602209,-36.5742356128,-7.87546190675721));
#67623=CARTESIAN_POINT('Ctrl Pts',(5.17031042933696,-36.5742356128,-7.94198201996909));
#67624=CARTESIAN_POINT('Ctrl Pts',(5.04814359116801,-36.5742356128,-8.00616326407657));
#67625=CARTESIAN_POINT('Ctrl Pts',(4.92482519220396,-36.5742356128,-8.06791498370429));
#67626=CARTESIAN_POINT('Ctrl Pts',(4.77828868798353,-36.5742356128,-8.14129317544099));
#67627=CARTESIAN_POINT('Ctrl Pts',(4.63012513822672,-36.5742356128,-8.21124076793695));
#67628=CARTESIAN_POINT('Ctrl Pts',(4.48037267031824,-36.5742356128,-8.27765035657664));
#67629=CARTESIAN_POINT('Ctrl Pts',(4.32793376944481,-36.5742356128,-8.34525127722308));
#67630=CARTESIAN_POINT('Ctrl Pts',(4.17384721339769,-36.5742356128,-8.40918661356067));
#67631=CARTESIAN_POINT('Ctrl Pts',(4.01816442281152,-36.5742356128,-8.46939577180371));
#67632=CARTESIAN_POINT('Ctrl Pts',(3.86134597137964,-36.5742356128,-8.53004413840955));
#67633=CARTESIAN_POINT('Ctrl Pts',(3.70290662104831,-36.5742356128,-8.58691239389757));
#67634=CARTESIAN_POINT('Ctrl Pts',(3.54292923213171,-36.5742356128,-8.6399829259404));
#67635=CARTESIAN_POINT('Ctrl Pts',(3.3938750351181,-36.5742356128,-8.68942982335697));
#67636=CARTESIAN_POINT('Ctrl Pts',(3.24348513062699,-36.5742356128,-8.73558077178669));
#67637=CARTESIAN_POINT('Ctrl Pts',(3.09186488177117,-36.5742356128,-8.77844839317499));
#67638=CARTESIAN_POINT('Ctrl Pts',(2.94558178293629,-36.5742356128,-8.81980704113714));
#67639=CARTESIAN_POINT('Ctrl Pts',(2.79815290474148,-36.5742356128,-8.85810997089225));
#67640=CARTESIAN_POINT('Ctrl Pts',(2.64971757941682,-36.5742356128,-8.89338492401371));
#67641=CARTESIAN_POINT('Ctrl Pts',(2.50830664355868,-36.5742356128,-8.92699056419637));
#67642=CARTESIAN_POINT('Ctrl Pts',(2.3659820008866,-36.5742356128,-8.95784844431244));
#67643=CARTESIAN_POINT('Ctrl Pts',(2.22291081731417,-36.5742356128,-8.9859910514163));
#67644=CARTESIAN_POINT('Ctrl Pts',(2.17062417406695,-36.5742356128,-8.99627601880766));
#67645=CARTESIAN_POINT('Ctrl Pts',(2.11823830832693,-36.5742356128,-9.00619838927665));
#67646=CARTESIAN_POINT('Ctrl Pts',(2.0657631474,-36.5742356128,-9.01575989378));
#67647=CARTESIAN_POINT('Ctrl Pts',(2.06575925082,-37.9742356128,-9.01576051427));
#67648=CARTESIAN_POINT('Ctrl Pts',(2.06575925243,-38.0684833925,-9.01576051398));
#67649=CARTESIAN_POINT('Ctrl Pts',(2.07239387846,-38.1627311721,-9.0521720105));
#67650=CARTESIAN_POINT('Ctrl Pts',(2.08574763055,-38.2372245964,-9.12545875939));
#67651=CARTESIAN_POINT('Ctrl Pts',(2.10264256354,-38.2742356129,-9.21817987454));
#67652=CARTESIAN_POINT('Ctrl Pts',(2.11953749589,-38.2742356128,-9.31090098978));
#67653=CARTESIAN_POINT('Ctrl Pts',(2.55230448535,-37.9742356128,-8.92710614538));
#67654=CARTESIAN_POINT('Ctrl Pts',(2.55230457983,-38.0684833936,-8.92710612828));
#67655=CARTESIAN_POINT('Ctrl Pts',(2.56051293846,-38.1627311744,-8.96323086957));
#67656=CARTESIAN_POINT('Ctrl Pts',(2.57703406707,-38.2372245991,-9.0359404797));
#67657=CARTESIAN_POINT('Ctrl Pts',(2.59793626097,-38.2742356147,-9.12793141729));
#67658=CARTESIAN_POINT('Ctrl Pts',(2.61883841766,-38.2742356128,-9.21992236087));
#67659=CARTESIAN_POINT('Ctrl Pts',(3.03294472376,-37.9742356128,-8.81251059078));
#67660=CARTESIAN_POINT('Ctrl Pts',(3.03294455621,-38.0684833844,-8.81251062117));
#67661=CARTESIAN_POINT('Ctrl Pts',(3.04275300679,-38.1627311559,-8.84825697631));
#67662=CARTESIAN_POINT('Ctrl Pts',(3.06249506668,-38.2372245773,-8.92020492813));
#67663=CARTESIAN_POINT('Ctrl Pts',(3.08747246677,-38.2742356002,-9.01123220726));
#67664=CARTESIAN_POINT('Ctrl Pts',(3.11244993377,-38.2742356128,-9.1022594793));
#67665=CARTESIAN_POINT('Ctrl Pts',(3.50352252846,-37.9742356128,-8.67141257711));
#67666=CARTESIAN_POINT('Ctrl Pts',(3.50352256012,-38.0684833947,-8.67141257232));
#67667=CARTESIAN_POINT('Ctrl Pts',(3.51501818843,-38.1627311765,-8.70666289898));
#67668=CARTESIAN_POINT('Ctrl Pts',(3.5381558134,-38.2372246016,-8.7776125257));
#67669=CARTESIAN_POINT('Ctrl Pts',(3.56742911598,-38.2742356164,-8.86737675603));
#67670=CARTESIAN_POINT('Ctrl Pts',(3.59670240576,-38.2742356128,-8.95714098692));
#67671=CARTESIAN_POINT('Ctrl Pts',(4.58730752681,-37.9742356128,-8.27387012043));
#67672=CARTESIAN_POINT('Ctrl Pts',(4.58730748381,-38.0684833894,-8.27387012693));
#67673=CARTESIAN_POINT('Ctrl Pts',(4.60272266161,-38.162731166,-8.30767434705));
#67674=CARTESIAN_POINT('Ctrl Pts',(4.63374941501,-38.2372245892,-8.37571332545));
#67675=CARTESIAN_POINT('Ctrl Pts',(4.67300394407,-38.2742356081,-8.46179505077));
#67676=CARTESIAN_POINT('Ctrl Pts',(4.71225849052,-38.2742356128,-8.54787677533));
#67677=CARTESIAN_POINT('Ctrl Pts',(5.60638547087,-37.9742356128,-7.7308046141));
#67678=CARTESIAN_POINT('Ctrl Pts',(5.60638552928,-38.0684833966,-7.73080460527));
#67679=CARTESIAN_POINT('Ctrl Pts',(5.62536773699,-38.1627311803,-7.76270770883));
#67680=CARTESIAN_POINT('Ctrl Pts',(5.66357383517,-38.2372246061,-7.82692026332));
#67681=CARTESIAN_POINT('Ctrl Pts',(5.71191149292,-38.2742356193,-7.90816086883));
#67682=CARTESIAN_POINT('Ctrl Pts',(5.76024912705,-38.2742356128,-7.98940147537));
#67683=CARTESIAN_POINT('Ctrl Pts',(6.16964163718,-37.9742356128,-7.37017137729));
#67684=CARTESIAN_POINT('Ctrl Pts',(6.16964161946,-38.0684833871,-7.37017139274));
#67685=CARTESIAN_POINT('Ctrl Pts',(6.1904385669,-38.1627311614,-7.40086532392));
#67686=CARTESIAN_POINT('Ctrl Pts',(6.23229736424,-38.2372245838,-7.46264410061));
#67687=CARTESIAN_POINT('Ctrl Pts',(6.28525639509,-38.2742356045,-7.54080552318));
#67688=CARTESIAN_POINT('Ctrl Pts',(6.33821543401,-38.2742356128,-7.61896694326));
#67689=CARTESIAN_POINT('Ctrl Pts',(7.09776508839,-37.9742356128,-6.69246789154));
#67690=CARTESIAN_POINT('Ctrl Pts',(7.0977651012,-38.0684833963,-6.69246788036));
#67691=CARTESIAN_POINT('Ctrl Pts',(7.12103415187,-38.1627311798,-6.72135650201));
#67692=CARTESIAN_POINT('Ctrl Pts',(7.16786860412,-38.2372246054,-6.77950169941));
#67693=CARTESIAN_POINT('Ctrl Pts',(7.227122727,-38.2742356189,-6.85306599289));
#67694=CARTESIAN_POINT('Ctrl Pts',(7.28637684404,-38.2742356128,-6.92663028817));
#67695=CARTESIAN_POINT('Ctrl Pts',(7.97017602494,-37.9742356128,-5.90158416283));
#67696=CARTESIAN_POINT('Ctrl Pts',(7.97017601568,-38.0684833897,-5.9015841709));
#67697=CARTESIAN_POINT('Ctrl Pts',(7.99582514165,-38.1627311665,-5.92831961073));
#67698=CARTESIAN_POINT('Ctrl Pts',(8.04745008519,-38.2372245898,-5.98213099676));
#67699=CARTESIAN_POINT('Ctrl Pts',(8.11276506833,-38.2742356085,-6.05021221902));
#67700=CARTESIAN_POINT('Ctrl Pts',(8.17808005568,-38.2742356128,-6.11829343998));
#67701=CARTESIAN_POINT('Ctrl Pts',(8.32234138636,-37.9742356128,-5.5511354177));
#67702=CARTESIAN_POINT('Ctrl Pts',(8.322341377,-38.0684833626,-5.55113542953));
#67703=CARTESIAN_POINT('Ctrl Pts',(8.34905084971,-38.1627311123,-5.57683611657));
#67704=CARTESIAN_POINT('Ctrl Pts',(8.40280999154,-38.237224526,-5.62856481282));
#67705=CARTESIAN_POINT('Ctrl Pts',(8.47082513402,-38.2742355659,-5.69401105676));
#67706=CARTESIAN_POINT('Ctrl Pts',(8.5388402942,-38.2742356128,-5.759457308));
#67707=CARTESIAN_POINT('Ctrl Pts',(8.90931541395,-37.9742356128,-4.89736181467));
#67708=CARTESIAN_POINT('Ctrl Pts',(8.90931542119,-38.0684834156,-4.89736180551));
#67709=CARTESIAN_POINT('Ctrl Pts',(8.93825785475,-38.1627312183,-4.92066469564));
#67710=CARTESIAN_POINT('Ctrl Pts',(8.99651133904,-38.2372246508,-4.9675672848));
#67711=CARTESIAN_POINT('Ctrl Pts',(9.07021261859,-38.2742356492,-5.02690762115));
#67712=CARTESIAN_POINT('Ctrl Pts',(9.14391388443,-38.2742356128,-5.08624795184));
#67713=CARTESIAN_POINT('Ctrl Pts',(9.39879152195,-37.9742356128,-4.17295757679));
#67714=CARTESIAN_POINT('Ctrl Pts',(9.39879151634,-38.0684833745,-4.17295758389));
#67715=CARTESIAN_POINT('Ctrl Pts',(9.4304078184,-38.1627311363,-4.19237724524));
#67716=CARTESIAN_POINT('Ctrl Pts',(9.49404311057,-38.2372245542,-4.23146389807));
#67717=CARTESIAN_POINT('Ctrl Pts',(9.57455337996,-38.2742355847,-4.28091564899));
#67718=CARTESIAN_POINT('Ctrl Pts',(9.65506365997,-38.2742356128,-4.33036740429));
#67719=CARTESIAN_POINT('Ctrl Pts',(9.58754232636,-37.9742356128,-3.84345571161));
#67720=CARTESIAN_POINT('Ctrl Pts',(9.58754233174,-38.0684833927,-3.84345574942));
#67721=CARTESIAN_POINT('Ctrl Pts',(9.62040667626,-38.1627311725,-3.86074836295));
#67722=CARTESIAN_POINT('Ctrl Pts',(9.68655393532,-38.2372245968,-3.89555378883));
#67723=CARTESIAN_POINT('Ctrl Pts',(9.77024228936,-38.2742356132,-3.93958898382));
#67724=CARTESIAN_POINT('Ctrl Pts',(9.85393064124,-38.2742356128,-3.98362416376));
#67725=CARTESIAN_POINT('Ctrl Pts',(10.0701345637,-37.9742356128,-2.79823040916));
#67726=CARTESIAN_POINT('Ctrl Pts',(10.0701345528,-38.068483392,-2.79823033248));
#67727=CARTESIAN_POINT('Ctrl Pts',(10.1063202118,-38.1627311712,-2.80841507563));
#67728=CARTESIAN_POINT('Ctrl Pts',(10.1791524231,-38.2372245954,-2.82891437946));
#67729=CARTESIAN_POINT('Ctrl Pts',(10.2712984713,-38.2742356122,-2.85484978525));
#67730=CARTESIAN_POINT('Ctrl Pts',(10.363444524,-38.2742356128,-2.88078522158));
#67731=CARTESIAN_POINT('Ctrl Pts',(10.2631011081,-37.9742356128,-1.6439245767));
#67732=CARTESIAN_POINT('Ctrl Pts',(10.2631011302,-38.0684833933,-1.64392473221));
#67733=CARTESIAN_POINT('Ctrl Pts',(10.300671344,-38.1627311737,-1.6458337115));
#67734=CARTESIAN_POINT('Ctrl Pts',(10.3762902569,-38.2372245983,-1.64967578111));
#67735=CARTESIAN_POINT('Ctrl Pts',(10.471961972,-38.2742356142,-1.65453661061));
#67736=CARTESIAN_POINT('Ctrl Pts',(10.5676336782,-38.2742356128,-1.6593973782));
#67737=CARTESIAN_POINT('Ctrl Pts',(10.2421633997,-37.9742356128,-0.862745648495));
#67738=CARTESIAN_POINT('Ctrl Pts',(10.2421633045,-38.0684833989,-0.862745049409));
#67739=CARTESIAN_POINT('Ctrl Pts',(10.2791438065,-38.1627311851,-0.860933872727));
#67740=CARTESIAN_POINT('Ctrl Pts',(10.3535759371,-38.2372246117,-0.857289229083));
#67741=CARTESIAN_POINT('Ctrl Pts',(10.4477462212,-38.2742356231,-0.852678435106));
#67742=CARTESIAN_POINT('Ctrl Pts',(10.5419165386,-38.2742356128,-0.848067876398));
#67743=CARTESIAN_POINT('Ctrl Pts',(10.1742417982,-37.9742356128,-0.101398893364));
#67744=CARTESIAN_POINT('Ctrl Pts',(10.1742418626,-38.068483393,-0.101399296931));
#67745=CARTESIAN_POINT('Ctrl Pts',(10.2111107023,-38.1627311731,-0.0976092671479));
#67746=CARTESIAN_POINT('Ctrl Pts',(10.2853178786,-38.2372245976,-0.0899804119975));
#67747=CARTESIAN_POINT('Ctrl Pts',(10.3792034651,-38.2742356137,-0.0803282850477));
#67748=CARTESIAN_POINT('Ctrl Pts',(10.473089026,-38.2742356128,-0.0706759998837));
#67749=CARTESIAN_POINT('Ctrl Pts',(10.0571290687,-37.9742356128,0.645802815386));
#67750=CARTESIAN_POINT('Ctrl Pts',(10.057129068,-38.0684833924,0.645802819843));
#67751=CARTESIAN_POINT('Ctrl Pts',(10.0936936567,-38.162731172,0.651533980199));
#67752=CARTESIAN_POINT('Ctrl Pts',(10.1672885404,-38.2372245963,0.663069290459));
#67753=CARTESIAN_POINT('Ctrl Pts',(10.2603995024,-38.2742356128,0.677663560866));
#67754=CARTESIAN_POINT('Ctrl Pts',(10.3535104648,-38.2742356128,0.692257829523));
#67755=CARTESIAN_POINT('',(2.06575948168,-37.9742356128,-9.01576047707));
#67756=CARTESIAN_POINT('Ctrl Pts',(10.0571285787,-37.9742356128,0.645805825719));
#67757=CARTESIAN_POINT('Ctrl Pts',(10.1742417982,-37.9742356128081,-0.101398893364));
#67758=CARTESIAN_POINT('Ctrl Pts',(10.2421633997,-37.9742356128081,-0.862745648495));
#67759=CARTESIAN_POINT('Ctrl Pts',(10.2631011081,-37.9742356128081,-1.6439245767));
#67760=CARTESIAN_POINT('Ctrl Pts',(10.0701345637,-37.9742356128081,-2.79823040916));
#67761=CARTESIAN_POINT('Ctrl Pts',(9.58754232635999,-37.9742356128081,-3.84345571161));
#67762=CARTESIAN_POINT('Ctrl Pts',(9.39879152195,-37.9742356128081,-4.17295757679));
#67763=CARTESIAN_POINT('Ctrl Pts',(8.90931541394999,-37.9742356128081,-4.89736181467));
#67764=CARTESIAN_POINT('Ctrl Pts',(8.32234138636,-37.9742356128081,-5.5511354177));
#67765=CARTESIAN_POINT('Ctrl Pts',(7.97017602494,-37.9742356128081,-5.90158416283));
#67766=CARTESIAN_POINT('Ctrl Pts',(7.09776508839,-37.9742356128081,-6.69246789154));
#67767=CARTESIAN_POINT('Ctrl Pts',(6.16964163718,-37.9742356128081,-7.37017137729));
#67768=CARTESIAN_POINT('Ctrl Pts',(5.60638547087,-37.9742356128081,-7.7308046141));
#67769=CARTESIAN_POINT('Ctrl Pts',(4.58730752681,-37.9742356128081,-8.27387012042999));
#67770=CARTESIAN_POINT('Ctrl Pts',(3.50352252846,-37.9742356128081,-8.67141257711));
#67771=CARTESIAN_POINT('Ctrl Pts',(3.03294472376,-37.9742356128081,-8.81251059078));
#67772=CARTESIAN_POINT('Ctrl Pts',(2.55230448535,-37.9742356128081,-8.92710614538));
#67773=CARTESIAN_POINT('Ctrl Pts',(2.06575948168,-37.9742356128,-9.01576047707));
#67774=CARTESIAN_POINT('Origin',(2.11915744553878,-37.9763569133101,-9.30881401396193));
#67775=CARTESIAN_POINT('Ctrl Pts',(10.0571285787,-37.9742356128,0.645805825719));
#67776=CARTESIAN_POINT('Ctrl Pts',(10.0571285787,-36.2942356128,0.645805825719));
#67777=CARTESIAN_POINT('Ctrl Pts',(10.1043144812,-37.9742356128,0.34475109394));
#67778=CARTESIAN_POINT('Ctrl Pts',(10.1043144812,-36.2942356128,0.34475109394));
#67779=CARTESIAN_POINT('Ctrl Pts',(10.1436911823,-37.9742356128,0.0415756247073));
#67780=CARTESIAN_POINT('Ctrl Pts',(10.1436911823,-36.2942356128,0.0415756247073));
#67781=CARTESIAN_POINT('Ctrl Pts',(10.1751569467,-37.9742356128,-0.265526349591));
#67782=CARTESIAN_POINT('Ctrl Pts',(10.1751569467,-36.2942356128,-0.265526349591));
#67783=CARTESIAN_POINT('Ctrl Pts',(10.2113958308,-37.9742356128,-0.803196289146));
#67784=CARTESIAN_POINT('Ctrl Pts',(10.2113958308,-36.2942356128,-0.803196289146));
#67785=CARTESIAN_POINT('Ctrl Pts',(10.2066163947,-37.9742356128,-1.34483444271));
#67786=CARTESIAN_POINT('Ctrl Pts',(10.2066163947,-36.2942356128,-1.34483444271));
#67787=CARTESIAN_POINT('Ctrl Pts',(10.1959693719,-37.9742356128,-1.57549366978));
#67788=CARTESIAN_POINT('Ctrl Pts',(10.1959693719,-36.2942356128,-1.57549366978));
#67789=CARTESIAN_POINT('Ctrl Pts',(10.154755688,-37.9742356128,-2.03576280703));
#67790=CARTESIAN_POINT('Ctrl Pts',(10.154755688,-36.2942356128,-2.03576280703));
#67791=CARTESIAN_POINT('Ctrl Pts',(10.0694270848,-37.9742356128,-2.49123410794));
#67792=CARTESIAN_POINT('Ctrl Pts',(10.0694270848,-36.2942356128,-2.49123410794));
#67793=CARTESIAN_POINT('Ctrl Pts',(10.0147288892,-37.9742356128,-2.71679407199));
#67794=CARTESIAN_POINT('Ctrl Pts',(10.0147288892,-36.2942356128,-2.71679407199));
#67795=CARTESIAN_POINT('Ctrl Pts',(9.84427307953,-37.9742356128,-3.28258152506));
#67796=CARTESIAN_POINT('Ctrl Pts',(9.84427307953,-36.2942356128,-3.28258152506));
#67797=CARTESIAN_POINT('Ctrl Pts',(9.59767693443,-37.9742356128,-3.81973064429));
#67798=CARTESIAN_POINT('Ctrl Pts',(9.59767693443,-36.2942356128,-3.81973064429));
#67799=CARTESIAN_POINT('Ctrl Pts',(9.42196991538,-37.9742356128,-4.13127436125));
#67800=CARTESIAN_POINT('Ctrl Pts',(9.42196991538,-36.2942356128,-4.13127436125));
#67801=CARTESIAN_POINT('Ctrl Pts',(8.90941365275,-37.9742356128,-4.9063140586));
#67802=CARTESIAN_POINT('Ctrl Pts',(8.90941365275,-36.2942356128,-4.9063140586));
#67803=CARTESIAN_POINT('Ctrl Pts',(8.28331893235,-37.9742356128,-5.59939000154));
#67804=CARTESIAN_POINT('Ctrl Pts',(8.28331893235,-36.2942356128,-5.59939000154));
#67805=CARTESIAN_POINT('Ctrl Pts',(7.87223833419,-37.9742356128,-6.00004951346));
#67806=CARTESIAN_POINT('Ctrl Pts',(7.87223833419,-36.2942356128,-6.00004951346));
#67807=CARTESIAN_POINT('Ctrl Pts',(7.23577044162,-37.9742356128,-6.56118503753));
#67808=CARTESIAN_POINT('Ctrl Pts',(7.23577044162,-36.2942356128,-6.56118503753));
#67809=CARTESIAN_POINT('Ctrl Pts',(6.57301164306,-37.9742356128,-7.06148474596));
#67810=CARTESIAN_POINT('Ctrl Pts',(6.57301164306,-36.2942356128,-7.06148474596));
#67811=CARTESIAN_POINT('Ctrl Pts',(6.34892734606,-37.9742356128,-7.22182745263));
#67812=CARTESIAN_POINT('Ctrl Pts',(6.34892734606,-36.2942356128,-7.22182745263));
#67813=CARTESIAN_POINT('Ctrl Pts',(5.43475192661,-37.9742356128,-7.8381799988));
#67814=CARTESIAN_POINT('Ctrl Pts',(5.43475192661,-36.2942356128,-7.8381799988));
#67815=CARTESIAN_POINT('Ctrl Pts',(4.45617471097,-37.9742356128,-8.34265749719));
#67816=CARTESIAN_POINT('Ctrl Pts',(4.45617471097,-36.2942356128,-8.34265749719));
#67817=CARTESIAN_POINT('Ctrl Pts',(3.69023581936,-37.9742356128,-8.64282630111));
#67818=CARTESIAN_POINT('Ctrl Pts',(3.69023581936,-36.2942356128,-8.64282630111));
#67819=CARTESIAN_POINT('Ctrl Pts',(2.88684751199,-37.9742356128,-8.86614972783));
#67820=CARTESIAN_POINT('Ctrl Pts',(2.88684751199,-36.2942356128,-8.86614972783));
#67821=CARTESIAN_POINT('Ctrl Pts',(2.06575948168,-37.9742356128,-9.01576047707));
#67822=CARTESIAN_POINT('Ctrl Pts',(2.06575948168,-36.2942356128,-9.01576047707));
#67823=CARTESIAN_POINT('',(2.06575948168,-37.2742356128,-9.01576047707));
#67824=CARTESIAN_POINT('Ctrl Pts',(2.11953715431,-36.2742356128,-9.31090105701));
#67825=CARTESIAN_POINT('Ctrl Pts',(2.10264240018,-36.2742356128,-9.21817990924));
#67826=CARTESIAN_POINT('Ctrl Pts',(2.08574764605,-36.3112466293,-9.12545876147));
#67827=CARTESIAN_POINT('Ctrl Pts',(2.07239403611,-36.3857400536,-9.05217198666));
#67828=CARTESIAN_POINT('Ctrl Pts',(2.06575948168,-36.4799878332,-9.01576047707));
#67829=CARTESIAN_POINT('Ctrl Pts',(2.06575948168,-36.5742356128,-9.01576047707));
#67830=CARTESIAN_POINT('Ctrl Pts',(2.11615383992,-36.2742356128,-9.31151753196));
#67831=CARTESIAN_POINT('Ctrl Pts',(2.09914098406,-36.2742356128,-9.21881790355));
#67832=CARTESIAN_POINT('Ctrl Pts',(2.08212812821,-36.3112466293,-9.12611827514));
#67833=CARTESIAN_POINT('Ctrl Pts',(2.06868117069,-36.3857400536,-9.05284850922));
#67834=CARTESIAN_POINT('Ctrl Pts',(2.06200023781,-36.4799878332,-9.01644545027));
#67835=CARTESIAN_POINT('Ctrl Pts',(2.06200023781,-36.5742356128,-9.01644545027));
#67836=CARTESIAN_POINT('Ctrl Pts',(2.11277150501,-36.2742356128,-9.31213939407));
#67837=CARTESIAN_POINT('Ctrl Pts',(2.09564058293,-36.2742356128,-9.21946147283));
#67838=CARTESIAN_POINT('Ctrl Pts',(2.07850966085,-36.3112466293,-9.12678355158));
#67839=CARTESIAN_POINT('Ctrl Pts',(2.0649693838,-36.3857400536,-9.05353094301));
#67840=CARTESIAN_POINT('Ctrl Pts',(2.05824208644,-36.4799878332,-9.01713640844));
#67841=CARTESIAN_POINT('Ctrl Pts',(2.05824208644,-36.5742356128,-9.01713640844));
#67842=CARTESIAN_POINT('Ctrl Pts',(2.10940495264,-36.2742356128,-9.31276374494));
#67843=CARTESIAN_POINT('Ctrl Pts',(2.09215498197,-36.2742356128,-9.22010791777));
#67844=CARTESIAN_POINT('Ctrl Pts',(2.0749050113,-36.3112466293,-9.12745209061));
#67845=CARTESIAN_POINT('Ctrl Pts',(2.0612711021,-36.3857400536,-9.0542168542));
#67846=CARTESIAN_POINT('Ctrl Pts',(2.05449659064,-36.4799878332,-9.01783108696));
#67847=CARTESIAN_POINT('Ctrl Pts',(2.05449659064,-36.5742356128,-9.01783108696));
#67848=CARTESIAN_POINT('Ctrl Pts',(2.10261462813,-36.2742356128,-9.31403480844));
#67849=CARTESIAN_POINT('Ctrl Pts',(2.08513070049,-36.2742356128,-9.22142274904));
#67850=CARTESIAN_POINT('Ctrl Pts',(2.06764677286,-36.3112466293,-9.12881068964));
#67851=CARTESIAN_POINT('Ctrl Pts',(2.05382701648,-36.3857400536,-9.05561022924));
#67852=CARTESIAN_POINT('Ctrl Pts',(2.04696155797,-36.4799878332,-9.01924146757));
#67853=CARTESIAN_POINT('Ctrl Pts',(2.04696155797,-36.5742356128,-9.01924146757));
#67854=CARTESIAN_POINT('Ctrl Pts',(2.09588758326,-36.2742356128,-9.31531579883));
#67855=CARTESIAN_POINT('Ctrl Pts',(2.07816577093,-36.2742356128,-9.22274905448));
#67856=CARTESIAN_POINT('Ctrl Pts',(2.0604439586,-36.3112466293,-9.13018231014));
#67857=CARTESIAN_POINT('Ctrl Pts',(2.04643710585,-36.3857400536,-9.05701748476));
#67858=CARTESIAN_POINT('Ctrl Pts',(2.03947730261,-36.4799878332,-9.02066670026));
#67859=CARTESIAN_POINT('Ctrl Pts',(2.03947730261,-36.5742356128,-9.02066670026));
#67860=CARTESIAN_POINT('Ctrl Pts',(2.0924351229,-36.2742356128,-9.31597928737));
#67861=CARTESIAN_POINT('Ctrl Pts',(2.07460058288,-36.2742356128,-9.22343417963));
#67862=CARTESIAN_POINT('Ctrl Pts',(2.05676604286,-36.3112466293,-9.13088907189));
#67863=CARTESIAN_POINT('Ctrl Pts',(2.04266777108,-36.3857400536,-9.05774180306));
#67864=CARTESIAN_POINT('Ctrl Pts',(2.03566601887,-36.4799878332,-9.02139906025));
#67865=CARTESIAN_POINT('Ctrl Pts',(2.03566601887,-36.5742356128,-9.02139906025));
#67866=CARTESIAN_POINT('Ctrl Pts',(2.08916179444,-36.2742356128,-9.31661328133));
#67867=CARTESIAN_POINT('Ctrl Pts',(2.07120234504,-36.2742356128,-9.22409238783));
#67868=CARTESIAN_POINT('Ctrl Pts',(2.05324289565,-36.3112466293,-9.13157149433));
#67869=CARTESIAN_POINT('Ctrl Pts',(2.03904898765,-36.3857400536,-9.05844275779));
#67870=CARTESIAN_POINT('Ctrl Pts',(2.03199509152,-36.4799878332,-9.02211013053));
#67871=CARTESIAN_POINT('Ctrl Pts',(2.03199509152,-36.5742356128,-9.02211013053));
#67872=CARTESIAN_POINT('Ctrl Pts',(2.08574076981,-36.2742356128,-9.31728177401));
#67873=CARTESIAN_POINT('Ctrl Pts',(2.06766662735,-36.2742356128,-9.2247832911));
#67874=CARTESIAN_POINT('Ctrl Pts',(2.04959248489,-36.3112466293,-9.13228480819));
#67875=CARTESIAN_POINT('Ctrl Pts',(2.03530668666,-36.3857400536,-9.05917402763));
#67876=CARTESIAN_POINT('Ctrl Pts',(2.02820898752,-36.4799878332,-9.02284995833));
#67877=CARTESIAN_POINT('Ctrl Pts',(2.02820898752,-36.5742356128,-9.02284995833));
#67878=CARTESIAN_POINT('',(2.02820898731014,-36.5742356128,-9.02284995728736));
#67879=CARTESIAN_POINT('Origin',(2.08533354520416,-36.5721143212383,-9.31519993529546));
#67880=CARTESIAN_POINT('Origin',(2.46549092919547,-36.5742356128,-11.235936157823));
#67881=CARTESIAN_POINT('Ctrl Pts',(2.02820898783,-37.9742356128,-9.02284995993));
#67882=CARTESIAN_POINT('Ctrl Pts',(2.02820898784,-38.0684833925,-9.02284995993));
#67883=CARTESIAN_POINT('Ctrl Pts',(2.03530642737,-38.1627311721,-9.05917408011));
#67884=CARTESIAN_POINT('Ctrl Pts',(2.04959170303,-38.2372245964,-9.1322849631));
#67885=CARTESIAN_POINT('Ctrl Pts',(2.06766518434,-38.2742356129,-9.2247835756));
#67886=CARTESIAN_POINT('Ctrl Pts',(2.08573866565,-38.2742356128,-9.31728218809));
#67887=CARTESIAN_POINT('Ctrl Pts',(2.03579644621,-37.9742356128,-9.02136733755));
#67888=CARTESIAN_POINT('Ctrl Pts',(2.03579644598,-38.0684833923,-9.0213673376));
#67889=CARTESIAN_POINT('Ctrl Pts',(2.04280758136,-38.1627311717,-9.05770831662));
#67890=CARTESIAN_POINT('Ctrl Pts',(2.05691513298,-38.2372245959,-9.13085392264));
#67891=CARTESIAN_POINT('Ctrl Pts',(2.07476544794,-38.2742356126,-9.22339613411));
#67892=CARTESIAN_POINT('Ctrl Pts',(2.09261576301,-38.2742356128,-9.31593834568));
#67893=CARTESIAN_POINT('Ctrl Pts',(2.04241519624,-37.9742356128,-9.02009857614));
#67894=CARTESIAN_POINT('Ctrl Pts',(2.04241519751,-38.0684833934,-9.02009857588));
#67895=CARTESIAN_POINT('Ctrl Pts',(2.04927723066,-38.162731174,-9.05646842916));
#67896=CARTESIAN_POINT('Ctrl Pts',(2.06305130931,-38.2372245982,-9.12967864434));
#67897=CARTESIAN_POINT('Ctrl Pts',(2.0805332169,-38.2742356144,-9.22229220064));
#67898=CARTESIAN_POINT('Ctrl Pts',(2.09801512347,-38.2742356128,-9.31490575612));
#67899=CARTESIAN_POINT('Ctrl Pts',(2.05016977896,-37.9742356128,-9.01862581454));
#67900=CARTESIAN_POINT('Ctrl Pts',(2.05016990862,-38.0684833525,-9.01862579091));
#67901=CARTESIAN_POINT('Ctrl Pts',(2.05712054303,-38.1627310922,-9.05497938491));
#67902=CARTESIAN_POINT('Ctrl Pts',(2.07094926138,-38.2372244929,-9.12817894215));
#67903=CARTESIAN_POINT('Ctrl Pts',(2.08878910363,-38.2742355501,-9.22072706798));
#67904=CARTESIAN_POINT('Ctrl Pts',(2.1066289132,-38.2742356128,-9.31327521737));
#67905=CARTESIAN_POINT('Ctrl Pts',(2.05824162123,-37.9742356128,-9.01713030917));
#67906=CARTESIAN_POINT('Ctrl Pts',(2.05824162123,-38.0684833924,-9.01713030917));
#67907=CARTESIAN_POINT('Ctrl Pts',(2.06496151432,-38.1627311721,-9.05352627015));
#67908=CARTESIAN_POINT('Ctrl Pts',(2.07850921618,-38.2372245951,-9.12677767742));
#67909=CARTESIAN_POINT('Ctrl Pts',(2.0956401522,-38.2742356128,-9.2194557914));
#67910=CARTESIAN_POINT('Ctrl Pts',(2.11277109007,-38.2742356128,-9.31213390404));
#67911=CARTESIAN_POINT('Ctrl Pts',(2.06575948168,-37.9742356128,-9.01576047707));
#67912=CARTESIAN_POINT('Ctrl Pts',(2.06575948168,-38.0684833924,-9.01576047707));
#67913=CARTESIAN_POINT('Ctrl Pts',(2.07239403611,-38.1627311721,-9.05217198666));
#67914=CARTESIAN_POINT('Ctrl Pts',(2.08574764605,-38.2372245963,-9.12545876147));
#67915=CARTESIAN_POINT('Ctrl Pts',(2.10264240018,-38.2742356128,-9.21817990924));
#67916=CARTESIAN_POINT('Ctrl Pts',(2.11953715431,-38.2742356128,-9.31090105701));
#67917=CARTESIAN_POINT('',(2.02820898738765,-37.9742356128,-9.02284995768736));
#67918=CARTESIAN_POINT('Origin',(2.46549092919547,-37.9742356128,-11.235936157823));
#67919=CARTESIAN_POINT('Origin',(2.08533051776226,-37.9763569038635,-9.3152005273479));
#67920=CARTESIAN_POINT('Origin',(2.60353950659216,-37.9742356128,-11.9671837481076));
#67921=CARTESIAN_POINT('',(2.02820898725,-37.2742356128,-9.02284995699));
#67922=CARTESIAN_POINT('Ctrl Pts',(2.08574170933,-36.2742356128,-9.31728158894));
#67923=CARTESIAN_POINT('Ctrl Pts',(2.06766727163,-36.2742356128,-9.22478316375));
#67924=CARTESIAN_POINT('Ctrl Pts',(2.04959283393,-36.3112466293,-9.13228473855));
#67925=CARTESIAN_POINT('Ctrl Pts',(2.03530680234,-36.3857400536,-9.05917400362));
#67926=CARTESIAN_POINT('Ctrl Pts',(2.02820898725,-36.4799878332,-9.02284995699));
#67927=CARTESIAN_POINT('Ctrl Pts',(2.02820898725,-36.5742356128,-9.02284995699));
#67928=CARTESIAN_POINT('Ctrl Pts',(1.88030492013,-36.2742356128,-9.35742448262));
#67929=CARTESIAN_POINT('Ctrl Pts',(1.87601517131,-36.2742356128,-9.26223249264));
#67930=CARTESIAN_POINT('Ctrl Pts',(1.87172542249,-36.3112466293,-9.16704050267));
#67931=CARTESIAN_POINT('Ctrl Pts',(1.86833480716,-36.3857400536,-9.09180077438));
#67932=CARTESIAN_POINT('Ctrl Pts',(1.86665022554,-36.4799878332,-9.05441896768));
#67933=CARTESIAN_POINT('Ctrl Pts',(1.86665022554,-36.5742356128,-9.05441896768));
#67934=CARTESIAN_POINT('Ctrl Pts',(1.66720984854,-36.2742356128,-9.35934604645));
#67935=CARTESIAN_POINT('Ctrl Pts',(1.6772952561,-36.2742356128,-9.26400888229));
#67936=CARTESIAN_POINT('Ctrl Pts',(1.68738066366,-36.3112466293,-9.16867171814));
#67937=CARTESIAN_POINT('Ctrl Pts',(1.69535216508,-36.3857400536,-9.09331724462));
#67938=CARTESIAN_POINT('Ctrl Pts',(1.69931269786,-36.4799878332,-9.05587842773));
#67939=CARTESIAN_POINT('Ctrl Pts',(1.69931269786,-36.5742356128,-9.05587842773));
#67940=CARTESIAN_POINT('Ctrl Pts',(1.45620168108,-36.2742356128,-9.32056455888));
#67941=CARTESIAN_POINT('Ctrl Pts',(1.48053714367,-36.2742356128,-9.22791078978));
#67942=CARTESIAN_POINT('Ctrl Pts',(1.50487260626,-36.3112466293,-9.13525702068));
#67943=CARTESIAN_POINT('Ctrl Pts',(1.52410735302,-36.3857400536,-9.06202365388));
#67944=CARTESIAN_POINT('Ctrl Pts',(1.53366386436,-36.4799878332,-9.02563845191));
#67945=CARTESIAN_POINT('Ctrl Pts',(1.53366386436,-36.5742356128,-9.02563845191));
#67946=CARTESIAN_POINT('Ctrl Pts',(0.987909440581,-36.2742356128,-9.13885167431));
#67947=CARTESIAN_POINT('Ctrl Pts',(1.04376958449,-36.2742356128,-9.05831007195));
#67948=CARTESIAN_POINT('Ctrl Pts',(1.0996297284,-36.3112466293,-8.9777684696));
#67949=CARTESIAN_POINT('Ctrl Pts',(1.14378156832,-36.3857400536,-8.91410819697));
#67950=CARTESIAN_POINT('Ctrl Pts',(1.16571780109,-36.4799878332,-8.88247979152));
#67951=CARTESIAN_POINT('Ctrl Pts',(1.16571780109,-36.5742356128,-8.88247979152));
#67952=CARTESIAN_POINT('Ctrl Pts',(0.634280235908,-36.2742356128,-8.77195100368));
#67953=CARTESIAN_POINT('Ctrl Pts',(0.713875172545,-36.2742356128,-8.71622821272));
#67954=CARTESIAN_POINT('Ctrl Pts',(0.793470109182,-36.3112466293,-8.66050542177));
#67955=CARTESIAN_POINT('Ctrl Pts',(0.856381940119,-36.3857400536,-8.61646242435));
#67956=CARTESIAN_POINT('Ctrl Pts',(0.887638788125,-36.4799878332,-8.59457985122));
#67957=CARTESIAN_POINT('Ctrl Pts',(0.887638788125,-36.5742356128,-8.59457985122));
#67958=CARTESIAN_POINT('Ctrl Pts',(0.489143266094,-36.2742356128,-8.5130156531));
#67959=CARTESIAN_POINT('Ctrl Pts',(0.578565086551,-36.2742356128,-8.47420086576));
#67960=CARTESIAN_POINT('Ctrl Pts',(0.667986907007,-36.3112466293,-8.43538607842));
#67961=CARTESIAN_POINT('Ctrl Pts',(0.738665869701,-36.3857400536,-8.40470575012));
#67962=CARTESIAN_POINT('Ctrl Pts',(0.773781761013,-36.4799878332,-8.3894643477));
#67963=CARTESIAN_POINT('Ctrl Pts',(0.773781761013,-36.5742356128,-8.3894643477));
#67964=CARTESIAN_POINT('Ctrl Pts',(0.417258904585,-36.2742356128,-8.22711946983));
#67965=CARTESIAN_POINT('Ctrl Pts',(0.511506458023,-36.2742356128,-8.20836329279));
#67966=CARTESIAN_POINT('Ctrl Pts',(0.60575401146,-36.3112466293,-8.18960711575));
#67967=CARTESIAN_POINT('Ctrl Pts',(0.680247273964,-36.3857400536,-8.17478299056));
#67968=CARTESIAN_POINT('Ctrl Pts',(0.717258184663,-36.4799878332,-8.16741670403));
#67969=CARTESIAN_POINT('Ctrl Pts',(0.717258184663,-36.5742356128,-8.16741670403));
#67970=CARTESIAN_POINT('Ctrl Pts',(0.417255480809,-36.2742356128,-7.94319578605));
#67971=CARTESIAN_POINT('Ctrl Pts',(0.51150326041,-36.2742356128,-7.94319464953));
#67972=CARTESIAN_POINT('Ctrl Pts',(0.60575104001,-36.3112466293,-7.94319351302));
#67973=CARTESIAN_POINT('Ctrl Pts',(0.680244464285,-36.3857400536,-7.94319261472));
#67974=CARTESIAN_POINT('Ctrl Pts',(0.717255480787,-36.4799878332,-7.94319216841));
#67975=CARTESIAN_POINT('Ctrl Pts',(0.717255480787,-36.5742356128,-7.94319216841));
#67976=CARTESIAN_POINT('',(0.717273457110329,-36.5742356128,-7.94951682245649));
#67977=CARTESIAN_POINT('Ctrl Pts',(0.717273550273509,-36.5742356128,-7.94951682199161));
#67978=CARTESIAN_POINT('Ctrl Pts',(0.717273718212123,-36.5569116248149,
-7.94954627039414));
#67979=CARTESIAN_POINT('Ctrl Pts',(0.715768903123445,-36.5395872493805,
-7.94957487707452));
#67980=CARTESIAN_POINT('Ctrl Pts',(0.71277861671105,-36.5225244523691,-7.9496036226719));
#67981=CARTESIAN_POINT('Ctrl Pts',(0.709713242042008,-36.505033196172,-7.94963309009205));
#67982=CARTESIAN_POINT('Ctrl Pts',(0.705087023665518,-36.4878172698378,
-7.94966269785234));
#67983=CARTESIAN_POINT('Ctrl Pts',(0.698974456303144,-36.4711465076226,
-7.94969279420693));
#67984=CARTESIAN_POINT('Ctrl Pts',(0.692790765864684,-36.4542817719394,
-7.94972324074913));
#67985=CARTESIAN_POINT('Ctrl Pts',(0.685086262181111,-36.4379754276189,
-7.94975417739394));
#67986=CARTESIAN_POINT('Ctrl Pts',(0.67598818460903,-36.4224873686871,-7.94978537077702));
#67987=CARTESIAN_POINT('Ctrl Pts',(0.666789257765644,-36.4068276295904,
-7.94981690992874));
#67988=CARTESIAN_POINT('Ctrl Pts',(0.656166059019434,-36.3920049178971,
-7.94984869974283));
#67989=CARTESIAN_POINT('Ctrl Pts',(0.644295761307527,-36.3782607241328,
-7.94988006139291));
#67990=CARTESIAN_POINT('Ctrl Pts',(0.639508097400346,-36.3727172590896,
-7.94989271053144));
#67991=CARTESIAN_POINT('Ctrl Pts',(0.634518043105347,-36.3673488954339,
-7.94990528609214));
#67992=CARTESIAN_POINT('Ctrl Pts',(0.62933907671151,-36.3621699634842,-7.94991773054105));
#67993=CARTESIAN_POINT('Ctrl Pts',(0.616486900705681,-36.3493178729552,
-7.94994861281282));
#67994=CARTESIAN_POINT('Ctrl Pts',(0.602465787135931,-36.3376319498832,
-7.94997981454275));
#67995=CARTESIAN_POINT('Ctrl Pts',(0.587504932485788,-36.3273064223065,
-7.95001101814882));
#67996=CARTESIAN_POINT('Ctrl Pts',(0.572728201972024,-36.3171079716177,
-7.95004183773024));
#67997=CARTESIAN_POINT('Ctrl Pts',(0.557035218119696,-36.3082369941902,
-7.95007264840558));
#67998=CARTESIAN_POINT('Ctrl Pts',(0.540675695845687,-36.3008391875838,
-7.95010325026941));
#67999=CARTESIAN_POINT('Ctrl Pts',(0.524509427466709,-36.2935287707505,
-7.95013349063556));
#68000=CARTESIAN_POINT('Ctrl Pts',(0.507692734616536,-36.287657247099,-7.95016351980852));
#68001=CARTESIAN_POINT('Ctrl Pts',(0.490487885069218,-36.2833194732264,
-7.95019338220779));
#68002=CARTESIAN_POINT('Ctrl Pts',(0.473641257747844,-36.2790720161571,
-7.95022262284195));
#68003=CARTESIAN_POINT('Ctrl Pts',(0.456422901148918,-36.2762953079016,
-7.95025170029614));
#68004=CARTESIAN_POINT('Ctrl Pts',(0.439093000583099,-36.2750305592133,
-7.95028096141245));
#68005=CARTESIAN_POINT('Ctrl Pts',(0.431832792919537,-36.2745007040024,
-7.95029322009679));
#68006=CARTESIAN_POINT('Ctrl Pts',(0.424553142006894,-36.2742356128,-7.95030551501276));
#68007=CARTESIAN_POINT('Ctrl Pts',(0.417273658050834,-36.2742356128,-7.95031788947841));
#68008=CARTESIAN_POINT('Ctrl Pts',(2.02820898725,-36.5742356128,-9.02284995699));
#68009=CARTESIAN_POINT('Ctrl Pts',(1.64860914359,-36.5742356128,-9.09702477361));
#68010=CARTESIAN_POINT('Ctrl Pts',(1.23586688919,-36.5742356128,-9.00518418336));
#68011=CARTESIAN_POINT('Ctrl Pts',(0.890959353803,-36.5742356128,-8.72278991704));
#68012=CARTESIAN_POINT('Ctrl Pts',(0.719470863523,-36.5742356128,-8.33628951564));
#68013=CARTESIAN_POINT('Ctrl Pts',(0.717273426056,-36.5742356128,-7.9495168227));
#68014=CARTESIAN_POINT('Ctrl Pts',(0.7172606582,-37.9742356128,-7.94658833073));
#68015=CARTESIAN_POINT('Ctrl Pts',(0.7172606582,-38.0684833924,-7.94658833073));
#68016=CARTESIAN_POINT('Ctrl Pts',(0.680249812977,-38.1627311721,-7.94670092992));
#68017=CARTESIAN_POINT('Ctrl Pts',(0.605756733441,-38.2372245963,-7.94692756242));
#68018=CARTESIAN_POINT('Ctrl Pts',(0.511509389998,-38.2742356128,-7.9472142939));
#68019=CARTESIAN_POINT('Ctrl Pts',(0.417262046555,-38.2742356128,-7.94750102538));
#68020=CARTESIAN_POINT('Ctrl Pts',(0.717867533103,-37.9742356128,-8.14606537112));
#68021=CARTESIAN_POINT('Ctrl Pts',(0.717867533103,-38.0684833924,-8.14606537112));
#68022=CARTESIAN_POINT('Ctrl Pts',(0.680876846203,-38.1627311721,-8.15279980919));
#68023=CARTESIAN_POINT('Ctrl Pts',(0.60642431038,-38.237224596,-8.16635699061));
#68024=CARTESIAN_POINT('Ctrl Pts',(0.512228274053,-38.2742356128,-8.18350823638));
#68025=CARTESIAN_POINT('Ctrl Pts',(0.418032238021,-38.2742356128,-8.20065948222));
#68026=CARTESIAN_POINT('Ctrl Pts',(0.763363662931,-37.9742356128,-8.34442356823));
#68027=CARTESIAN_POINT('Ctrl Pts',(0.763363667813,-38.0684833919,-8.34442352344));
#68028=CARTESIAN_POINT('Ctrl Pts',(0.727897495111,-38.1627311709,-8.35801562032));
#68029=CARTESIAN_POINT('Ctrl Pts',(0.656513470554,-38.2372245955,-8.38536918483));
#68030=CARTESIAN_POINT('Ctrl Pts',(0.566199629112,-38.2742356119,-8.41997806019));
#68031=CARTESIAN_POINT('Ctrl Pts',(0.47588578497,-38.2742356128,-8.45458695312));
#68032=CARTESIAN_POINT('Ctrl Pts',(0.854204420009,-37.9742356128,-8.52995308217));
#68033=CARTESIAN_POINT('Ctrl Pts',(0.854204232522,-38.0684833927,-8.52995300167));
#68034=CARTESIAN_POINT('Ctrl Pts',(0.821817681684,-38.1627311726,-8.5496918088));
#68035=CARTESIAN_POINT('Ctrl Pts',(0.756629824743,-38.2372245969,-8.58942235372));
#68036=CARTESIAN_POINT('Ctrl Pts',(0.674156446967,-38.2742356133,-8.6396881941));
#68037=CARTESIAN_POINT('Ctrl Pts',(0.591683143127,-38.2742356128,-8.68995406613));
#68038=CARTESIAN_POINT('Ctrl Pts',(1.10581964187,-37.9742356128,-8.83717100477));
#68039=CARTESIAN_POINT('Ctrl Pts',(1.1058198191,-38.0684833922,-8.83717108086));
#68040=CARTESIAN_POINT('Ctrl Pts',(1.08188082307,-38.1627311716,-8.8672647092));
#68041=CARTESIAN_POINT('Ctrl Pts',(1.03370006531,-38.2372245958,-8.92783380533));
#68042=CARTESIAN_POINT('Ctrl Pts',(0.972741517449,-38.2742356124,-9.00446529129));
#68043=CARTESIAN_POINT('Ctrl Pts',(0.911782899689,-38.2742356128,-9.08109674732));
#68044=CARTESIAN_POINT('Ctrl Pts',(1.46215717903,-37.9742356128,-9.01047889206));
#68045=CARTESIAN_POINT('Ctrl Pts',(1.46215701149,-38.0684833927,-9.01047882012));
#68046=CARTESIAN_POINT('Ctrl Pts',(1.450187899,-38.1627311725,-9.04635771927));
#68047=CARTESIAN_POINT('Ctrl Pts',(1.4260952181,-38.2372245969,-9.11857386339));
#68048=CARTESIAN_POINT('Ctrl Pts',(1.3956146111,-38.2742356132,-9.2099399714));
#68049=CARTESIAN_POINT('Ctrl Pts',(1.36513407019,-38.2742356128,-9.30130610772));
#68050=CARTESIAN_POINT('Ctrl Pts',(1.65094597751,-37.9742356128,-9.0556796597));
#68051=CARTESIAN_POINT('Ctrl Pts',(1.65094609924,-38.0684833926,-9.05567973396));
#68052=CARTESIAN_POINT('Ctrl Pts',(1.64534839287,-38.1627311724,-9.09311495351));
#68053=CARTESIAN_POINT('Ctrl Pts',(1.63409038501,-38.2372245964,-9.16846036625));
#68054=CARTESIAN_POINT('Ctrl Pts',(1.61984316027,-38.2742356131,-9.26378674848));
#68055=CARTESIAN_POINT('Ctrl Pts',(1.60559588761,-38.2742356128,-9.35911310119));
#68056=CARTESIAN_POINT('Ctrl Pts',(1.8433625614,-37.9742356128,-9.05896943904));
#68057=CARTESIAN_POINT('Ctrl Pts',(1.8433625614,-38.0684833924,-9.05896943904));
#68058=CARTESIAN_POINT('Ctrl Pts',(1.84426881625,-38.1627311721,-9.09650333241));
#68059=CARTESIAN_POINT('Ctrl Pts',(1.84608697067,-38.2372245966,-9.17205032437));
#68060=CARTESIAN_POINT('Ctrl Pts',(1.84838974451,-38.2742356128,-9.26763057434));
#68061=CARTESIAN_POINT('Ctrl Pts',(1.85069251843,-38.2742356128,-9.36321082448));
#68062=CARTESIAN_POINT('Ctrl Pts',(2.02820898725,-37.9742356128,-9.02284995699));
#68063=CARTESIAN_POINT('Ctrl Pts',(2.02820898725,-38.0684833924,-9.02284995699));
#68064=CARTESIAN_POINT('Ctrl Pts',(2.03530680234,-38.1627311721,-9.05917400362));
#68065=CARTESIAN_POINT('Ctrl Pts',(2.04959283393,-38.2372245963,-9.13228473855));
#68066=CARTESIAN_POINT('Ctrl Pts',(2.06766727163,-38.2742356128,-9.22478316375));
#68067=CARTESIAN_POINT('Ctrl Pts',(2.08574170933,-38.2742356128,-9.31728158894));
#68068=CARTESIAN_POINT('',(0.717273429106671,-37.9742356128,-7.94951682267615));
#68069=CARTESIAN_POINT('Ctrl Pts',(2.02820898725,-37.9742356128,-9.02284995699));
#68070=CARTESIAN_POINT('Ctrl Pts',(1.64860914359,-37.9742356128,-9.09702477361));
#68071=CARTESIAN_POINT('Ctrl Pts',(1.23586688919,-37.9742356128,-9.00518418336));
#68072=CARTESIAN_POINT('Ctrl Pts',(0.890959353803,-37.9742356128,-8.72278991704));
#68073=CARTESIAN_POINT('Ctrl Pts',(0.719470863523,-37.9742356128,-8.33628951564));
#68074=CARTESIAN_POINT('Ctrl Pts',(0.717273426056,-37.9742356128,-7.9495168227));
#68075=CARTESIAN_POINT('Ctrl Pts',(0.417273442888033,-38.2742356128,-7.95031782080527));
#68076=CARTESIAN_POINT('Ctrl Pts',(0.434598525986889,-38.2742356128,-7.95028837214399));
#68077=CARTESIAN_POINT('Ctrl Pts',(0.451923974993303,-38.2727304797968,
-7.95025935917568));
#68078=CARTESIAN_POINT('Ctrl Pts',(0.468987789398651,-38.2697397345538,
-7.95023028762418));
#68079=CARTESIAN_POINT('Ctrl Pts',(0.486480149422269,-38.2666738788613,
-7.95020048596125));
#68080=CARTESIAN_POINT('Ctrl Pts',(0.503697118834521,-38.2620470205853,
-7.9501706245799));
#68081=CARTESIAN_POINT('Ctrl Pts',(0.520368827692176,-38.2559336669727,
-7.95014052771515));
#68082=CARTESIAN_POINT('Ctrl Pts',(0.53723453530731,-38.2497491759011,-7.95011008063109));
#68083=CARTESIAN_POINT('Ctrl Pts',(0.553541752130104,-38.2420437192392,
-7.95007939879925));
#68084=CARTESIAN_POINT('Ctrl Pts',(0.56903054794127,-38.2329445513992,-7.95004859832233));
#68085=CARTESIAN_POINT('Ctrl Pts',(0.584691001018681,-38.2237445404532,
-7.95001745649379));
#68086=CARTESIAN_POINT('Ctrl Pts',(0.599514291550423,-38.2131201228315,
-7.94998620332128));
#68087=CARTESIAN_POINT('Ctrl Pts',(0.613258891559137,-38.2012484884415,
-7.94995513871314));
#68088=CARTESIAN_POINT('Ctrl Pts',(0.618798575895286,-38.1964636924465,
-7.94994261829618));
#68089=CARTESIAN_POINT('Ctrl Pts',(0.624163379983104,-38.1914767749953,
-7.94993012967329));
#68090=CARTESIAN_POINT('Ctrl Pts',(0.629339001124755,-38.1863011865543,
-7.94991769434846));
#68091=CARTESIAN_POINT('Ctrl Pts',(0.642190475730227,-38.1734497931471,
-7.94988681645827));
#68092=CARTESIAN_POINT('Ctrl Pts',(0.653875928692519,-38.1594295641484,
-7.9498551419374));
#68093=CARTESIAN_POINT('Ctrl Pts',(0.664201133736344,-38.1444696525599,
-7.94982348173407));
#68094=CARTESIAN_POINT('Ctrl Pts',(0.674399245792677,-38.129693882579,-7.94979221123631));
#68095=CARTESIAN_POINT('Ctrl Pts',(0.683270033662761,-38.1140019200491,
-7.94976096659087));
#68096=CARTESIAN_POINT('Ctrl Pts',(0.690667797597331,-38.097643441461,-7.94973017875777));
#68097=CARTESIAN_POINT('Ctrl Pts',(0.697978168202641,-38.081478213417,-7.94969975463609));
#68098=CARTESIAN_POINT('Ctrl Pts',(0.703849790613318,-38.0646625836195,
-7.94966978700977));
#68099=CARTESIAN_POINT('Ctrl Pts',(0.708187802634565,-38.0474587849797,
-7.94964018198505));
#68100=CARTESIAN_POINT('Ctrl Pts',(0.712435492937246,-38.0306131865135,
-7.94961119336634));
#68101=CARTESIAN_POINT('Ctrl Pts',(0.715212568059503,-38.0133958472847,
-7.94958255936925));
#68102=CARTESIAN_POINT('Ctrl Pts',(0.71647780862749,-37.9960669200146,-7.94955357367437));
#68103=CARTESIAN_POINT('Ctrl Pts',(0.717008189396048,-37.9888027443343,
-7.94954142305612));
#68104=CARTESIAN_POINT('Ctrl Pts',(0.717273508649237,-37.9815190941805,
-7.94952920247982));
#68105=CARTESIAN_POINT('Ctrl Pts',(0.717273438258802,-37.9742356128,-7.94951682263062));
#68106=CARTESIAN_POINT('Ctrl Pts',(2.02820898725,-37.9742356128,-9.02284995699));
#68107=CARTESIAN_POINT('Ctrl Pts',(2.02820898725,-36.2942356128,-9.02284995699));
#68108=CARTESIAN_POINT('Ctrl Pts',(1.64860914359,-37.9742356128,-9.09702477361));
#68109=CARTESIAN_POINT('Ctrl Pts',(1.64860914359,-36.2942356128,-9.09702477361));
#68110=CARTESIAN_POINT('Ctrl Pts',(1.23586688919,-37.9742356128,-9.00518418336));
#68111=CARTESIAN_POINT('Ctrl Pts',(1.23586688919,-36.2942356128,-9.00518418336));
#68112=CARTESIAN_POINT('Ctrl Pts',(0.890959353803,-37.9742356128,-8.72278991704));
#68113=CARTESIAN_POINT('Ctrl Pts',(0.890959353803,-36.2942356128,-8.72278991704));
#68114=CARTESIAN_POINT('Ctrl Pts',(0.719470863523,-37.9742356128,-8.33628951564));
#68115=CARTESIAN_POINT('Ctrl Pts',(0.719470863523,-36.2942356128,-8.33628951564));
#68116=CARTESIAN_POINT('Ctrl Pts',(0.717273426056,-37.9742356128,-7.9495168227));
#68117=CARTESIAN_POINT('Ctrl Pts',(0.717273426056,-36.2942356128,-7.9495168227));
#68118=CARTESIAN_POINT('',(0.717273426056,-37.2742356128,-7.9495168227));
#68119=CARTESIAN_POINT('Origin',(0.417273426056,-36.5742356128,0.915007091638));
#68120=CARTESIAN_POINT('',(0.717273426056,-36.5742356128,-3.28965091665));
#68121=CARTESIAN_POINT('Origin',(0.41939471766068,-36.5721143212087,-3.28965091665326));
#68122=CARTESIAN_POINT('',(0.717273426056,-36.5742356128,-5.61958386968));
#68123=CARTESIAN_POINT('Origin',(0.417273426056,-37.9742356128,0.916320001688));
#68124=CARTESIAN_POINT('',(0.717273426056,-37.9742356128,-3.28965091665));
#68125=CARTESIAN_POINT('',(0.717273426056,-37.9742356128,-5.61958386968));
#68126=CARTESIAN_POINT('Origin',(0.419394717187198,-37.9763569039297,-3.28965091667348));
#68127=CARTESIAN_POINT('Origin',(0.717273426056,-38.2742356128,-7.9495168227));
#68128=CARTESIAN_POINT('',(0.717273426056,-37.2742356128,-3.28965091665));
#68129=CARTESIAN_POINT('Ctrl Pts',(0.417273426056,-36.2742356128,-3.28965091665));
#68130=CARTESIAN_POINT('Ctrl Pts',(0.511521205664,-36.2742356128,-3.28965091665));
#68131=CARTESIAN_POINT('Ctrl Pts',(0.605768985271,-36.3112466293,-3.28965091665));
#68132=CARTESIAN_POINT('Ctrl Pts',(0.680262409552,-36.3857400536,-3.28965091665));
#68133=CARTESIAN_POINT('Ctrl Pts',(0.717273426056,-36.4799878332,-3.28965091665));
#68134=CARTESIAN_POINT('Ctrl Pts',(0.717273426056,-36.5742356128,-3.28965091665));
#68135=CARTESIAN_POINT('Ctrl Pts',(0.417273426056,-36.2742356128,-3.16524611306));
#68136=CARTESIAN_POINT('Ctrl Pts',(0.511521205664,-36.2742356128,-3.18000729667));
#68137=CARTESIAN_POINT('Ctrl Pts',(0.605768985271,-36.3112466293,-3.19476848028));
#68138=CARTESIAN_POINT('Ctrl Pts',(0.680262408262,-36.3857400536,-3.20643571855));
#68139=CARTESIAN_POINT('Ctrl Pts',(0.717273426056,-36.4799878332,-3.21223241981));
#68140=CARTESIAN_POINT('Ctrl Pts',(0.717273426056,-36.5742356128,-3.21223241981));
#68141=CARTESIAN_POINT('Ctrl Pts',(0.441599544527,-36.2742356128,-3.04112730047));
#68142=CARTESIAN_POINT('Ctrl Pts',(0.532969569844,-36.2742356128,-3.07035582302));
#68143=CARTESIAN_POINT('Ctrl Pts',(0.624339595161,-36.3112466293,-3.09958434558));
#68144=CARTESIAN_POINT('Ctrl Pts',(0.696558447571,-36.3857400536,-3.12268655792));
#68145=CARTESIAN_POINT('Ctrl Pts',(0.73243936812,-36.4799878332,-3.13416457735));
#68146=CARTESIAN_POINT('Ctrl Pts',(0.73243936812,-36.5742356128,-3.13416457735));
#68147=CARTESIAN_POINT('Ctrl Pts',(0.48971071229,-36.2742356128,-2.92311263468));
#68148=CARTESIAN_POINT('Ctrl Pts',(0.575439222257,-36.2742356128,-2.96626059864));
#68149=CARTESIAN_POINT('Ctrl Pts',(0.661167732224,-36.3112466293,-3.0094085626));
#68150=CARTESIAN_POINT('Ctrl Pts',(0.728928155046,-36.3857400536,-3.04351258121));
#68151=CARTESIAN_POINT('Ctrl Pts',(0.762593034794,-36.4799878332,-3.06045686966));
#68152=CARTESIAN_POINT('Ctrl Pts',(0.762593034794,-36.5742356128,-3.06045686966));
#68153=CARTESIAN_POINT('Ctrl Pts',(0.613174121579,-36.2742356128,-2.73656462166));
#68154=CARTESIAN_POINT('Ctrl Pts',(0.68434190078,-36.2742356128,-2.8017427822));
#68155=CARTESIAN_POINT('Ctrl Pts',(0.755509679981,-36.3112466293,-2.86692094274));
#68156=CARTESIAN_POINT('Ctrl Pts',(0.811760201326,-36.3857400536,-2.91843783481));
#68157=CARTESIAN_POINT('Ctrl Pts',(0.839708198554,-36.4799878332,-2.94403315029));
#68158=CARTESIAN_POINT('Ctrl Pts',(0.839708198554,-36.5742356128,-2.94403315029));
#68159=CARTESIAN_POINT('Ctrl Pts',(0.790505416227,-36.2742356128,-2.60290926659));
#68160=CARTESIAN_POINT('Ctrl Pts',(0.84074776272,-36.2742356128,-2.68383943279));
#68161=CARTESIAN_POINT('Ctrl Pts',(0.890990109212,-36.3112466293,-2.76476959899));
#68162=CARTESIAN_POINT('Ctrl Pts',(0.930702009443,-36.3857400536,-2.82873672124));
#68163=CARTESIAN_POINT('Ctrl Pts',(0.950431772163,-36.4799878332,-2.86051798652));
#68164=CARTESIAN_POINT('Ctrl Pts',(0.950431772163,-36.5742356128,-2.86051798652));
#68165=CARTESIAN_POINT('Ctrl Pts',(0.875558654279,-36.2742356128,-2.55689129959));
#68166=CARTESIAN_POINT('Ctrl Pts',(0.915879301025,-36.2742356128,-2.64319398283));
#68167=CARTESIAN_POINT('Ctrl Pts',(0.956199947771,-36.3112466293,-2.72949666608));
#68168=CARTESIAN_POINT('Ctrl Pts',(0.988067915893,-36.3857400536,-2.79771056105));
#68169=CARTESIAN_POINT('Ctrl Pts',(1.00390325904,-36.4799878332,-2.83160127239));
#68170=CARTESIAN_POINT('Ctrl Pts',(1.00390325904,-36.5742356128,-2.83160127239));
#68171=CARTESIAN_POINT('Ctrl Pts',(0.966362779946,-36.2742356128,-2.52404170312));
#68172=CARTESIAN_POINT('Ctrl Pts',(0.995964836957,-36.2742356128,-2.61422938163));
#68173=CARTESIAN_POINT('Ctrl Pts',(1.02556689397,-36.3112466293,-2.70441706013));
#68174=CARTESIAN_POINT('Ctrl Pts',(1.04896532681,-36.3857400536,-2.77570120058));
#68175=CARTESIAN_POINT('Ctrl Pts',(1.06058905392,-36.4799878332,-2.81111799992));
#68176=CARTESIAN_POINT('Ctrl Pts',(1.06058905392,-36.5742356128,-2.81111799992));
#68177=CARTESIAN_POINT('Ctrl Pts',(1.05996676265,-36.2742356128,-2.50526930112));
#68178=CARTESIAN_POINT('Ctrl Pts',(1.07849866849,-36.2742356128,-2.59767714375));
#68179=CARTESIAN_POINT('Ctrl Pts',(1.09703057432,-36.3112466293,-2.69008498638));
#68180=CARTESIAN_POINT('Ctrl Pts',(1.11167818862,-36.3857400536,-2.76312412488));
#68181=CARTESIAN_POINT('Ctrl Pts',(1.11895565102,-36.4799878332,-2.79941259982));
#68182=CARTESIAN_POINT('Ctrl Pts',(1.11895565102,-36.5742356128,-2.79941259982));
#68183=CARTESIAN_POINT('',(1.11895565834,-36.5742356128,-2.79941259037));
#68184=CARTESIAN_POINT('Origin',(1.06038498235599,-36.5721142080809,-2.50734904525943));
#68185=CARTESIAN_POINT('Ctrl Pts',(0.717273426056,-36.5742356128,-3.28965091665));
#68186=CARTESIAN_POINT('Ctrl Pts',(0.717273426056,-36.5742356128,-3.15236381141));
#68187=CARTESIAN_POINT('Ctrl Pts',(0.764935707726,-36.5742356128,-3.0142516443));
#68188=CARTESIAN_POINT('Ctrl Pts',(0.858305199948,-36.5742356128,-2.90029762813));
#68189=CARTESIAN_POINT('Ctrl Pts',(0.984348856958,-36.5742356128,-2.82640811382));
#68190=CARTESIAN_POINT('Ctrl Pts',(1.11895565834,-36.5742356128,-2.79941259037));
#68191=CARTESIAN_POINT('Ctrl Pts',(1.11895565835,-37.9742356128,-2.79941259036));
#68192=CARTESIAN_POINT('Ctrl Pts',(1.11895565835,-38.0684833924,-2.79941259036));
#68193=CARTESIAN_POINT('Ctrl Pts',(1.11167797924,-38.1627311721,-2.7631241524));
#68194=CARTESIAN_POINT('Ctrl Pts',(1.09702992877,-38.2372245963,-2.69008508834));
#68195=CARTESIAN_POINT('Ctrl Pts',(1.0784974711,-38.2742356128,-2.59767733988));
#68196=CARTESIAN_POINT('Ctrl Pts',(1.05996501343,-38.2742356128,-2.50526959142));
#68197=CARTESIAN_POINT('Ctrl Pts',(1.05079714613,-37.9742356128,-2.81308183852));
#68198=CARTESIAN_POINT('Ctrl Pts',(1.05079714459,-38.0684833915,-2.81308183883));
#68199=CARTESIAN_POINT('Ctrl Pts',(1.03842294874,-38.1627311702,-2.77781551551));
#68200=CARTESIAN_POINT('Ctrl Pts',(1.01350086203,-38.2372245936,-2.7068369058));
#68201=CARTESIAN_POINT('Ctrl Pts',(0.981976632903,-38.2742356114,-2.61703465975));
#68202=CARTESIAN_POINT('Ctrl Pts',(0.950452403813,-38.2742356128,-2.52723241358));
#68203=CARTESIAN_POINT('Ctrl Pts',(0.984545966087,-37.9742356128,-2.83883463086));
#68204=CARTESIAN_POINT('Ctrl Pts',(0.98454601951,-38.0684833954,-2.83883463094));
#68205=CARTESIAN_POINT('Ctrl Pts',(0.96732248259,-38.1627311779,-2.80547148767));
#68206=CARTESIAN_POINT('Ctrl Pts',(0.932680120997,-38.2372246041,-2.73831545226));
#68207=CARTESIAN_POINT('Ctrl Pts',(0.888841036929,-38.2742356175,-2.65335283513));
#68208=CARTESIAN_POINT('Ctrl Pts',(0.845001933072,-38.2742356128,-2.56839021887));
#68209=CARTESIAN_POINT('Ctrl Pts',(0.923689095375,-37.9742356128,-2.8760099825));
#68210=CARTESIAN_POINT('Ctrl Pts',(0.923689119028,-38.0684833919,-2.87600994329));
#68211=CARTESIAN_POINT('Ctrl Pts',(0.901979860215,-38.162731171,-2.84536674598));
#68212=CARTESIAN_POINT('Ctrl Pts',(0.858278675606,-38.237224595,-2.78369427505));
#68213=CARTESIAN_POINT('Ctrl Pts',(0.802991263748,-38.274235612,-2.70566561619));
#68214=CARTESIAN_POINT('Ctrl Pts',(0.747703842309,-38.2742356128,-2.62763697264));
#68215=CARTESIAN_POINT('Ctrl Pts',(0.819317393776,-37.9742356128,-2.96776730531));
#68216=CARTESIAN_POINT('Ctrl Pts',(0.819317370869,-38.068483393,-2.96776734328));
#68217=CARTESIAN_POINT('Ctrl Pts',(0.789854337745,-38.1627311731,-2.94394296668));
#68218=CARTESIAN_POINT('Ctrl Pts',(0.7305590039,-38.2372245976,-2.89598667512));
#68219=CARTESIAN_POINT('Ctrl Pts',(0.655537093063,-38.2742356137,-2.83531489222));
#68220=CARTESIAN_POINT('Ctrl Pts',(0.580515191511,-38.2742356128,-2.77464309447));
#68221=CARTESIAN_POINT('Ctrl Pts',(0.751652775661,-37.9742356128,-3.08946794145));
#68222=CARTESIAN_POINT('Ctrl Pts',(0.751652797847,-38.0684833919,-3.08946790467));
#68223=CARTESIAN_POINT('Ctrl Pts',(0.717171967169,-38.162731171,-3.07467132905));
#68224=CARTESIAN_POINT('Ctrl Pts',(0.647765324546,-38.2372245951,-3.04489371052));
#68225=CARTESIAN_POINT('Ctrl Pts',(0.559955670297,-38.274235612,-3.00721795236));
#68226=CARTESIAN_POINT('Ctrl Pts',(0.472146007049,-38.2742356128,-2.96954220859));
#68227=CARTESIAN_POINT('Ctrl Pts',(0.728810629724,-37.9742356128,-3.15397751799));
#68228=CARTESIAN_POINT('Ctrl Pts',(0.728810613963,-38.0684833915,-3.15397750075));
#68229=CARTESIAN_POINT('Ctrl Pts',(0.692660998557,-38.1627311702,-3.14394628549));
#68230=CARTESIAN_POINT('Ctrl Pts',(0.619901810784,-38.2372245934,-3.12374493319));
#68231=CARTESIAN_POINT('Ctrl Pts',(0.527847978649,-38.2742356114,-3.09819124184));
#68232=CARTESIAN_POINT('Ctrl Pts',(0.435794152725,-38.2742356128,-3.07263755644));
#68233=CARTESIAN_POINT('Ctrl Pts',(0.717273426056,-37.9742356128,-3.22232941308));
#68234=CARTESIAN_POINT('Ctrl Pts',(0.717273426056,-38.0684833924,-3.22232941308));
#68235=CARTESIAN_POINT('Ctrl Pts',(0.680262508937,-38.1627311721,-3.21728624585));
#68236=CARTESIAN_POINT('Ctrl Pts',(0.605768984872,-38.2372245968,-3.20714313748));
#68237=CARTESIAN_POINT('Ctrl Pts',(0.511521205664,-38.2742356128,-3.19430712084));
#68238=CARTESIAN_POINT('Ctrl Pts',(0.417273426056,-38.2742356128,-3.1814711047));
#68239=CARTESIAN_POINT('Ctrl Pts',(0.717273426056,-37.9742356128,-3.28965091665));
#68240=CARTESIAN_POINT('Ctrl Pts',(0.717273426056,-38.0684833924,-3.28965091665));
#68241=CARTESIAN_POINT('Ctrl Pts',(0.680262409552,-38.1627311721,-3.28965091665));
#68242=CARTESIAN_POINT('Ctrl Pts',(0.605768985271,-38.2372245963,-3.28965091665));
#68243=CARTESIAN_POINT('Ctrl Pts',(0.511521205664,-38.2742356128,-3.28965091665));
#68244=CARTESIAN_POINT('Ctrl Pts',(0.417273426056,-38.2742356128,-3.28965091665));
#68245=CARTESIAN_POINT('',(1.11895565834,-37.9742356128,-2.79941259037));
#68246=CARTESIAN_POINT('Ctrl Pts',(0.717273426056,-37.9742356128,-3.28965091665));
#68247=CARTESIAN_POINT('Ctrl Pts',(0.717273426056,-37.9742356128,-3.22232941308));
#68248=CARTESIAN_POINT('Ctrl Pts',(0.728810629724,-37.9742356128,-3.15397751799));
#68249=CARTESIAN_POINT('Ctrl Pts',(0.751652775661,-37.9742356128,-3.08946794145));
#68250=CARTESIAN_POINT('Ctrl Pts',(0.819317393776,-37.9742356128,-2.96776730531));
#68251=CARTESIAN_POINT('Ctrl Pts',(0.923689095375,-37.9742356128,-2.8760099825));
#68252=CARTESIAN_POINT('Ctrl Pts',(0.984545966087,-37.9742356128,-2.83883463086));
#68253=CARTESIAN_POINT('Ctrl Pts',(1.05079714613,-37.9742356128,-2.81308183852));
#68254=CARTESIAN_POINT('Ctrl Pts',(1.11895565834,-37.9742356128,-2.79941259037));
#68255=CARTESIAN_POINT('Origin',(1.06038213453216,-37.9763569039054,-2.50734946784708));
#68256=CARTESIAN_POINT('Ctrl Pts',(0.717273426056,-37.9742356128,-3.28965091665));
#68257=CARTESIAN_POINT('Ctrl Pts',(0.717273426056,-36.2942356128,-3.28965091665));
#68258=CARTESIAN_POINT('Ctrl Pts',(0.717273426056,-37.9742356128,-3.15236381141));
#68259=CARTESIAN_POINT('Ctrl Pts',(0.717273426056,-36.2942356128,-3.15236381141));
#68260=CARTESIAN_POINT('Ctrl Pts',(0.764935707726,-37.9742356128,-3.0142516443));
#68261=CARTESIAN_POINT('Ctrl Pts',(0.764935707726,-36.2942356128,-3.0142516443));
#68262=CARTESIAN_POINT('Ctrl Pts',(0.858305199948,-37.9742356128,-2.90029762813));
#68263=CARTESIAN_POINT('Ctrl Pts',(0.858305199948,-36.2942356128,-2.90029762813));
#68264=CARTESIAN_POINT('Ctrl Pts',(0.984348856958,-37.9742356128,-2.82640811382));
#68265=CARTESIAN_POINT('Ctrl Pts',(0.984348856958,-36.2942356128,-2.82640811382));
#68266=CARTESIAN_POINT('Ctrl Pts',(1.11895565834,-37.9742356128,-2.79941259037));
#68267=CARTESIAN_POINT('Ctrl Pts',(1.11895565834,-36.2942356128,-2.79941259037));
#68268=CARTESIAN_POINT('',(1.11895565834,-37.2742356128,-2.79941259037));
#68269=CARTESIAN_POINT('Ctrl Pts',(1.05996499772,-36.2742356128,-2.50526959461));
#68270=CARTESIAN_POINT('Ctrl Pts',(1.07849746032,-36.2742356128,-2.59767734207));
#68271=CARTESIAN_POINT('Ctrl Pts',(1.09702992293,-36.3112466293,-2.69008508953));
#68272=CARTESIAN_POINT('Ctrl Pts',(1.1116779773,-36.3857400536,-2.7631241528));
#68273=CARTESIAN_POINT('Ctrl Pts',(1.11895565834,-36.4799878332,-2.79941259037));
#68274=CARTESIAN_POINT('Ctrl Pts',(1.11895565834,-36.5742356128,-2.79941259037));
#68275=CARTESIAN_POINT('Ctrl Pts',(1.18794302831,-36.2742356128,-2.47960347752));
#68276=CARTESIAN_POINT('Ctrl Pts',(1.20872454331,-36.2742356128,-2.57156017536));
#68277=CARTESIAN_POINT('Ctrl Pts',(1.22950605832,-36.3112466293,-2.66351687319));
#68278=CARTESIAN_POINT('Ctrl Pts',(1.24593176322,-36.3857400536,-2.73619942694));
#68279=CARTESIAN_POINT('Ctrl Pts',(1.25409264508,-36.4799878332,-2.77231073775));
#68280=CARTESIAN_POINT('Ctrl Pts',(1.25409264508,-36.5742356128,-2.77231073775));
#68281=CARTESIAN_POINT('Ctrl Pts',(1.31515278454,-36.2742356128,-2.45004137538));
#68282=CARTESIAN_POINT('Ctrl Pts',(1.33816133022,-36.2742356128,-2.54148026436));
#68283=CARTESIAN_POINT('Ctrl Pts',(1.36116987589,-36.3112466293,-2.63291915334));
#68284=CARTESIAN_POINT('Ctrl Pts',(1.37935582534,-36.3857400536,-2.70519243109));
#68285=CARTESIAN_POINT('Ctrl Pts',(1.3883912601,-36.4799878332,-2.74110039882));
#68286=CARTESIAN_POINT('Ctrl Pts',(1.3883912601,-36.5742356128,-2.74110039882));
#68287=CARTESIAN_POINT('Ctrl Pts',(1.44143362741,-36.2742356128,-2.41663560271));
#68288=CARTESIAN_POINT('Ctrl Pts',(1.46665027818,-36.2742356128,-2.50748956127));
#68289=CARTESIAN_POINT('Ctrl Pts',(1.49186692895,-36.3112466293,-2.59834351983));
#68290=CARTESIAN_POINT('Ctrl Pts',(1.51179810201,-36.3857400536,-2.67015449813));
#68291=CARTESIAN_POINT('Ctrl Pts',(1.52170071978,-36.4799878332,-2.70583273481));
#68292=CARTESIAN_POINT('Ctrl Pts',(1.52170071978,-36.5742356128,-2.70583273481));
#68293=CARTESIAN_POINT('Ctrl Pts',(1.69185428337,-36.2742356128,-2.34222503069));
#68294=CARTESIAN_POINT('Ctrl Pts',(1.72143190971,-36.2742356128,-2.43178423883));
#68295=CARTESIAN_POINT('Ctrl Pts',(1.75100953605,-36.3112466293,-2.52134344697));
#68296=CARTESIAN_POINT('Ctrl Pts',(1.77438774757,-36.3857400536,-2.59213099598));
#68297=CARTESIAN_POINT('Ctrl Pts',(1.7860027921,-36.4799878332,-2.62730084419));
#68298=CARTESIAN_POINT('Ctrl Pts',(1.7860027921,-36.5742356128,-2.62730084419));
#68299=CARTESIAN_POINT('Ctrl Pts',(1.93730960461,-36.2742356128,-2.25284977591));
#68300=CARTESIAN_POINT('Ctrl Pts',(1.97117385257,-36.2742356128,-2.34084746769));
#68301=CARTESIAN_POINT('Ctrl Pts',(2.00503810053,-36.3112466293,-2.42884515947));
#68302=CARTESIAN_POINT('Ctrl Pts',(2.0318043325,-36.3857400536,-2.49839854512));
#68303=CARTESIAN_POINT('Ctrl Pts',(2.04510285375,-36.4799878332,-2.53295512846));
#68304=CARTESIAN_POINT('Ctrl Pts',(2.04510285375,-36.5742356128,-2.53295512846));
#68305=CARTESIAN_POINT('Ctrl Pts',(2.05867417483,-36.2742356128,-2.20445670509));
#68306=CARTESIAN_POINT('Ctrl Pts',(2.09464235556,-36.2742356128,-2.29161676797));
#68307=CARTESIAN_POINT('Ctrl Pts',(2.13061053629,-36.3112466293,-2.37877683084));
#68308=CARTESIAN_POINT('Ctrl Pts',(2.15904002711,-36.3857400536,-2.44766800768));
#68309=CARTESIAN_POINT('Ctrl Pts',(2.17316444997,-36.4799878332,-2.48189580202));
#68310=CARTESIAN_POINT('Ctrl Pts',(2.17316444997,-36.5742356128,-2.48189580202));
#68311=CARTESIAN_POINT('Ctrl Pts',(2.17843292253,-36.2742356128,-2.15245040014));
#68312=CARTESIAN_POINT('Ctrl Pts',(2.21651835677,-36.2742356128,-2.23869055108));
#68313=CARTESIAN_POINT('Ctrl Pts',(2.25460379102,-36.3112466293,-2.32493070202));
#68314=CARTESIAN_POINT('Ctrl Pts',(2.28470634408,-36.3857400536,-2.39309497682));
#68315=CARTESIAN_POINT('Ctrl Pts',(2.29966262492,-36.4799878332,-2.42696132644));
#68316=CARTESIAN_POINT('Ctrl Pts',(2.29966262492,-36.5742356128,-2.42696132644));
#68317=CARTESIAN_POINT('Ctrl Pts',(2.29653436395,-36.2742356128,-2.09683572989));
#68318=CARTESIAN_POINT('Ctrl Pts',(2.3366869803,-36.2742356128,-2.18210243716));
#68319=CARTESIAN_POINT('Ctrl Pts',(2.37683959666,-36.3112466293,-2.26736914443));
#68320=CARTESIAN_POINT('Ctrl Pts',(2.40857621579,-36.3857400536,-2.33476393111));
#68321=CARTESIAN_POINT('Ctrl Pts',(2.42434411136,-36.4799878332,-2.36824808876));
#68322=CARTESIAN_POINT('Ctrl Pts',(2.42434411136,-36.5742356128,-2.36824808876));
#68323=CARTESIAN_POINT('',(2.42434411094,-36.5742356128,-2.36824808793));
#68324=CARTESIAN_POINT('Origin',(2.2974382266538,-36.5721143196987,-2.09875482216244));
#68325=CARTESIAN_POINT('Origin',(0.445434424817657,-36.5742356128,1.43140361501688));
#68326=CARTESIAN_POINT('Ctrl Pts',(2.42434410765,-37.9742356128,-2.36824808142));
#68327=CARTESIAN_POINT('Ctrl Pts',(2.42434410765,-38.0684833925,-2.36824808142));
#68328=CARTESIAN_POINT('Ctrl Pts',(2.4085761387,-38.1627311721,-2.33476395847));
#68329=CARTESIAN_POINT('Ctrl Pts',(2.37683937187,-38.2372245964,-2.26736924161));
#68330=CARTESIAN_POINT('Ctrl Pts',(2.33668656866,-38.2742356129,-2.1821026227));
#68331=CARTESIAN_POINT('Ctrl Pts',(2.29653376547,-38.2742356128,-2.0968360038));
#68332=CARTESIAN_POINT('Ctrl Pts',(2.29966569663,-37.9742356128,-2.42695994895));
#68333=CARTESIAN_POINT('Ctrl Pts',(2.29966569667,-38.0684833925,-2.42695994893));
#68334=CARTESIAN_POINT('Ctrl Pts',(2.28470854164,-38.1627311723,-2.39309400964));
#68335=CARTESIAN_POINT('Ctrl Pts',(2.25460410565,-38.2372245966,-2.32493061899));
#68336=CARTESIAN_POINT('Ctrl Pts',(2.21651634095,-38.274235613,-2.23869156224));
#68337=CARTESIAN_POINT('Ctrl Pts',(2.17842857626,-38.2742356128,-2.15245250557));
#68338=CARTESIAN_POINT('Ctrl Pts',(2.17315794346,-37.9742356128,-2.48189872286));
#68339=CARTESIAN_POINT('Ctrl Pts',(2.17315794944,-38.0684833917,-2.48189872001));
#68340=CARTESIAN_POINT('Ctrl Pts',(2.15903493648,-38.1627311705,-2.44767026483));
#68341=CARTESIAN_POINT('Ctrl Pts',(2.13060846119,-38.2372245946,-2.37877767407));
#68342=CARTESIAN_POINT('Ctrl Pts',(2.09464401419,-38.2742356116,-2.29161586047));
#68343=CARTESIAN_POINT('Ctrl Pts',(2.05867956465,-38.2742356128,-2.20445404757));
#68344=CARTESIAN_POINT('Ctrl Pts',(2.04510265844,-37.9742356128,-2.53295494804));
#68345=CARTESIAN_POINT('Ctrl Pts',(2.04510267392,-38.068483392,-2.53295494205));
#68346=CARTESIAN_POINT('Ctrl Pts',(2.03180403214,-38.1627311711,-2.49839847555));
#68347=CARTESIAN_POINT('Ctrl Pts',(2.005037321,-38.2372245952,-2.42884538862));
#68348=CARTESIAN_POINT('Ctrl Pts',(1.97117254874,-38.2742356121,-2.3408480546));
#68349=CARTESIAN_POINT('Ctrl Pts',(1.9373077703,-38.2742356128,-2.25285072267));
#68350=CARTESIAN_POINT('Ctrl Pts',(1.78600167486,-37.9742356128,-2.62730149119));
#68351=CARTESIAN_POINT('Ctrl Pts',(1.78600169488,-38.0684833923,-2.62730148454));
#68352=CARTESIAN_POINT('Ctrl Pts',(1.77438683171,-38.1627311718,-2.59213150305));
#68353=CARTESIAN_POINT('Ctrl Pts',(1.75100917837,-38.2372245961,-2.5213436377));
#68354=CARTESIAN_POINT('Ctrl Pts',(1.72143215468,-38.2742356127,-2.43178405694));
#68355=CARTESIAN_POINT('Ctrl Pts',(1.69185512312,-38.2742356128,-2.34222447873));
#68356=CARTESIAN_POINT('Ctrl Pts',(1.52170151672,-37.9742356128,-2.70583218602));
#68357=CARTESIAN_POINT('Ctrl Pts',(1.52170152953,-38.0684833931,-2.70583218274));
#68358=CARTESIAN_POINT('Ctrl Pts',(1.51179878238,-38.1627311734,-2.67015406859));
#68359=CARTESIAN_POINT('Ctrl Pts',(1.49186711563,-38.2372245979,-2.59834339715));
#68360=CARTESIAN_POINT('Ctrl Pts',(1.46664992394,-38.2742356139,-2.50748980544));
#68361=CARTESIAN_POINT('Ctrl Pts',(1.44143272734,-38.2742356128,-2.41663621543));
#68362=CARTESIAN_POINT('Ctrl Pts',(1.38839422114,-37.9742356128,-2.74109975505));
#68363=CARTESIAN_POINT('Ctrl Pts',(1.38839422089,-38.0684833925,-2.74109975528));
#68364=CARTESIAN_POINT('Ctrl Pts',(1.37935818392,-38.1627311721,-2.70519190943));
#68365=CARTESIAN_POINT('Ctrl Pts',(1.36117170821,-38.2372245964,-2.63291873908));
#68366=CARTESIAN_POINT('Ctrl Pts',(1.33816220899,-38.2742356129,-2.5414800437));
#68367=CARTESIAN_POINT('Ctrl Pts',(1.31515270986,-38.2742356128,-2.45004134821));
#68368=CARTESIAN_POINT('Ctrl Pts',(1.25409290934,-37.9742356128,-2.77231068475));
#68369=CARTESIAN_POINT('Ctrl Pts',(1.25409290934,-38.0684833924,-2.77231068475));
#68370=CARTESIAN_POINT('Ctrl Pts',(1.24593217744,-38.1627311721,-2.73619934385));
#68371=CARTESIAN_POINT('Ctrl Pts',(1.22950631738,-38.2372245963,-2.66351682126));
#68372=CARTESIAN_POINT('Ctrl Pts',(1.20872479797,-38.2742356128,-2.57156012428));
#68373=CARTESIAN_POINT('Ctrl Pts',(1.18794327857,-38.2742356128,-2.47960342733));
#68374=CARTESIAN_POINT('Ctrl Pts',(1.11895565834,-37.9742356128,-2.79941259037));
#68375=CARTESIAN_POINT('Ctrl Pts',(1.11895565834,-38.0684833924,-2.79941259037));
#68376=CARTESIAN_POINT('Ctrl Pts',(1.1116779773,-38.1627311721,-2.7631241528));
#68377=CARTESIAN_POINT('Ctrl Pts',(1.09702992293,-38.2372245963,-2.69008508953));
#68378=CARTESIAN_POINT('Ctrl Pts',(1.07849746032,-38.2742356128,-2.59767734207));
#68379=CARTESIAN_POINT('Ctrl Pts',(1.05996499772,-38.2742356128,-2.50526959461));
#68380=CARTESIAN_POINT('',(2.42434411094,-37.9742356128,-2.36824808793));
#68381=CARTESIAN_POINT('Origin',(0.445434424817657,-37.9742356128,1.43140361501688));
#68382=CARTESIAN_POINT('Origin',(2.29743725625794,-37.9763568917663,-2.09875525922514));
#68383=CARTESIAN_POINT('Ctrl Pts',(1.11895565834,-37.9742356128,-2.79941259037));
#68384=CARTESIAN_POINT('Ctrl Pts',(1.11895565834,-36.2942356128,-2.79941259037));
#68385=CARTESIAN_POINT('Ctrl Pts',(1.38919794322,-37.9742356128,-2.7452152403));
#68386=CARTESIAN_POINT('Ctrl Pts',(1.38919794322,-36.2942356128,-2.7452152403));
#68387=CARTESIAN_POINT('Ctrl Pts',(1.65613520407,-37.9742356128,-2.67457823688));
#68388=CARTESIAN_POINT('Ctrl Pts',(1.65613520407,-36.2942356128,-2.67457823688));
#68389=CARTESIAN_POINT('Ctrl Pts',(1.91849016776,-37.9742356128,-2.58792345825));
#68390=CARTESIAN_POINT('Ctrl Pts',(1.91849016776,-36.2942356128,-2.58792345825));
#68391=CARTESIAN_POINT('Ctrl Pts',(2.1749855611,-37.9742356128,-2.48567278256));
#68392=CARTESIAN_POINT('Ctrl Pts',(2.1749855611,-36.2942356128,-2.48567278256));
#68393=CARTESIAN_POINT('Ctrl Pts',(2.42434411094,-37.9742356128,-2.36824808793));
#68394=CARTESIAN_POINT('Ctrl Pts',(2.42434411094,-36.2942356128,-2.36824808793));
#68395=CARTESIAN_POINT('',(2.42434411094,-37.2742356128,-2.36824808793));
#68396=CARTESIAN_POINT('Ctrl Pts',(2.29653416635,-36.2742356128,-2.09683582206));
#68397=CARTESIAN_POINT('Ctrl Pts',(2.33668684465,-36.2742356128,-2.18210250012));
#68398=CARTESIAN_POINT('Ctrl Pts',(2.37683952295,-36.3112466293,-2.26736917817));
#68399=CARTESIAN_POINT('Ctrl Pts',(2.40857619105,-36.3857400536,-2.33476394176));
#68400=CARTESIAN_POINT('Ctrl Pts',(2.42434411094,-36.4799878332,-2.36824808793));
#68401=CARTESIAN_POINT('Ctrl Pts',(2.42434411094,-36.5742356128,-2.36824808793));
#68402=CARTESIAN_POINT('Ctrl Pts',(2.95453073399,-36.2742356128,-1.78698061128));
#68403=CARTESIAN_POINT('Ctrl Pts',(3.00083493027,-36.2742356128,-1.86935049626));
#68404=CARTESIAN_POINT('Ctrl Pts',(3.04713912654,-36.3112466293,-1.95172038124));
#68405=CARTESIAN_POINT('Ctrl Pts',(3.08373795336,-36.3857400536,-2.01682552));
#68406=CARTESIAN_POINT('Ctrl Pts',(3.10192156845,-36.4799878332,-2.04917209841));
#68407=CARTESIAN_POINT('Ctrl Pts',(3.10192156845,-36.5742356128,-2.04917209841));
#68408=CARTESIAN_POINT('Ctrl Pts',(3.5952546957,-36.2742356128,-1.41294917537));
#68409=CARTESIAN_POINT('Ctrl Pts',(3.64373574115,-36.2742356128,-1.49338900213));
#68410=CARTESIAN_POINT('Ctrl Pts',(3.6922167866,-36.3112466293,-1.5738288289));
#68411=CARTESIAN_POINT('Ctrl Pts',(3.73053619354,-36.3857400536,-1.63740845094));
#68412=CARTESIAN_POINT('Ctrl Pts',(3.7495746563,-36.4799878332,-1.6689970964));
#68413=CARTESIAN_POINT('Ctrl Pts',(3.7495746563,-36.5742356128,-1.6689970964));
#68414=CARTESIAN_POINT('Ctrl Pts',(4.24448534634,-36.2742356128,-1.01869348797));
#68415=CARTESIAN_POINT('Ctrl Pts',(4.29909048777,-36.2742356128,-1.09736282407));
#68416=CARTESIAN_POINT('Ctrl Pts',(4.35369562921,-36.3112466293,-1.17603216016));
#68417=CARTESIAN_POINT('Ctrl Pts',(4.39685551792,-36.3857400536,-1.23821239064));
#68418=CARTESIAN_POINT('Ctrl Pts',(4.41829890989,-36.4799878332,-1.26910576216));
#68419=CARTESIAN_POINT('Ctrl Pts',(4.41829890989,-36.5742356128,-1.26910576216));
#68420=CARTESIAN_POINT('Ctrl Pts',(4.92993816697,-36.2742356128,-0.405284473542));
#68421=CARTESIAN_POINT('Ctrl Pts',(4.99982900549,-36.2742356128,-0.471480723113));
#68422=CARTESIAN_POINT('Ctrl Pts',(5.06971984401,-36.3112466293,-0.537676972684));
#68423=CARTESIAN_POINT('Ctrl Pts',(5.12496154763,-36.3857400536,-0.589998473204));
#68424=CARTESIAN_POINT('Ctrl Pts',(5.15240761552,-36.4799878332,-0.615993680209));
#68425=CARTESIAN_POINT('Ctrl Pts',(5.15240761552,-36.5742356128,-0.615993680209));
#68426=CARTESIAN_POINT('Ctrl Pts',(5.39693231373,-36.2742356128,0.342016557109));
#68427=CARTESIAN_POINT('Ctrl Pts',(5.4787021914,-36.2742356128,0.2948529986));
#68428=CARTESIAN_POINT('Ctrl Pts',(5.56047206907,-36.3112466293,0.247689440091));
#68429=CARTESIAN_POINT('Ctrl Pts',(5.62510296248,-36.3857400536,0.210411373802));
#68430=CARTESIAN_POINT('Ctrl Pts',(5.65721391827,-36.4799878332,0.191890287698));
#68431=CARTESIAN_POINT('Ctrl Pts',(5.65721391827,-36.5742356128,0.191890287698));
#68432=CARTESIAN_POINT('Ctrl Pts',(5.4810890824,-36.2742356128,0.496036554802));
#68433=CARTESIAN_POINT('Ctrl Pts',(5.56496873272,-36.2742356128,0.452739908435));
#68434=CARTESIAN_POINT('Ctrl Pts',(5.64884838304,-36.3112466293,0.409443262069));
#68435=CARTESIAN_POINT('Ctrl Pts',(5.71514684025,-36.3857400536,0.375221601448));
#68436=CARTESIAN_POINT('Ctrl Pts',(5.74808630186,-36.4799878332,0.358219049031));
#68437=CARTESIAN_POINT('Ctrl Pts',(5.74808630186,-36.5742356128,0.358219049031));
#68438=CARTESIAN_POINT('Ctrl Pts',(5.60372131748,-36.2742356128,0.754858335755));
#68439=CARTESIAN_POINT('Ctrl Pts',(5.69047130637,-36.2742356128,0.717714053116));
#68440=CARTESIAN_POINT('Ctrl Pts',(5.77722129526,-36.3112466293,0.680569770476));
#68441=CARTESIAN_POINT('Ctrl Pts',(5.84578846738,-36.3857400536,0.651210937785));
#68442=CARTESIAN_POINT('Ctrl Pts',(5.87985510838,-36.4799878332,0.636624411961));
#68443=CARTESIAN_POINT('Ctrl Pts',(5.87985510838,-36.5742356128,0.636624411961));
#68444=CARTESIAN_POINT('Ctrl Pts',(5.70660931534,-36.2742356128,1.02615041344));
#68445=CARTESIAN_POINT('Ctrl Pts',(5.79530810838,-36.2742356128,0.994188908045));
#68446=CARTESIAN_POINT('Ctrl Pts',(5.88400690142,-36.3112466293,0.962227402652));
#68447=CARTESIAN_POINT('Ctrl Pts',(5.95411440796,-36.3857400536,0.936965035973));
#68448=CARTESIAN_POINT('Ctrl Pts',(5.98894634251,-36.4799878332,0.924413781998));
#68449=CARTESIAN_POINT('Ctrl Pts',(5.98894634251,-36.5742356128,0.924413781998));
#68450=CARTESIAN_POINT('Ctrl Pts',(5.74376248036,-36.2742356128,1.13296600714));
#68451=CARTESIAN_POINT('Ctrl Pts',(5.83306897758,-36.2742356128,1.10277988931));
#68452=CARTESIAN_POINT('Ctrl Pts',(5.92237547479,-36.3112466293,1.07259377148));
#68453=CARTESIAN_POINT('Ctrl Pts',(5.99296331053,-36.3857400536,1.04873466986));
#68454=CARTESIAN_POINT('Ctrl Pts',(6.02803389001,-36.4799878332,1.03688060983));
#68455=CARTESIAN_POINT('Ctrl Pts',(6.02803389001,-36.5742356128,1.03688060983));
#68456=CARTESIAN_POINT('Ctrl Pts',(5.79918814733,-36.2742356128,1.3044656396));
#68457=CARTESIAN_POINT('Ctrl Pts',(5.88927282406,-36.2742356128,1.276721735));
#68458=CARTESIAN_POINT('Ctrl Pts',(5.97935750079,-36.3112466293,1.24897783041));
#68459=CARTESIAN_POINT('Ctrl Pts',(6.0505604095,-36.3857400536,1.22704905448));
#68460=CARTESIAN_POINT('Ctrl Pts',(6.08593657929,-36.4799878332,1.21615404846));
#68461=CARTESIAN_POINT('Ctrl Pts',(6.08593657929,-36.5742356128,1.21615404846));
#68462=CARTESIAN_POINT('Ctrl Pts',(5.85112053171,-36.2742356128,1.48092066179));
#68463=CARTESIAN_POINT('Ctrl Pts',(5.94165101522,-36.2742356128,1.45470447779));
#68464=CARTESIAN_POINT('Ctrl Pts',(6.03218149873,-36.3112466293,1.42848829379));
#68465=CARTESIAN_POINT('Ctrl Pts',(6.10373677297,-36.3857400536,1.40776702777));
#68466=CARTESIAN_POINT('Ctrl Pts',(6.13928801073,-36.4799878332,1.39747195633));
#68467=CARTESIAN_POINT('Ctrl Pts',(6.13928801073,-36.5742356128,1.39747195633));
#68468=CARTESIAN_POINT('Ctrl Pts',(5.86993279335,-36.2742356128,1.54652856629));
#68469=CARTESIAN_POINT('Ctrl Pts',(5.96057340692,-36.2742356128,1.52070063308));
#68470=CARTESIAN_POINT('Ctrl Pts',(6.05121402049,-36.3112466293,1.49487269988));
#68471=CARTESIAN_POINT('Ctrl Pts',(6.12285634131,-36.3857400536,1.47445830642));
#68472=CARTESIAN_POINT('Ctrl Pts',(6.15845082724,-36.4799878332,1.4643157015));
#68473=CARTESIAN_POINT('Ctrl Pts',(6.15845082724,-36.5742356128,1.4643157015));
#68474=CARTESIAN_POINT('Ctrl Pts',(5.90547870352,-36.2742356128,1.67276409439));
#68475=CARTESIAN_POINT('Ctrl Pts',(5.99629775732,-36.2742356128,1.6475719299));
#68476=CARTESIAN_POINT('Ctrl Pts',(6.08711681113,-36.3112466293,1.62237976542));
#68477=CARTESIAN_POINT('Ctrl Pts',(6.15890017139,-36.3857400536,1.60246788439));
#68478=CARTESIAN_POINT('Ctrl Pts',(6.19456473032,-36.4799878332,1.59257494429));
#68479=CARTESIAN_POINT('Ctrl Pts',(6.19456473032,-36.5742356128,1.59257494429));
#68480=CARTESIAN_POINT('Ctrl Pts',(5.94051748703,-36.2742356128,1.79907562584));
#68481=CARTESIAN_POINT('Ctrl Pts',(6.03131527525,-36.2742356128,1.77381004956));
#68482=CARTESIAN_POINT('Ctrl Pts',(6.12211306348,-36.3112466293,1.74854447327));
#68483=CARTESIAN_POINT('Ctrl Pts',(6.19387961533,-36.3857400536,1.72857456759));
#68484=CARTESIAN_POINT('Ctrl Pts',(6.22953582338,-36.4799878332,1.71865279873));
#68485=CARTESIAN_POINT('Ctrl Pts',(6.22953582338,-36.5742356128,1.71865279873));
#68486=CARTESIAN_POINT('Ctrl Pts',(5.95837521227,-36.2742356128,1.86312440916));
#68487=CARTESIAN_POINT('Ctrl Pts',(6.04910326111,-36.2742356128,1.8376090522));
#68488=CARTESIAN_POINT('Ctrl Pts',(6.13983130995,-36.3112466293,1.81209369523));
#68489=CARTESIAN_POINT('Ctrl Pts',(6.21154274281,-36.3857400536,1.79192636818));
#68490=CARTESIAN_POINT('Ctrl Pts',(6.24717156127,-36.4799878332,1.78190650545));
#68491=CARTESIAN_POINT('Ctrl Pts',(6.24717156127,-36.5742356128,1.78190650545));
#68492=CARTESIAN_POINT('Ctrl Pts',(6.01765623996,-36.2742356128,2.07213314299));
#68493=CARTESIAN_POINT('Ctrl Pts',(6.10806285924,-36.2742356128,2.04545736833));
#68494=CARTESIAN_POINT('Ctrl Pts',(6.19846947852,-36.3112466293,2.01878159367));
#68495=CARTESIAN_POINT('Ctrl Pts',(6.26992684338,-36.3857400536,1.99769705348));
#68496=CARTESIAN_POINT('Ctrl Pts',(6.30542944689,-36.4799878332,1.98722151502));
#68497=CARTESIAN_POINT('Ctrl Pts',(6.30542944689,-36.5742356128,1.98722151502));
#68498=CARTESIAN_POINT('Ctrl Pts',(6.08567485884,-36.2742356128,2.29020798204));
#68499=CARTESIAN_POINT('Ctrl Pts',(6.17503220776,-36.2742356128,2.26008450139));
#68500=CARTESIAN_POINT('Ctrl Pts',(6.26438955668,-36.3112466293,2.22996102075));
#68501=CARTESIAN_POINT('Ctrl Pts',(6.33501760237,-36.3857400536,2.20615146186));
#68502=CARTESIAN_POINT('Ctrl Pts',(6.37010813448,-36.4799878332,2.19432196508));
#68503=CARTESIAN_POINT('Ctrl Pts',(6.37010813448,-36.5742356128,2.19432196508));
#68504=CARTESIAN_POINT('Ctrl Pts',(6.13676392343,-36.2742356128,2.43482563093));
#68505=CARTESIAN_POINT('Ctrl Pts',(6.2249876692,-36.2742356128,2.40121723527));
#68506=CARTESIAN_POINT('Ctrl Pts',(6.31321141497,-36.3112466293,2.3676088396));
#68507=CARTESIAN_POINT('Ctrl Pts',(6.38294338684,-36.3857400536,2.34104466316));
#68508=CARTESIAN_POINT('Ctrl Pts',(6.41758882819,-36.4799878332,2.32784678495));
#68509=CARTESIAN_POINT('Ctrl Pts',(6.41758882819,-36.5742356128,2.32784678495));
#68510=CARTESIAN_POINT('Ctrl Pts',(6.19859174917,-36.2742356128,2.58091129692));
#68511=CARTESIAN_POINT('Ctrl Pts',(6.28484385346,-36.2742356128,2.54230495555));
#68512=CARTESIAN_POINT('Ctrl Pts',(6.37109595776,-36.3112466293,2.50369861417));
#68513=CARTESIAN_POINT('Ctrl Pts',(6.43926964058,-36.3857400536,2.47318424312));
#68514=CARTESIAN_POINT('Ctrl Pts',(6.47314072418,-36.4799878332,2.45802349563));
#68515=CARTESIAN_POINT('Ctrl Pts',(6.47314072418,-36.5742356128,2.45802349563));
#68516=CARTESIAN_POINT('Ctrl Pts',(6.27496287808,-36.2742356128,2.72284550202));
#68517=CARTESIAN_POINT('Ctrl Pts',(6.35795875815,-36.2742356128,2.67818760544));
#68518=CARTESIAN_POINT('Ctrl Pts',(6.44095463823,-36.3112466293,2.63352970885));
#68519=CARTESIAN_POINT('Ctrl Pts',(6.50655456359,-36.3857400536,2.59823211721));
#68520=CARTESIAN_POINT('Ctrl Pts',(6.53914696948,-36.4799878332,2.58069500223));
#68521=CARTESIAN_POINT('Ctrl Pts',(6.53914696948,-36.5742356128,2.58069500223));
#68522=CARTESIAN_POINT('Ctrl Pts',(2.42434411094,-36.5742356128,-2.36824808793));
#68523=CARTESIAN_POINT('Ctrl Pts',(2.54136162563,-36.5742356128,-2.31314371739));
#68524=CARTESIAN_POINT('Ctrl Pts',(2.65752099957,-36.5742356128,-2.25621686612));
#68525=CARTESIAN_POINT('Ctrl Pts',(2.77407974247,-36.5742356128,-2.1971394748));
#68526=CARTESIAN_POINT('Ctrl Pts',(3.24315352432,-36.5742356128,-1.95213056688));
#68527=CARTESIAN_POINT('Ctrl Pts',(3.70906725491,-36.5742356128,-1.67871445412));
#68528=CARTESIAN_POINT('Ctrl Pts',(4.05512009518,-36.5742356128,-1.45762154475));
#68529=CARTESIAN_POINT('Ctrl Pts',(4.83098837637,-36.5742356128,-0.890342468227));
#68530=CARTESIAN_POINT('Ctrl Pts',(5.472362609,-36.5742356128,-0.180892800224));
#68531=CARTESIAN_POINT('Ctrl Pts',(5.76642241654,-36.5742356128,0.2786624797));
#68532=CARTESIAN_POINT('Ctrl Pts',(6.00694923868,-36.5742356128,0.922077058536));
#68533=CARTESIAN_POINT('Ctrl Pts',(6.19138019969,-36.5742356128,1.57972239002));
#68534=CARTESIAN_POINT('Ctrl Pts',(6.22058475326,-36.5742356128,1.68729406867));
#68535=CARTESIAN_POINT('Ctrl Pts',(6.29416488239538,-36.5742356128,1.9543061191784));
#68536=CARTESIAN_POINT('Ctrl Pts',(6.37839829623924,-36.5742356128,2.2167883668313));
#68537=CARTESIAN_POINT('Ctrl Pts',(6.4240234576883,-36.5742356128,2.3426643448704));
#68538=CARTESIAN_POINT('Ctrl Pts',(6.47656234367984,-36.5742356128,2.46438238106866));
#68539=CARTESIAN_POINT('Ctrl Pts',(6.53914700243265,-36.5742356128,2.58069506476114));
#68540=CARTESIAN_POINT('Ctrl Pts',(6.53914703241,-37.9742356128,2.58069512031));
#68541=CARTESIAN_POINT('Ctrl Pts',(6.5391470324,-38.0684833925,2.58069512029));
#68542=CARTESIAN_POINT('Ctrl Pts',(6.50655461068,-38.1627311721,2.59823220638));
#68543=CARTESIAN_POINT('Ctrl Pts',(6.44095465346,-38.2372245963,2.63352973988));
#68544=CARTESIAN_POINT('Ctrl Pts',(6.35795873309,-38.2742356128,2.67818756293));
#68545=CARTESIAN_POINT('Ctrl Pts',(6.27496281272,-38.2742356128,2.72284538598));
#68546=CARTESIAN_POINT('Ctrl Pts',(6.47749928031,-37.9742356128,2.46612372063));
#68547=CARTESIAN_POINT('Ctrl Pts',(6.47749928325,-38.0684833921,2.46612372592));
#68548=CARTESIAN_POINT('Ctrl Pts',(6.44371355209,-38.1627311714,2.4814430712));
#68549=CARTESIAN_POINT('Ctrl Pts',(6.37571165731,-38.2372245955,2.51227664714));
#68550=CARTESIAN_POINT('Ctrl Pts',(6.2896768948,-38.2742356123,2.55128684019));
#68551=CARTESIAN_POINT('Ctrl Pts',(6.20364213078,-38.2742356128,2.59029703093));
#68552=CARTESIAN_POINT('Ctrl Pts',(6.4250505295,-37.9742356128,2.34529109436));
#68553=CARTESIAN_POINT('Ctrl Pts',(6.4250505205,-38.0684834574,2.34529107738));
#68554=CARTESIAN_POINT('Ctrl Pts',(6.39050752202,-38.1627313021,2.35875081294));
#68555=CARTESIAN_POINT('Ctrl Pts',(6.3209817521,-38.2372247495,2.38584206978));
#68556=CARTESIAN_POINT('Ctrl Pts',(6.23301891757,-38.2742357149,2.4201173123));
#68557=CARTESIAN_POINT('Ctrl Pts',(6.14505612298,-38.2742356128,2.45439254437));
#68558=CARTESIAN_POINT('Ctrl Pts',(6.37923785733,-37.9742356128,2.21935750204));
#68559=CARTESIAN_POINT('Ctrl Pts',(6.37923785229,-38.0684834205,2.21935748159));
#68560=CARTESIAN_POINT('Ctrl Pts',(6.34424285411,-38.1627312282,2.23147400682));
#68561=CARTESIAN_POINT('Ctrl Pts',(6.27380710482,-38.2372246625,2.25586132033));
#68562=CARTESIAN_POINT('Ctrl Pts',(6.18469305765,-38.274235657,2.28671576875));
#68563=CARTESIAN_POINT('Ctrl Pts',(6.09557902928,-38.2742356128,2.31757022073));
#68564=CARTESIAN_POINT('Ctrl Pts',(6.29255842824,-37.9742356128,1.94958030449));
#68565=CARTESIAN_POINT('Ctrl Pts',(6.29255843379,-38.0684833616,1.94958032698));
#68566=CARTESIAN_POINT('Ctrl Pts',(6.25694629473,-38.1627311103,1.95971958966));
#68567=CARTESIAN_POINT('Ctrl Pts',(6.18526848373,-38.2372245236,1.98012731791));
#68568=CARTESIAN_POINT('Ctrl Pts',(6.09458293312,-38.2742355643,2.00594677005));
#68569=CARTESIAN_POINT('Ctrl Pts',(6.00389736185,-38.2742356128,2.03176621828));
#68570=CARTESIAN_POINT('Ctrl Pts',(6.21629158074,-37.9742356128,1.67179392517));
#68571=CARTESIAN_POINT('Ctrl Pts',(6.21629157465,-38.0684834264,1.67179390044));
#68572=CARTESIAN_POINT('Ctrl Pts',(6.18059131343,-38.16273124,1.68154041674));
#68573=CARTESIAN_POINT('Ctrl Pts',(6.10873604958,-38.2372246763,1.70115751673));
#68574=CARTESIAN_POINT('Ctrl Pts',(6.01782606333,-38.2742356662,1.72597678277));
#68575=CARTESIAN_POINT('Ctrl Pts',(5.92691609981,-38.2742356128,1.75079605312));
#68576=CARTESIAN_POINT('Ctrl Pts',(6.18335047849,-37.9742356128,1.55015139283));
#68577=CARTESIAN_POINT('Ctrl Pts',(6.18335048466,-38.068483409,1.55015141338));
#68578=CARTESIAN_POINT('Ctrl Pts',(6.1476764427,-38.1627312051,1.56001197253));
#68579=CARTESIAN_POINT('Ctrl Pts',(6.07587398952,-38.2372246353,1.57985865724));
#68580=CARTESIAN_POINT('Ctrl Pts',(5.98503078164,-38.2742356388,1.60496832085));
#68581=CARTESIAN_POINT('Ctrl Pts',(5.89418758109,-38.2742356128,1.63007797337));
#68582=CARTESIAN_POINT('Ctrl Pts',(6.10683421874,-37.9742356128,1.27934110155));
#68583=CARTESIAN_POINT('Ctrl Pts',(6.10683421362,-38.0684833787,1.2793410845));
#68584=CARTESIAN_POINT('Ctrl Pts',(6.07133589713,-38.1627311446,1.28985606578));
#68585=CARTESIAN_POINT('Ctrl Pts',(5.99988714566,-38.237224564,1.31101997322));
#68586=CARTESIAN_POINT('Ctrl Pts',(5.90949143082,-38.2742355913,1.33779619135));
#68587=CARTESIAN_POINT('Ctrl Pts',(5.81909570989,-38.2742356128,1.36457241864));
#68588=CARTESIAN_POINT('Ctrl Pts',(6.02154757341,-37.9742356128,1.0171856396));
#68589=CARTESIAN_POINT('Ctrl Pts',(6.02154757766,-38.0684834038,1.01718565375));
#68590=CARTESIAN_POINT('Ctrl Pts',(5.98651519,-38.1627311948,1.02915949851));
#68591=CARTESIAN_POINT('Ctrl Pts',(5.91600421823,-38.2372246232,1.05325967438));
#68592=CARTESIAN_POINT('Ctrl Pts',(5.82679497009,-38.2742356307,1.08375078668));
#68593=CARTESIAN_POINT('Ctrl Pts',(5.737585727,-38.2742356128,1.11424189141));
#68594=CARTESIAN_POINT('Ctrl Pts',(5.97900661099,-37.9742356128,0.896224423713));
#68595=CARTESIAN_POINT('Ctrl Pts',(5.97900661569,-38.0684834269,0.896224436759));
#68596=CARTESIAN_POINT('Ctrl Pts',(5.94423871805,-38.162731241,0.908957424316));
#68597=CARTESIAN_POINT('Ctrl Pts',(5.87426009442,-38.2372246775,0.934585556151));
#68598=CARTESIAN_POINT('Ctrl Pts',(5.78572437213,-38.274235667,0.967009808905));
#68599=CARTESIAN_POINT('Ctrl Pts',(5.69718866798,-38.2742356128,0.999434049256));
#68600=CARTESIAN_POINT('Ctrl Pts',(5.88756297838,-37.9742356128,0.659856731438));
#68601=CARTESIAN_POINT('Ctrl Pts',(5.88756298491,-38.0684834275,0.659856746387));
#68602=CARTESIAN_POINT('Ctrl Pts',(5.85345466069,-38.1627312422,0.674306677198));
#68603=CARTESIAN_POINT('Ctrl Pts',(5.78480358285,-38.2372246789,0.703390562944));
#68604=CARTESIAN_POINT('Ctrl Pts',(5.69794744689,-38.2742356679,0.740186972418));
#68605=CARTESIAN_POINT('Ctrl Pts',(5.61109132821,-38.2742356128,0.776983367386));
#68606=CARTESIAN_POINT('Ctrl Pts',(5.78044949711,-37.9742356128,0.430172441648));
#68607=CARTESIAN_POINT('Ctrl Pts',(5.78044950152,-38.0684834047,0.430172449852));
#68608=CARTESIAN_POINT('Ctrl Pts',(5.74724282873,-38.1627311966,0.44656967303));
#68609=CARTESIAN_POINT('Ctrl Pts',(5.68040654018,-38.2372246253,0.47957295341));
#68610=CARTESIAN_POINT('Ctrl Pts',(5.59584643675,-38.2742356321,0.521328119811));
#68611=CARTESIAN_POINT('Ctrl Pts',(5.51128633822,-38.2742356128,0.56308327929));
#68612=CARTESIAN_POINT('Ctrl Pts',(5.7226529197,-37.9742356128,0.317367361304));
#68613=CARTESIAN_POINT('Ctrl Pts',(5.72265292242,-38.068483393,0.317367365818));
#68614=CARTESIAN_POINT('Ctrl Pts',(5.68995600371,-38.1627311732,0.334765690655));
#68615=CARTESIAN_POINT('Ctrl Pts',(5.62414571793,-38.2372245977,0.369783928543));
#68616=CARTESIAN_POINT('Ctrl Pts',(5.54088369215,-38.2742356138,0.414088388794));
#68617=CARTESIAN_POINT('Ctrl Pts',(5.4576216655,-38.2742356128,0.458392846952));
#68618=CARTESIAN_POINT('Ctrl Pts',(5.56080084046,-37.9742356128,0.0295320933249));
#68619=CARTESIAN_POINT('Ctrl Pts',(5.56080083609,-38.0684833915,0.0295320860792));
#68620=CARTESIAN_POINT('Ctrl Pts',(5.52957060213,-38.1627311702,0.0495393442441));
#68621=CARTESIAN_POINT('Ctrl Pts',(5.46671237524,-38.2372245941,0.089808691663));
#68622=CARTESIAN_POINT('Ctrl Pts',(5.38718524665,-38.2742356113,0.140756771766));
#68623=CARTESIAN_POINT('Ctrl Pts',(5.30765811944,-38.2742356128,0.191704855228));
#68624=CARTESIAN_POINT('Ctrl Pts',(5.37029202866,-37.9742356128,-0.241067403666));
#68625=CARTESIAN_POINT('Ctrl Pts',(5.37029203567,-38.068483394,-0.241067392035));
#68626=CARTESIAN_POINT('Ctrl Pts',(5.34079929298,-38.1627311751,-0.218590865746));
#68627=CARTESIAN_POINT('Ctrl Pts',(5.2814381653,-38.2372245999,-0.17335155271));
#68628=CARTESIAN_POINT('Ctrl Pts',(5.2063354988,-38.2742356152,-0.116115572303));
#68629=CARTESIAN_POINT('Ctrl Pts',(5.13123283009,-38.2742356128,-0.0588795972884));
#68630=CARTESIAN_POINT('Ctrl Pts',(5.24251980415,-37.9742356128,-0.400329171328));
#68631=CARTESIAN_POINT('Ctrl Pts',(5.24251981319,-38.0684833825,-0.400329163319));
#68632=CARTESIAN_POINT('Ctrl Pts',(5.21414835053,-38.1627311521,-0.376472093618));
#68633=CARTESIAN_POINT('Ctrl Pts',(5.15704406285,-38.2372245728,-0.328454107043));
#68634=CARTESIAN_POINT('Ctrl Pts',(5.08479670601,-38.2742355971,-0.267702591492));
#68635=CARTESIAN_POINT('Ctrl Pts',(5.01254934105,-38.2742356128,-0.206951074935));
#68636=CARTESIAN_POINT('Ctrl Pts',(4.6934087233,-37.9742356128,-1.00944907659));
#68637=CARTESIAN_POINT('Ctrl Pts',(4.6934086961,-38.0684834225,-1.00944910069));
#68638=CARTESIAN_POINT('Ctrl Pts',(4.66949795797,-38.1627312322,-0.980685909202));
#68639=CARTESIAN_POINT('Ctrl Pts',(4.6213719682,-38.2372246672,-0.922793157139));
#68640=CARTESIAN_POINT('Ctrl Pts',(4.56048383437,-38.2742356601,-0.84954825045));
#68641=CARTESIAN_POINT('Ctrl Pts',(4.49959572501,-38.2742356128,-0.776303346788));
#68642=CARTESIAN_POINT('Ctrl Pts',(4.02409822752,-37.9742356128,-1.50218108799));
#68643=CARTESIAN_POINT('Ctrl Pts',(4.02409830939,-38.0684833019,-1.50218101545));
#68644=CARTESIAN_POINT('Ctrl Pts',(4.00389313666,-38.1627309911,-1.47102303591));
#68645=CARTESIAN_POINT('Ctrl Pts',(3.96322537228,-38.2372243831,-1.40831031261));
#68646=CARTESIAN_POINT('Ctrl Pts',(3.91177314147,-38.2742354707,-1.3289672931));
#68647=CARTESIAN_POINT('Ctrl Pts',(3.860320837,-38.2742356128,-1.24962426449));
#68648=CARTESIAN_POINT('Ctrl Pts',(3.49329943878,-37.9742356128,-1.81694867414));
#68649=CARTESIAN_POINT('Ctrl Pts',(3.49329940337,-38.0684833917,-1.81694869081));
#68650=CARTESIAN_POINT('Ctrl Pts',(3.4746893405,-38.1627311706,-1.78496313544));
#68651=CARTESIAN_POINT('Ctrl Pts',(3.43723215534,-38.2372245946,-1.72058465543));
#68652=CARTESIAN_POINT('Ctrl Pts',(3.38984202793,-38.2742356117,-1.63913410317));
#68653=CARTESIAN_POINT('Ctrl Pts',(3.34245191658,-38.2742356128,-1.55768354279));
#68654=CARTESIAN_POINT('Ctrl Pts',(2.96849813462,-37.9742356128,-2.11200213165));
#68655=CARTESIAN_POINT('Ctrl Pts',(2.96849813462,-38.0684833924,-2.11200213165));
#68656=CARTESIAN_POINT('Ctrl Pts',(2.9507901825,-38.1627311721,-2.07943156023));
#68657=CARTESIAN_POINT('Ctrl Pts',(2.91514879128,-38.2372245963,-2.01387555828));
#68658=CARTESIAN_POINT('Ctrl Pts',(2.8700559069,-38.2742356128,-1.93093525801));
#68659=CARTESIAN_POINT('Ctrl Pts',(2.82496302107,-38.2742356128,-1.84799495842));
#68660=CARTESIAN_POINT('Ctrl Pts',(2.42434411094,-37.9742356128,-2.36824808793));
#68661=CARTESIAN_POINT('Ctrl Pts',(2.42434411094,-38.0684833924,-2.36824808793));
#68662=CARTESIAN_POINT('Ctrl Pts',(2.40857619105,-38.1627311721,-2.33476394176));
#68663=CARTESIAN_POINT('Ctrl Pts',(2.37683952295,-38.2372245963,-2.26736917817));
#68664=CARTESIAN_POINT('Ctrl Pts',(2.33668684465,-38.2742356128,-2.18210250012));
#68665=CARTESIAN_POINT('Ctrl Pts',(2.29653416635,-38.2742356128,-2.09683582206));
#68666=CARTESIAN_POINT('Ctrl Pts',(2.42434411094,-37.9742356128,-2.36824808793));
#68667=CARTESIAN_POINT('Ctrl Pts',(2.96849813462,-37.9742356128005,-2.11200213165));
#68668=CARTESIAN_POINT('Ctrl Pts',(3.49329943878,-37.9742356128005,-1.81694867414));
#68669=CARTESIAN_POINT('Ctrl Pts',(4.02409822752,-37.9742356128005,-1.50218108799));
#68670=CARTESIAN_POINT('Ctrl Pts',(4.6934087233,-37.9742356128005,-1.00944907659));
#68671=CARTESIAN_POINT('Ctrl Pts',(5.24251980415,-37.9742356128005,-0.400329171328));
#68672=CARTESIAN_POINT('Ctrl Pts',(5.37029202866,-37.9742356128005,-0.241067403666));
#68673=CARTESIAN_POINT('Ctrl Pts',(5.56080084046,-37.9742356128005,0.0295320933249));
#68674=CARTESIAN_POINT('Ctrl Pts',(5.7226529197,-37.9742356128005,0.317367361304));
#68675=CARTESIAN_POINT('Ctrl Pts',(5.78044949711,-37.9742356128005,0.430172441648));
#68676=CARTESIAN_POINT('Ctrl Pts',(5.88756297838,-37.9742356128005,0.659856731438));
#68677=CARTESIAN_POINT('Ctrl Pts',(5.97900661099,-37.9742356128005,0.896224423713));
#68678=CARTESIAN_POINT('Ctrl Pts',(6.02154757341,-37.9742356128005,1.0171856396));
#68679=CARTESIAN_POINT('Ctrl Pts',(6.10683421874,-37.9742356128005,1.27934110155));
#68680=CARTESIAN_POINT('Ctrl Pts',(6.18335047849,-37.9742356128005,1.55015139283));
#68681=CARTESIAN_POINT('Ctrl Pts',(6.21629158074,-37.9742356128005,1.67179392517));
#68682=CARTESIAN_POINT('Ctrl Pts',(6.29255842824,-37.9742356128005,1.94958030449));
#68683=CARTESIAN_POINT('Ctrl Pts',(6.37923785733,-37.9742356128005,2.21935750204));
#68684=CARTESIAN_POINT('Ctrl Pts',(6.4250505295,-37.9742356128005,2.34529109436));
#68685=CARTESIAN_POINT('Ctrl Pts',(6.47749928031,-37.9742356128005,2.46612372063));
#68686=CARTESIAN_POINT('Ctrl Pts',(6.53914701908,-37.9742356128,2.5806950957));
#68687=CARTESIAN_POINT('Ctrl Pts',(2.42434411094,-37.9742356128,-2.36824808793));
#68688=CARTESIAN_POINT('Ctrl Pts',(2.42434411094,-36.2942356128,-2.36824808793));
#68689=CARTESIAN_POINT('Ctrl Pts',(2.54136162563,-37.9742356128,-2.31314371739));
#68690=CARTESIAN_POINT('Ctrl Pts',(2.54136162563,-36.2942356128,-2.31314371739));
#68691=CARTESIAN_POINT('Ctrl Pts',(2.65752099957,-37.9742356128,-2.25621686612));
#68692=CARTESIAN_POINT('Ctrl Pts',(2.65752099957,-36.2942356128,-2.25621686612));
#68693=CARTESIAN_POINT('Ctrl Pts',(2.77407974247,-37.9742356128,-2.1971394748));
#68694=CARTESIAN_POINT('Ctrl Pts',(2.77407974247,-36.2942356128,-2.1971394748));
#68695=CARTESIAN_POINT('Ctrl Pts',(3.24315352432,-37.9742356128,-1.95213056688));
#68696=CARTESIAN_POINT('Ctrl Pts',(3.24315352432,-36.2942356128,-1.95213056688));
#68697=CARTESIAN_POINT('Ctrl Pts',(3.70906725491,-37.9742356128,-1.67871445412));
#68698=CARTESIAN_POINT('Ctrl Pts',(3.70906725491,-36.2942356128,-1.67871445412));
#68699=CARTESIAN_POINT('Ctrl Pts',(4.05512009518,-37.9742356128,-1.45762154475));
#68700=CARTESIAN_POINT('Ctrl Pts',(4.05512009518,-36.2942356128,-1.45762154475));
#68701=CARTESIAN_POINT('Ctrl Pts',(4.83098837637,-37.9742356128,-0.890342468227));
#68702=CARTESIAN_POINT('Ctrl Pts',(4.83098837637,-36.2942356128,-0.890342468227));
#68703=CARTESIAN_POINT('Ctrl Pts',(5.472362609,-37.9742356128,-0.180892800224));
#68704=CARTESIAN_POINT('Ctrl Pts',(5.472362609,-36.2942356128,-0.180892800224));
#68705=CARTESIAN_POINT('Ctrl Pts',(5.76642241654,-37.9742356128,0.2786624797));
#68706=CARTESIAN_POINT('Ctrl Pts',(5.76642241654,-36.2942356128,0.2786624797));
#68707=CARTESIAN_POINT('Ctrl Pts',(6.00694923868,-37.9742356128,0.922077058536));
#68708=CARTESIAN_POINT('Ctrl Pts',(6.00694923868,-36.2942356128,0.922077058536));
#68709=CARTESIAN_POINT('Ctrl Pts',(6.19138019969,-37.9742356128,1.57972239002));
#68710=CARTESIAN_POINT('Ctrl Pts',(6.19138019969,-36.2942356128,1.57972239002));
#68711=CARTESIAN_POINT('Ctrl Pts',(6.22058475326,-37.9742356128,1.68729406867));
#68712=CARTESIAN_POINT('Ctrl Pts',(6.22058475326,-36.2942356128,1.68729406867));
#68713=CARTESIAN_POINT('Ctrl Pts',(6.2941648843,-37.9742356128,1.95430612609));
#68714=CARTESIAN_POINT('Ctrl Pts',(6.2941648843,-36.2942356128,1.95430612609));
#68715=CARTESIAN_POINT('Ctrl Pts',(6.3783983006,-37.9742356128,2.21678838042));
#68716=CARTESIAN_POINT('Ctrl Pts',(6.3783983006,-36.2942356128,2.21678838042));
#68717=CARTESIAN_POINT('Ctrl Pts',(6.42402346497,-37.9742356128,2.34266436496));
#68718=CARTESIAN_POINT('Ctrl Pts',(6.42402346497,-36.2942356128,2.34266436496));
#68719=CARTESIAN_POINT('Ctrl Pts',(6.47656235486,-37.9742356128,2.46438240697));
#68720=CARTESIAN_POINT('Ctrl Pts',(6.47656235486,-36.2942356128,2.46438240697));
#68721=CARTESIAN_POINT('Ctrl Pts',(6.53914701908,-37.9742356128,2.5806950957));
#68722=CARTESIAN_POINT('Ctrl Pts',(6.53914701908,-36.2942356128,2.5806950957));
#68723=CARTESIAN_POINT('Ctrl Pts',(6.62478636278,-36.5742356128,4.12129363314));
#68724=CARTESIAN_POINT('Ctrl Pts',(6.62478636278,-36.4799878332,4.12129363314));
#68725=CARTESIAN_POINT('Ctrl Pts',(6.64533881083,-36.3857400536,4.09051357105));
#68726=CARTESIAN_POINT('Ctrl Pts',(6.68670547342,-36.3112466293,4.02856141623));
#68727=CARTESIAN_POINT('Ctrl Pts',(6.7390418526,-36.2742356128,3.95018063176));
#68728=CARTESIAN_POINT('Ctrl Pts',(6.79137823178,-36.2742356128,3.87179984728));
#68729=CARTESIAN_POINT('Ctrl Pts',(6.98489076396,-36.5742356128,4.36174236824));
#68730=CARTESIAN_POINT('Ctrl Pts',(6.98489076396,-36.4799878332,4.36174236824));
#68731=CARTESIAN_POINT('Ctrl Pts',(7.00065080016,-36.3857400536,4.3277623195));
#68732=CARTESIAN_POINT('Ctrl Pts',(7.03237160049,-36.3112466293,4.25936943399));
#68733=CARTESIAN_POINT('Ctrl Pts',(7.07250420315,-36.2742356128,4.17283994981));
#68734=CARTESIAN_POINT('Ctrl Pts',(7.11263680581,-36.2742356128,4.08631046562));
#68735=CARTESIAN_POINT('Ctrl Pts',(7.39717344286,-36.5742356128,4.53703336491));
#68736=CARTESIAN_POINT('Ctrl Pts',(7.39717342808,-36.4799878254,4.53703335475));
#68737=CARTESIAN_POINT('Ctrl Pts',(7.40695489431,-36.385740038,4.50036897905));
#68738=CARTESIAN_POINT('Ctrl Pts',(7.42664242728,-36.3112466109,4.42657326421));
#68739=CARTESIAN_POINT('Ctrl Pts',(7.45155075762,-36.2742356005,4.33320822323));
#68740=CARTESIAN_POINT('Ctrl Pts',(7.47645909178,-36.2742356128,4.23984319062));
#68741=CARTESIAN_POINT('Ctrl Pts',(7.85671042359,-36.5742356128,4.61558616292));
#68742=CARTESIAN_POINT('Ctrl Pts',(7.85671043413,-36.4799878271,4.61558615243));
#68743=CARTESIAN_POINT('Ctrl Pts',(7.85903775873,-36.3857400413,4.57747578228));
#68744=CARTESIAN_POINT('Ctrl Pts',(7.86372203974,-36.3112466149,4.50076965772));
#68745=CARTESIAN_POINT('Ctrl Pts',(7.86964850582,-36.2742356032,4.40372241788));
#68746=CARTESIAN_POINT('Ctrl Pts',(7.87557497252,-36.2742356128,4.30667518455));
#68747=CARTESIAN_POINT('Ctrl Pts',(8.54369953399,-36.5742356128,4.54933608482));
#68748=CARTESIAN_POINT('Ctrl Pts',(8.54369952872,-36.4799878363,4.54933609007));
#68749=CARTESIAN_POINT('Ctrl Pts',(8.53475132294,-36.3857400598,4.51242231126));
#68750=CARTESIAN_POINT('Ctrl Pts',(8.51674094895,-36.3112466366,4.43812459524));
#68751=CARTESIAN_POINT('Ctrl Pts',(8.49395453991,-36.2742356177,4.34412441801));
#68752=CARTESIAN_POINT('Ctrl Pts',(8.47116813057,-36.2742356128,4.25012423752));
#68753=CARTESIAN_POINT('Ctrl Pts',(9.14546603834,-36.5742356128,4.26313835988));
#68754=CARTESIAN_POINT('Ctrl Pts',(9.14546604097,-36.4799878317,4.26313835725));
#68755=CARTESIAN_POINT('Ctrl Pts',(9.12717740792,-36.3857400506,4.2306861245));
#68756=CARTESIAN_POINT('Ctrl Pts',(9.09036720445,-36.3112466257,4.16536833407));
#68757=CARTESIAN_POINT('Ctrl Pts',(9.04379557728,-36.2742356104,4.08272940811));
#68758=CARTESIAN_POINT('Ctrl Pts',(8.99722395025,-36.2742356128,4.00009048378));
#68759=CARTESIAN_POINT('Ctrl Pts',(9.33430629029,-36.5742356128,4.1449615154));
#68760=CARTESIAN_POINT('Ctrl Pts',(9.33430624684,-36.4799878386,4.14496156749));
#68761=CARTESIAN_POINT('Ctrl Pts',(9.31320927896,-36.3857400644,4.11430294877));
#68762=CARTESIAN_POINT('Ctrl Pts',(9.27074665566,-36.311246642,4.05259522538));
#68763=CARTESIAN_POINT('Ctrl Pts',(9.21702372832,-36.2742356213,3.97452363113));
#68764=CARTESIAN_POINT('Ctrl Pts',(9.16330081692,-36.2742356128,3.89645201289));
#68765=CARTESIAN_POINT('Ctrl Pts',(9.68898808689,-36.5742356128,3.86407647413));
#68766=CARTESIAN_POINT('Ctrl Pts',(9.68898813284,-36.4799878275,3.86407641904));
#68767=CARTESIAN_POINT('Ctrl Pts',(9.66297620974,-36.3857400423,3.83738683986));
#68768=CARTESIAN_POINT('Ctrl Pts',(9.61062104631,-36.3112466159,3.7836677505));
#68769=CARTESIAN_POINT('Ctrl Pts',(9.54438216355,-36.2742356039,3.7157033607));
#68770=CARTESIAN_POINT('Ctrl Pts',(9.47814326392,-36.2742356128,3.64773899629));
#68771=CARTESIAN_POINT('Ctrl Pts',(9.97409371558,-36.5742356128,3.5368417215));
#68772=CARTESIAN_POINT('Ctrl Pts',(9.97409366698,-36.4799878392,3.53684177977));
#68773=CARTESIAN_POINT('Ctrl Pts',(9.94505212424,-36.3857400657,3.51373460238));
#68774=CARTESIAN_POINT('Ctrl Pts',(9.88659916874,-36.3112466435,3.46722594263));
#68775=CARTESIAN_POINT('Ctrl Pts',(9.81264555648,-36.2742356223,3.40838393028));
#68776=CARTESIAN_POINT('Ctrl Pts',(9.73869196204,-36.2742356128,3.34954189108));
#68777=CARTESIAN_POINT('Ctrl Pts',(10.1029300816,-36.5742356128,3.36222205123));
#68778=CARTESIAN_POINT('Ctrl Pts',(10.1029301671,-36.4799878807,3.36222190496));
#68779=CARTESIAN_POINT('Ctrl Pts',(10.0727204671,-36.3857401486,3.34076368711));
#68780=CARTESIAN_POINT('Ctrl Pts',(10.0119163664,-36.3112467413,3.29757384942));
#68781=CARTESIAN_POINT('Ctrl Pts',(9.93498794039,-36.2742356875,3.24293101687));
#68782=CARTESIAN_POINT('Ctrl Pts',(9.85805945703,-36.2742356128,3.18828822444));
#68783=CARTESIAN_POINT('Ctrl Pts',(10.2192706083,-36.5742356128,3.18776254463));
#68784=CARTESIAN_POINT('Ctrl Pts',(10.2192705627,-36.4799878336,3.18776261966));
#68785=CARTESIAN_POINT('Ctrl Pts',(10.1883194918,-36.3857400544,3.16743138786));
#68786=CARTESIAN_POINT('Ctrl Pts',(10.1260230843,-36.3112466302,3.12651006944));
#68787=CARTESIAN_POINT('Ctrl Pts',(10.0472068327,-36.2742356134,3.07473700749));
#68788=CARTESIAN_POINT('Ctrl Pts',(9.96839059861,-36.2742356128,3.02296391637));
#68789=CARTESIAN_POINT('Ctrl Pts',(10.3257938388,-36.5742356128,3.01323063831));
#68790=CARTESIAN_POINT('Ctrl Pts',(10.3257938435,-36.4799878332,3.01323063056));
#68791=CARTESIAN_POINT('Ctrl Pts',(10.2942021431,-36.3857400536,2.99394903723));
#68792=CARTESIAN_POINT('Ctrl Pts',(10.2306163683,-36.3112466293,2.9551402798));
#68793=CARTESIAN_POINT('Ctrl Pts',(10.1501687536,-36.2742356128,2.90604012229));
#68794=CARTESIAN_POINT('Ctrl Pts',(10.0697211371,-36.2742356128,2.85693996784));
#68795=CARTESIAN_POINT('',(6.6247863622675,-36.5742356128,4.121293632315));
#68796=CARTESIAN_POINT('Origin',(6.79020000386945,-36.572114293675,3.87356387873257));
#68797=CARTESIAN_POINT('',(10.3257952821,-36.5742356128,3.01322822759));
#68798=CARTESIAN_POINT('Ctrl Pts',(6.62478636278,-36.5742356128,4.12129363314));
#68799=CARTESIAN_POINT('Ctrl Pts',(6.98489076396,-36.5742356127964,4.36174236824));
#68800=CARTESIAN_POINT('Ctrl Pts',(7.39717344286,-36.5742356127964,4.53703336491));
#68801=CARTESIAN_POINT('Ctrl Pts',(7.85671042359,-36.5742356127964,4.61558616292));
#68802=CARTESIAN_POINT('Ctrl Pts',(8.54369953399,-36.5742356127964,4.54933608482));
#68803=CARTESIAN_POINT('Ctrl Pts',(9.14546603834001,-36.5742356127964,4.26313835988));
#68804=CARTESIAN_POINT('Ctrl Pts',(9.33430629029,-36.5742356127964,4.1449615154));
#68805=CARTESIAN_POINT('Ctrl Pts',(9.68898808689,-36.5742356127964,3.86407647413));
#68806=CARTESIAN_POINT('Ctrl Pts',(9.97409371558,-36.5742356127964,3.5368417215));
#68807=CARTESIAN_POINT('Ctrl Pts',(10.1029300816,-36.5742356127964,3.36222205123));
#68808=CARTESIAN_POINT('Ctrl Pts',(10.2192706083,-36.5742356127964,3.18776254463));
#68809=CARTESIAN_POINT('Ctrl Pts',(10.3257952821,-36.5742356128,3.01322822759));
#68810=CARTESIAN_POINT('Origin',(10.0715309146271,-36.5721142827529,2.85804663423425));
#68811=CARTESIAN_POINT('Ctrl Pts',(10.0697226343,-38.2742356128,2.85693747561));
#68812=CARTESIAN_POINT('Ctrl Pts',(10.1501702339,-38.2742356128,2.9060376555));
#68813=CARTESIAN_POINT('Ctrl Pts',(10.2306178336,-38.2372245963,2.95513783538));
#68814=CARTESIAN_POINT('Ctrl Pts',(10.2942035987,-38.1627311721,2.99394660677));
#68815=CARTESIAN_POINT('Ctrl Pts',(10.3257952972,-38.0684833924,3.01322820232));
#68816=CARTESIAN_POINT('Ctrl Pts',(10.3257952972,-37.9742356128,3.01322820232));
#68817=CARTESIAN_POINT('Ctrl Pts',(9.96239262302,-38.2742356128,3.03279125873));
#68818=CARTESIAN_POINT('Ctrl Pts',(10.0411275292,-38.2742356128,3.08469759446));
#68819=CARTESIAN_POINT('Ctrl Pts',(10.1198624354,-38.2372245963,3.13660393018));
#68820=CARTESIAN_POINT('Ctrl Pts',(10.1820945837,-38.1627311721,3.17763052871));
#68821=CARTESIAN_POINT('Ctrl Pts',(10.2130136133,-38.0684833924,3.19801425689));
#68822=CARTESIAN_POINT('Ctrl Pts',(10.2130136133,-37.9742356128,3.19801425689));
#68823=CARTESIAN_POINT('Ctrl Pts',(9.84476270741,-38.2742356128,3.20806595154));
#68824=CARTESIAN_POINT('Ctrl Pts',(9.92144376871,-38.2742356128,3.26308291366));
#68825=CARTESIAN_POINT('Ctrl Pts',(9.99812483001,-38.2372245963,3.31809987579));
#68826=CARTESIAN_POINT('Ctrl Pts',(10.0587333807,-38.1627311721,3.36158550664));
#68827=CARTESIAN_POINT('Ctrl Pts',(10.0888461064,-38.0684833924,3.38319038106));
#68828=CARTESIAN_POINT('Ctrl Pts',(10.0888461064,-37.9742356128,3.38319038106));
#68829=CARTESIAN_POINT('Ctrl Pts',(9.71703247101,-38.2742356128,3.37827910506));
#68830=CARTESIAN_POINT('Ctrl Pts',(9.79053204643,-38.2742356128,3.43778793927));
#68831=CARTESIAN_POINT('Ctrl Pts',(9.86403162186,-38.2372245963,3.49729677347));
#68832=CARTESIAN_POINT('Ctrl Pts',(9.92212570714,-38.1627311721,3.54433248183));
#68833=CARTESIAN_POINT('Ctrl Pts',(9.9509888859,-38.0684833924,3.56770160749));
#68834=CARTESIAN_POINT('Ctrl Pts',(9.9509888859,-37.9742356128,3.56770160749));
#68835=CARTESIAN_POINT('Ctrl Pts',(9.4465153344,-38.2742356128,3.67954908967));
#68836=CARTESIAN_POINT('Ctrl Pts',(9.51165483329,-38.2742356128,3.74868285322));
#68837=CARTESIAN_POINT('Ctrl Pts',(9.57679433219,-38.2372245963,3.81781661678));
#68838=CARTESIAN_POINT('Ctrl Pts',(9.62828054625,-38.1627311721,3.87245998019));
#68839=CARTESIAN_POINT('Ctrl Pts',(9.65386079919,-38.0684833924,3.89960869375));
#68840=CARTESIAN_POINT('Ctrl Pts',(9.65386079919,-37.9742356128,3.89960869375));
#68841=CARTESIAN_POINT('Ctrl Pts',(9.11961907684,-38.2742356128,3.92493521278));
#68842=CARTESIAN_POINT('Ctrl Pts',(9.17143121953,-38.2742356128,4.00428974878));
#68843=CARTESIAN_POINT('Ctrl Pts',(9.22324336223,-38.2372245963,4.08364428479));
#68844=CARTESIAN_POINT('Ctrl Pts',(9.26419569527,-38.1627311721,4.14636604856));
#68845=CARTESIAN_POINT('Ctrl Pts',(9.28454224928,-38.0684833924,4.17752854602));
#68846=CARTESIAN_POINT('Ctrl Pts',(9.28454224928,-37.9742356128,4.17752854602));
#68847=CARTESIAN_POINT('Ctrl Pts',(8.95439425436,-38.2742356128,4.02292606705));
#68848=CARTESIAN_POINT('Ctrl Pts',(8.99905838483,-38.2742356128,4.10659587218));
#68849=CARTESIAN_POINT('Ctrl Pts',(9.04372251529,-38.2372245963,4.19026567732));
#68850=CARTESIAN_POINT('Ctrl Pts',(9.07902498138,-38.1627311721,4.25639823777));
#68851=CARTESIAN_POINT('Ctrl Pts',(9.09656459722,-38.0684833924,4.28925532855));
#68852=CARTESIAN_POINT('Ctrl Pts',(9.09656459722,-37.9742356128,4.28925532855));
#68853=CARTESIAN_POINT('Ctrl Pts',(8.43375423048,-38.2742356128,4.25670358831));
#68854=CARTESIAN_POINT('Ctrl Pts',(8.45474053418,-38.2742356128,4.35103499499));
#68855=CARTESIAN_POINT('Ctrl Pts',(8.47572683789,-38.2372245963,4.44536640166));
#68856=CARTESIAN_POINT('Ctrl Pts',(8.49231451374,-38.1627311721,4.51992599457));
#68857=CARTESIAN_POINT('Ctrl Pts',(8.50055570992,-38.0684833924,4.55696978154));
#68858=CARTESIAN_POINT('Ctrl Pts',(8.50055570992,-37.9742356128,4.55696978154));
#68859=CARTESIAN_POINT('Ctrl Pts',(7.85070473056,-38.2742356128,4.30204442107));
#68860=CARTESIAN_POINT('Ctrl Pts',(7.84356701002,-38.2742356128,4.39888585549));
#68861=CARTESIAN_POINT('Ctrl Pts',(7.83642928948,-38.2372245963,4.49572728991));
#68862=CARTESIAN_POINT('Ctrl Pts',(7.83078742393,-38.1627311721,4.57227059967));
#68863=CARTESIAN_POINT('Ctrl Pts',(7.82798466043,-38.0684833924,4.61030028076));
#68864=CARTESIAN_POINT('Ctrl Pts',(7.82798466043,-37.9742356128,4.61030028076));
#68865=CARTESIAN_POINT('Ctrl Pts',(7.46124971174,-38.2742356128,4.23337366135));
#68866=CARTESIAN_POINT('Ctrl Pts',(7.43569930686,-38.2742356128,4.32644610908));
#68867=CARTESIAN_POINT('Ctrl Pts',(7.41014890199,-38.2372245963,4.41951855682));
#68868=CARTESIAN_POINT('Ctrl Pts',(7.38995471066,-38.1627311721,4.49308356189));
#68869=CARTESIAN_POINT('Ctrl Pts',(7.37992024706,-38.0684833924,4.5296324638));
#68870=CARTESIAN_POINT('Ctrl Pts',(7.37992024706,-37.9742356128,4.5296324638));
#68871=CARTESIAN_POINT('Ctrl Pts',(7.10590026383,-38.2742356128,4.0818123451));
#68872=CARTESIAN_POINT('Ctrl Pts',(7.06551175748,-38.2742356128,4.1681709574));
#68873=CARTESIAN_POINT('Ctrl Pts',(7.02512325114,-38.2372245963,4.25452956969));
#68874=CARTESIAN_POINT('Ctrl Pts',(6.99319962237,-38.1627311721,4.32278702275));
#68875=CARTESIAN_POINT('Ctrl Pts',(6.97733965525,-38.0684833924,4.35670034561));
#68876=CARTESIAN_POINT('Ctrl Pts',(6.97733965525,-37.9742356128,4.35670034561));
#68877=CARTESIAN_POINT('Ctrl Pts',(6.79137823178,-38.2742356128,3.87179984728));
#68878=CARTESIAN_POINT('Ctrl Pts',(6.7390418526,-38.2742356128,3.95018063176));
#68879=CARTESIAN_POINT('Ctrl Pts',(6.68670547342,-38.2372245963,4.02856141623));
#68880=CARTESIAN_POINT('Ctrl Pts',(6.64533881083,-38.1627311721,4.09051357105));
#68881=CARTESIAN_POINT('Ctrl Pts',(6.62478636278,-38.0684833924,4.12129363314));
#68882=CARTESIAN_POINT('Ctrl Pts',(6.62478636278,-37.9742356128,4.12129363314));
#68883=CARTESIAN_POINT('',(6.62478636196,-37.9742356128,4.121293631845));
#68884=CARTESIAN_POINT('Origin',(6.79019999558982,-37.9763569532443,3.87356390622112));
#68885=CARTESIAN_POINT('',(10.3257952821,-37.9742356128,3.01322822759));
#68886=CARTESIAN_POINT('Origin',(10.0715333086021,-37.9763569039709,2.85804261568983));
#68887=CARTESIAN_POINT('Ctrl Pts',(6.62478636278,-37.9742356128,4.12129363314));
#68888=CARTESIAN_POINT('Ctrl Pts',(6.77209862642,-37.9742356128,4.21965690596));
#68889=CARTESIAN_POINT('Ctrl Pts',(6.92865784201,-37.9742356128,4.30723684413));
#68890=CARTESIAN_POINT('Ctrl Pts',(7.09318322917,-37.9742356128,4.3815910145));
#68891=CARTESIAN_POINT('Ctrl Pts',(7.35028595871,-37.9742356128,4.47075138071));
#68892=CARTESIAN_POINT('Ctrl Pts',(7.61904353259,-37.9742356128,4.52294971153));
#68893=CARTESIAN_POINT('Ctrl Pts',(7.71036083894,-37.9742356128,4.53610818987));
#68894=CARTESIAN_POINT('Ctrl Pts',(7.98526439172,-37.9742356128,4.56199873534));
#68895=CARTESIAN_POINT('Ctrl Pts',(8.26232955523,-37.9742356128,4.54692356056));
#68896=CARTESIAN_POINT('Ctrl Pts',(8.44551261186,-37.9742356128,4.51817058272));
#68897=CARTESIAN_POINT('Ctrl Pts',(8.80081499429,-37.9742356128,4.42491856124));
#68898=CARTESIAN_POINT('Ctrl Pts',(9.12906626269,-37.9742356128,4.26637622783));
#68899=CARTESIAN_POINT('Ctrl Pts',(9.28446203337,-37.9742356128,4.17257256592));
#68900=CARTESIAN_POINT('Ctrl Pts',(9.50104385578,-37.9742356128,4.01328807602));
#68901=CARTESIAN_POINT('Ctrl Pts',(9.69216005671,-37.9742356128,3.83525523444));
#68902=CARTESIAN_POINT('Ctrl Pts',(9.75297759191,-37.9742356128,3.77433260224));
#68903=CARTESIAN_POINT('Ctrl Pts',(9.92328269257,-37.9742356128,3.5920488793));
#68904=CARTESIAN_POINT('Ctrl Pts',(10.0727130885,-37.9742356128,3.39989142333));
#68905=CARTESIAN_POINT('Ctrl Pts',(10.163703376,-37.9742356128,3.27006200044));
#68906=CARTESIAN_POINT('Ctrl Pts',(10.24741676,-37.9742356128,3.14164655991));
#68907=CARTESIAN_POINT('Ctrl Pts',(10.3257952821,-37.9742356128,3.01322822759));
#68908=CARTESIAN_POINT('Ctrl Pts',(10.3257952821,-37.9742356128,3.01322822759));
#68909=CARTESIAN_POINT('Ctrl Pts',(10.3257952821,-36.2942356128,3.01322822759));
#68910=CARTESIAN_POINT('Ctrl Pts',(10.24741676,-37.9742356128,3.14164655991));
#68911=CARTESIAN_POINT('Ctrl Pts',(10.24741676,-36.2942356128,3.14164655991));
#68912=CARTESIAN_POINT('Ctrl Pts',(10.163703376,-37.9742356128,3.27006200044));
#68913=CARTESIAN_POINT('Ctrl Pts',(10.163703376,-36.2942356128,3.27006200044));
#68914=CARTESIAN_POINT('Ctrl Pts',(10.0727130885,-37.9742356128,3.39989142333));
#68915=CARTESIAN_POINT('Ctrl Pts',(10.0727130885,-36.2942356128,3.39989142333));
#68916=CARTESIAN_POINT('Ctrl Pts',(9.92328269257,-37.9742356128,3.5920488793));
#68917=CARTESIAN_POINT('Ctrl Pts',(9.92328269257,-36.2942356128,3.5920488793));
#68918=CARTESIAN_POINT('Ctrl Pts',(9.75297759191,-37.9742356128,3.77433260224));
#68919=CARTESIAN_POINT('Ctrl Pts',(9.75297759191,-36.2942356128,3.77433260224));
#68920=CARTESIAN_POINT('Ctrl Pts',(9.69216005671,-37.9742356128,3.83525523444));
#68921=CARTESIAN_POINT('Ctrl Pts',(9.69216005671,-36.2942356128,3.83525523444));
#68922=CARTESIAN_POINT('Ctrl Pts',(9.50104385578,-37.9742356128,4.01328807602));
#68923=CARTESIAN_POINT('Ctrl Pts',(9.50104385578,-36.2942356128,4.01328807602));
#68924=CARTESIAN_POINT('Ctrl Pts',(9.28446203337,-37.9742356128,4.17257256592));
#68925=CARTESIAN_POINT('Ctrl Pts',(9.28446203337,-36.2942356128,4.17257256592));
#68926=CARTESIAN_POINT('Ctrl Pts',(9.12906626269,-37.9742356128,4.26637622783));
#68927=CARTESIAN_POINT('Ctrl Pts',(9.12906626269,-36.2942356128,4.26637622783));
#68928=CARTESIAN_POINT('Ctrl Pts',(8.80081499429,-37.9742356128,4.42491856124));
#68929=CARTESIAN_POINT('Ctrl Pts',(8.80081499429,-36.2942356128,4.42491856124));
#68930=CARTESIAN_POINT('Ctrl Pts',(8.44551261186,-37.9742356128,4.51817058272));
#68931=CARTESIAN_POINT('Ctrl Pts',(8.44551261186,-36.2942356128,4.51817058272));
#68932=CARTESIAN_POINT('Ctrl Pts',(8.26232955523,-37.9742356128,4.54692356056));
#68933=CARTESIAN_POINT('Ctrl Pts',(8.26232955523,-36.2942356128,4.54692356056));
#68934=CARTESIAN_POINT('Ctrl Pts',(7.98526439172,-37.9742356128,4.56199873534));
#68935=CARTESIAN_POINT('Ctrl Pts',(7.98526439172,-36.2942356128,4.56199873534));
#68936=CARTESIAN_POINT('Ctrl Pts',(7.71036083894,-37.9742356128,4.53610818987));
#68937=CARTESIAN_POINT('Ctrl Pts',(7.71036083894,-36.2942356128,4.53610818987));
#68938=CARTESIAN_POINT('Ctrl Pts',(7.61904353259,-37.9742356128,4.52294971153));
#68939=CARTESIAN_POINT('Ctrl Pts',(7.61904353259,-36.2942356128,4.52294971153));
#68940=CARTESIAN_POINT('Ctrl Pts',(7.35028595871,-37.9742356128,4.47075138071));
#68941=CARTESIAN_POINT('Ctrl Pts',(7.35028595871,-36.2942356128,4.47075138071));
#68942=CARTESIAN_POINT('Ctrl Pts',(7.09318322917,-37.9742356128,4.3815910145));
#68943=CARTESIAN_POINT('Ctrl Pts',(7.09318322917,-36.2942356128,4.3815910145));
#68944=CARTESIAN_POINT('Ctrl Pts',(6.92865784201,-37.9742356128,4.30723684413));
#68945=CARTESIAN_POINT('Ctrl Pts',(6.92865784201,-36.2942356128,4.30723684413));
#68946=CARTESIAN_POINT('Ctrl Pts',(6.77209862642,-37.9742356128,4.21965690596));
#68947=CARTESIAN_POINT('Ctrl Pts',(6.77209862642,-36.2942356128,4.21965690596));
#68948=CARTESIAN_POINT('Ctrl Pts',(6.62478636278,-37.9742356128,4.12129363314));
#68949=CARTESIAN_POINT('Ctrl Pts',(6.62478636278,-36.2942356128,4.12129363314));
#68950=CARTESIAN_POINT('',(10.3257952821,-37.2742356128,3.01322822759));
#68951=CARTESIAN_POINT('',(6.62478636278,-37.2742356128,4.12129363314));
#68952=CARTESIAN_POINT('Ctrl Pts',(6.16208308783,-36.5742356128,4.4189333977));
#68953=CARTESIAN_POINT('Ctrl Pts',(6.16208308783,-36.4799878332,4.4189333977));
#68954=CARTESIAN_POINT('Ctrl Pts',(6.12555180739,-36.3857400536,4.42487316974));
#68955=CARTESIAN_POINT('Ctrl Pts',(6.0520239654,-36.3112466293,4.4368283658));
#68956=CARTESIAN_POINT('Ctrl Pts',(5.95899782364,-36.2742356128,4.45195387109));
#68957=CARTESIAN_POINT('Ctrl Pts',(5.86597168188,-36.2742356128,4.46707937639));
#68958=CARTESIAN_POINT('Ctrl Pts',(6.15238298742,-36.5742356128,4.35927503269));
#68959=CARTESIAN_POINT('Ctrl Pts',(6.15238298742,-36.4799878332,4.35927503269));
#68960=CARTESIAN_POINT('Ctrl Pts',(6.11466577784,-36.3857400536,4.35792099922));
#68961=CARTESIAN_POINT('Ctrl Pts',(6.03875096538,-36.3112466293,4.35519565622));
#68962=CARTESIAN_POINT('Ctrl Pts',(5.94270487345,-36.2742356128,4.35174761258));
#68963=CARTESIAN_POINT('Ctrl Pts',(5.84665878152,-36.2742356128,4.34829956896));
#68964=CARTESIAN_POINT('Ctrl Pts',(6.15762307668,-36.5742356128,4.29742569118));
#68965=CARTESIAN_POINT('Ctrl Pts',(6.15762309009,-36.4799878341,4.29742572463));
#68966=CARTESIAN_POINT('Ctrl Pts',(6.12052271305,-36.3857400553,4.28842649608));
#68967=CARTESIAN_POINT('Ctrl Pts',(6.04584940666,-36.3112466313,4.27031343988));
#68968=CARTESIAN_POINT('Ctrl Pts',(5.95137403766,-36.2742356142,4.24739707171));
#68969=CARTESIAN_POINT('Ctrl Pts',(5.85689866288,-36.2742356128,4.22448069029));
#68970=CARTESIAN_POINT('Ctrl Pts',(6.1785485954,-36.5742356128,4.23847486966));
#68971=CARTESIAN_POINT('Ctrl Pts',(6.17854857015,-36.4799878332,4.23847488615));
#68972=CARTESIAN_POINT('Ctrl Pts',(6.14407261188,-36.3857400535,4.22209265639));
#68973=CARTESIAN_POINT('Ctrl Pts',(6.07468029561,-36.3112466293,4.1891186584));
#68974=CARTESIAN_POINT('Ctrl Pts',(5.98688692179,-36.2742356128,4.14740088542));
#68975=CARTESIAN_POINT('Ctrl Pts',(5.89909355815,-36.2742356128,4.10568310582));
#68976=CARTESIAN_POINT('Ctrl Pts',(6.25923171959,-36.5742356128,4.11978495173));
#68977=CARTESIAN_POINT('Ctrl Pts',(6.25923175272,-36.4799878333,4.11978493009));
#68978=CARTESIAN_POINT('Ctrl Pts',(6.23474842569,-36.3857400538,4.08878629998));
#68979=CARTESIAN_POINT('Ctrl Pts',(6.1854715852,-36.3112466295,4.02639543407));
#68980=CARTESIAN_POINT('Ctrl Pts',(6.12312665839,-36.2742356129,3.94745911673));
#68981=CARTESIAN_POINT('Ctrl Pts',(6.06078171822,-36.2742356128,3.86852280807));
#68982=CARTESIAN_POINT('Ctrl Pts',(6.39414337331,-36.5742356128,4.06099492613));
#68983=CARTESIAN_POINT('Ctrl Pts',(6.39414332985,-36.4799878331,4.06099495453));
#68984=CARTESIAN_POINT('Ctrl Pts',(6.38612870308,-36.3857400534,4.02281971522));
#68985=CARTESIAN_POINT('Ctrl Pts',(6.369995284,-36.3112466292,3.9459813705));
#68986=CARTESIAN_POINT('Ctrl Pts',(6.34958448959,-36.2742356127,3.84876749811));
#68987=CARTESIAN_POINT('Ctrl Pts',(6.32917371276,-36.2742356128,3.75155361429));
#68988=CARTESIAN_POINT('Ctrl Pts',(6.47897493351,-36.5742356128,4.05513069729));
#68989=CARTESIAN_POINT('Ctrl Pts',(6.47897491719,-36.4799878312,4.05513067751));
#68990=CARTESIAN_POINT('Ctrl Pts',(6.48151319419,-36.3857400495,4.01612595006));
#68991=CARTESIAN_POINT('Ctrl Pts',(6.48663098039,-36.3112466242,3.93762581777));
#68992=CARTESIAN_POINT('Ctrl Pts',(6.49310219221,-36.2742356096,3.83830627934));
#68993=CARTESIAN_POINT('Ctrl Pts',(6.49957341023,-36.2742356128,3.73898674982));
#68994=CARTESIAN_POINT('Ctrl Pts',(6.55876184042,-36.5742356128,4.07720779466));
#68995=CARTESIAN_POINT('Ctrl Pts',(6.55876183658,-36.4799878345,4.07720779208));
#68996=CARTESIAN_POINT('Ctrl Pts',(6.57126454019,-36.3857400562,4.04105280425));
#68997=CARTESIAN_POINT('Ctrl Pts',(6.59642328625,-36.3112466325,3.96827827511));
#68998=CARTESIAN_POINT('Ctrl Pts',(6.62825617609,-36.2742356148,3.87620692129));
#68999=CARTESIAN_POINT('Ctrl Pts',(6.66008906758,-36.2742356128,3.78413556779));
#69000=CARTESIAN_POINT('Ctrl Pts',(6.62478636073,-36.5742356128,4.12129362984));
#69001=CARTESIAN_POINT('Ctrl Pts',(6.62478636078,-36.4799878332,4.12129362988));
#69002=CARTESIAN_POINT('Ctrl Pts',(6.64533878987,-36.3857400535,4.09051355751));
#69003=CARTESIAN_POINT('Ctrl Pts',(6.68670541424,-36.3112466292,4.02856138193));
#69004=CARTESIAN_POINT('Ctrl Pts',(6.73904174502,-36.2742356128,3.95018057117));
#69005=CARTESIAN_POINT('Ctrl Pts',(6.79137807575,-36.2742356128,3.87179976043));
#69006=CARTESIAN_POINT('',(6.16208308816031,-36.5742356128,4.41893339764629));
#69007=CARTESIAN_POINT('Origin',(5.8680654705604,-36.5721143212264,4.46673889588175));
#69008=CARTESIAN_POINT('Ctrl Pts',(6.16208308783,-36.5742356128,4.4189333977));
#69009=CARTESIAN_POINT('Ctrl Pts',(6.13973650651,-36.5742356128,4.28149559307));
#69010=CARTESIAN_POINT('Ctrl Pts',(6.19622108576,-36.5742356128,4.13004365321));
#69011=CARTESIAN_POINT('Ctrl Pts',(6.34774592774,-36.5742356128,4.03257337207));
#69012=CARTESIAN_POINT('Ctrl Pts',(6.50898576372,-36.5742356128,4.04397131362));
#69013=CARTESIAN_POINT('Ctrl Pts',(6.62478636278,-36.5742356128,4.12129363314));
#69014=CARTESIAN_POINT('Ctrl Pts',(6.79137807329,-38.2742356128,3.87179977251));
#69015=CARTESIAN_POINT('Ctrl Pts',(6.73904174287,-38.2742356128,3.95018057885));
#69016=CARTESIAN_POINT('Ctrl Pts',(6.68670541245,-38.2372245963,4.02856138519));
#69017=CARTESIAN_POINT('Ctrl Pts',(6.6453387884,-38.1627311721,4.09051355729));
#69018=CARTESIAN_POINT('Ctrl Pts',(6.6247863595,-38.0684833924,4.12129362796));
#69019=CARTESIAN_POINT('Ctrl Pts',(6.6247863595,-37.9742356128,4.12129362796));
#69020=CARTESIAN_POINT('Ctrl Pts',(6.67468686061,-38.2742356128,3.79388274471));
#69021=CARTESIAN_POINT('Ctrl Pts',(6.64057040577,-38.2742356128,3.88442933328));
#69022=CARTESIAN_POINT('Ctrl Pts',(6.60645395093,-38.2372245963,3.97497592186));
#69023=CARTESIAN_POINT('Ctrl Pts',(6.57948981739,-38.1627311721,4.04654496794));
#69024=CARTESIAN_POINT('Ctrl Pts',(6.56609081204,-38.0684833924,4.08210148774));
#69025=CARTESIAN_POINT('Ctrl Pts',(6.56609081204,-37.9742356128,4.08210148774));
#69026=CARTESIAN_POINT('Ctrl Pts',(6.53492809075,-38.2742356128,3.7495789243));
#69027=CARTESIAN_POINT('Ctrl Pts',(6.52286609392,-38.2742356128,3.84720752091));
#69028=CARTESIAN_POINT('Ctrl Pts',(6.51080409709,-38.2372245963,3.94483611753));
#69029=CARTESIAN_POINT('Ctrl Pts',(6.50126803274,-38.1627311721,4.0220001801));
#69030=CARTESIAN_POINT('Ctrl Pts',(6.49653356236,-38.0684833924,4.06034039907));
#69031=CARTESIAN_POINT('Ctrl Pts',(6.49653356236,-37.9742356128,4.06034039907));
#69032=CARTESIAN_POINT('Ctrl Pts',(6.38553386058,-38.2742356128,3.74945814774));
#69033=CARTESIAN_POINT('Ctrl Pts',(6.39707418027,-38.2742356128,3.84703544696));
#69034=CARTESIAN_POINT('Ctrl Pts',(6.40861449997,-38.2372245963,3.94461274618));
#69035=CARTESIAN_POINT('Ctrl Pts',(6.41773671293,-38.1627311721,4.02173930641));
#69036=CARTESIAN_POINT('Ctrl Pts',(6.42226783906,-38.0684833924,4.06005633783));
#69037=CARTESIAN_POINT('Ctrl Pts',(6.42226783906,-37.9742356128,4.06005633783));
#69038=CARTESIAN_POINT('Ctrl Pts',(6.10848563002,-38.2742356128,3.83467286799));
#69039=CARTESIAN_POINT('Ctrl Pts',(6.16340332634,-38.2742356128,3.91886622309));
#69040=CARTESIAN_POINT('Ctrl Pts',(6.21832102267,-38.2372245963,4.00305957819));
#69041=CARTESIAN_POINT('Ctrl Pts',(6.26172720453,-38.1627311721,4.06960454208));
#69042=CARTESIAN_POINT('Ctrl Pts',(6.28329408668,-38.0684833924,4.10266864079));
#69043=CARTESIAN_POINT('Ctrl Pts',(6.28329408668,-37.9742356128,4.10266864079));
#69044=CARTESIAN_POINT('Ctrl Pts',(5.91969829593,-38.2742356128,4.0541842541));
#69045=CARTESIAN_POINT('Ctrl Pts',(6.00421162703,-38.2742356128,4.10402542076));
#69046=CARTESIAN_POINT('Ctrl Pts',(6.08872495813,-38.2372245963,4.15386658741));
#69047=CARTESIAN_POINT('Ctrl Pts',(6.15552503566,-38.1627311721,4.19326244205));
#69048=CARTESIAN_POINT('Ctrl Pts',(6.18871258397,-38.0684833924,4.21283361496));
#69049=CARTESIAN_POINT('Ctrl Pts',(6.18871258397,-37.9742356128,4.21283361496));
#69050=CARTESIAN_POINT('Ctrl Pts',(5.86049982571,-38.2742356128,4.18805332395));
#69051=CARTESIAN_POINT('Ctrl Pts',(5.95442429429,-38.2742356128,4.21671667916));
#69052=CARTESIAN_POINT('Ctrl Pts',(6.04834876288,-38.2372245963,4.24538003438));
#69053=CARTESIAN_POINT('Ctrl Pts',(6.12258586761,-38.1627311721,4.26803136845));
#69054=CARTESIAN_POINT('Ctrl Pts',(6.15947069476,-38.0684833924,4.27929161731));
#69055=CARTESIAN_POINT('Ctrl Pts',(6.15947069476,-37.9742356128,4.27929161731));
#69056=CARTESIAN_POINT('Ctrl Pts',(5.84384347146,-38.2742356128,4.33098461465));
#69057=CARTESIAN_POINT('Ctrl Pts',(5.94032979225,-38.2742356128,4.33714019046));
#69058=CARTESIAN_POINT('Ctrl Pts',(6.03681611303,-38.2372245963,4.34329576626));
#69059=CARTESIAN_POINT('Ctrl Pts',(6.11307940101,-38.1627311721,4.34816391257));
#69060=CARTESIAN_POINT('Ctrl Pts',(6.15096896934,-38.0684833924,4.35057842098));
#69061=CARTESIAN_POINT('Ctrl Pts',(6.15096896934,-37.9742356128,4.35057842098));
#69062=CARTESIAN_POINT('Ctrl Pts',(5.86597168188,-38.2742356128,4.46707937639));
#69063=CARTESIAN_POINT('Ctrl Pts',(5.95899782364,-38.2742356128,4.45195387109));
#69064=CARTESIAN_POINT('Ctrl Pts',(6.0520239654,-38.2372245963,4.4368283658));
#69065=CARTESIAN_POINT('Ctrl Pts',(6.12555180739,-38.1627311721,4.42487316974));
#69066=CARTESIAN_POINT('Ctrl Pts',(6.16208308783,-38.0684833924,4.4189333977));
#69067=CARTESIAN_POINT('Ctrl Pts',(6.16208308783,-37.9742356128,4.4189333977));
#69068=CARTESIAN_POINT('',(6.16208308783,-37.9742356128,4.4189333977));
#69069=CARTESIAN_POINT('Origin',(5.86806547685312,-37.9763569039045,4.46673893760219));
#69070=CARTESIAN_POINT('Ctrl Pts',(6.16208308783,-37.9742356128,4.4189333977));
#69071=CARTESIAN_POINT('Ctrl Pts',(6.15919261847849,-37.9742356128,4.40115619248035));
#69072=CARTESIAN_POINT('Ctrl Pts',(6.1578958682542,-37.9742356128,4.38312498437982));
#69073=CARTESIAN_POINT('Ctrl Pts',(6.15821910283257,-37.9742356128,4.365132913013));
#69074=CARTESIAN_POINT('Ctrl Pts',(6.15854192725494,-37.9742356128,4.34716367198903));
#69075=CARTESIAN_POINT('Ctrl Pts',(6.16048059072391,-37.9742356128,4.32923373168325));
#69076=CARTESIAN_POINT('Ctrl Pts',(6.16401008069579,-37.9742356128,4.31162615872299));
#69077=CARTESIAN_POINT('Ctrl Pts',(6.16753519147487,-37.9742356128,4.29404043224978));
#69078=CARTESIAN_POINT('Ctrl Pts',(6.17264712597345,-37.9742356128,4.2767765339022));
#69079=CARTESIAN_POINT('Ctrl Pts',(6.17927059085163,-37.9742356128,4.2601036138989));
#69080=CARTESIAN_POINT('Ctrl Pts',(6.185882474244,-37.9742356128,4.24345984739608));
#69081=CARTESIAN_POINT('Ctrl Pts',(6.19400052518591,-37.9742356128,4.22740524746908));
#69082=CARTESIAN_POINT('Ctrl Pts',(6.20350066431033,-37.9742356128,4.21219088469382));
#69083=CARTESIAN_POINT('Ctrl Pts',(6.212990313481,-37.9742356128,4.196993321458));
#69084=CARTESIAN_POINT('Ctrl Pts',(6.22385890537373,-37.9742356128,4.18263438843155));
#69085=CARTESIAN_POINT('Ctrl Pts',(6.2359349706977,-37.9742356128,4.16934392349151));
#69086=CARTESIAN_POINT('Ctrl Pts',(6.24799262158315,-37.9742356128,4.1560737247924));
#69087=CARTESIAN_POINT('Ctrl Pts',(6.2612539503332,-37.9742356128,4.14386897449315));
#69088=CARTESIAN_POINT('Ctrl Pts',(6.27550217470401,-37.9742356128,4.13293448634083));
#69089=CARTESIAN_POINT('Ctrl Pts',(6.28129678738945,-37.9742356128,4.12848753757673));
#69090=CARTESIAN_POINT('Ctrl Pts',(6.2872541085728,-37.9742356128,4.12425039027964));
#69091=CARTESIAN_POINT('Ctrl Pts',(6.29335744170626,-37.9742356128,4.12023554862129));
#69092=CARTESIAN_POINT('Ctrl Pts',(6.30811707445383,-37.9742356128,4.11052649504004));
#69093=CARTESIAN_POINT('Ctrl Pts',(6.32373132640604,-37.9742356128,4.1021214113779));
#69094=CARTESIAN_POINT('Ctrl Pts',(6.33994605204457,-37.9742356128,4.09515243205252));
#69095=CARTESIAN_POINT('Ctrl Pts',(6.35637472997303,-37.9742356128,4.08809149748113));
#69096=CARTESIAN_POINT('Ctrl Pts',(6.3734193219789,-37.9742356128,4.08250481550582));
#69097=CARTESIAN_POINT('Ctrl Pts',(6.39080390205361,-37.9742356128,4.07847709763709));
#69098=CARTESIAN_POINT('Ctrl Pts',(6.40837174310293,-37.9742356128,4.07440692125058));
#69099=CARTESIAN_POINT('Ctrl Pts',(6.42628621839665,-37.9742356128,4.07192870130141));
#69100=CARTESIAN_POINT('Ctrl Pts',(6.44425897825834,-37.9742356128,4.07107677316466));
#69101=CARTESIAN_POINT('Ctrl Pts',(6.46238597578069,-37.9742356128,4.070217533997));
#69102=CARTESIAN_POINT('Ctrl Pts',(6.48057166961878,-37.9742356128,4.07101252700654));
#69103=CARTESIAN_POINT('Ctrl Pts',(6.49852532361879,-37.9742356128,4.0734443564819));
#69104=CARTESIAN_POINT('Ctrl Pts',(6.51648139915476,-37.9742356128,4.07587651395527));
#69105=CARTESIAN_POINT('Ctrl Pts',(6.53420479100214,-37.9742356128,4.07994576358515));
#69106=CARTESIAN_POINT('Ctrl Pts',(6.55141856220953,-37.9742356128,4.08558449609217));
#69107=CARTESIAN_POINT('Ctrl Pts',(6.56853351254586,-37.9742356128,4.09119085774616));
#69108=CARTESIAN_POINT('Ctrl Pts',(6.58514414635111,-37.9742356128,4.09834849003559));
#69109=CARTESIAN_POINT('Ctrl Pts',(6.60100030737395,-37.9742356128,4.10694459823105));
#69110=CARTESIAN_POINT('Ctrl Pts',(6.60913757342369,-37.9742356128,4.11135605818519));
#69111=CARTESIAN_POINT('Ctrl Pts',(6.61707654315828,-37.9742356128,4.11614563605583));
#69112=CARTESIAN_POINT('Ctrl Pts',(6.6247863595,-37.9742356128,4.12129362796));
#69113=CARTESIAN_POINT('Ctrl Pts',(6.62478636278,-37.9742356128,4.12129363314));
#69114=CARTESIAN_POINT('Ctrl Pts',(6.62478636278,-36.2942356128,4.12129363314));
#69115=CARTESIAN_POINT('Ctrl Pts',(6.50898576372,-37.9742356128,4.04397131362));
#69116=CARTESIAN_POINT('Ctrl Pts',(6.50898576372,-36.2942356128,4.04397131362));
#69117=CARTESIAN_POINT('Ctrl Pts',(6.34774592774,-37.9742356128,4.03257337207));
#69118=CARTESIAN_POINT('Ctrl Pts',(6.34774592774,-36.2942356128,4.03257337207));
#69119=CARTESIAN_POINT('Ctrl Pts',(6.19622108576,-37.9742356128,4.13004365321));
#69120=CARTESIAN_POINT('Ctrl Pts',(6.19622108576,-36.2942356128,4.13004365321));
#69121=CARTESIAN_POINT('Ctrl Pts',(6.13973650651,-37.9742356128,4.28149559307));
#69122=CARTESIAN_POINT('Ctrl Pts',(6.13973650651,-36.2942356128,4.28149559307));
#69123=CARTESIAN_POINT('Ctrl Pts',(6.16208308783,-37.9742356128,4.4189333977));
#69124=CARTESIAN_POINT('Ctrl Pts',(6.16208308783,-36.2942356128,4.4189333977));
#69125=CARTESIAN_POINT('',(6.16208308783,-37.2742356128,4.4189333977));
#69126=CARTESIAN_POINT('Ctrl Pts',(-4.4408920985E-16,-36.5742356128,11.6643459897));
#69127=CARTESIAN_POINT('Ctrl Pts',(0.,-36.4799878332,11.6643459897));
#69128=CARTESIAN_POINT('Ctrl Pts',(-2.4666821874E-6,-36.3857400536,11.6273349733));
#69129=CARTESIAN_POINT('Ctrl Pts',(-7.43146349125E-6,-36.3112466293,11.5528415491));
#69130=CARTESIAN_POINT('Ctrl Pts',(-1.37128181037E-5,-36.2742356128,11.4585937697));
#69131=CARTESIAN_POINT('Ctrl Pts',(-1.99941727144E-5,-36.2742356128,11.3643459904));
#69132=CARTESIAN_POINT('Ctrl Pts',(1.22322324235,-36.5742356128,11.6642644652));
#69133=CARTESIAN_POINT('Ctrl Pts',(1.22322324235,-36.4799878332,11.6642644652));
#69134=CARTESIAN_POINT('Ctrl Pts',(1.21599829202,-36.3857400536,11.6272539302));
#69135=CARTESIAN_POINT('Ctrl Pts',(1.20145637047,-36.3112466293,11.5527614749));
#69136=CARTESIAN_POINT('Ctrl Pts',(1.18305818534,-36.2742356128,11.4585149213));
#69137=CARTESIAN_POINT('Ctrl Pts',(1.16466000022,-36.2742356128,11.3642683676));
#69138=CARTESIAN_POINT('Ctrl Pts',(2.4473136708,-36.5742356128,11.3659246093));
#69139=CARTESIAN_POINT('Ctrl Pts',(2.44731353996,-36.4799878304,11.3659245634));
#69140=CARTESIAN_POINT('Ctrl Pts',(2.43279023211,-36.385740048,11.3306770417));
#69141=CARTESIAN_POINT('Ctrl Pts',(2.40355880045,-36.3112466227,11.2597331237));
#69142=CARTESIAN_POINT('Ctrl Pts',(2.36657578312,-36.2742356084,11.1699761465));
#69143=CARTESIAN_POINT('Ctrl Pts',(2.32959281761,-36.2742356128,11.080219189));
#69144=CARTESIAN_POINT('Ctrl Pts',(3.57166410201,-36.5742356128,10.7642929822));
#69145=CARTESIAN_POINT('Ctrl Pts',(3.57166393324,-36.4799878332,10.7642932734));
#69146=CARTESIAN_POINT('Ctrl Pts',(3.55046878885,-36.3857400536,10.7326400178));
#69147=CARTESIAN_POINT('Ctrl Pts',(3.50780873346,-36.3112466293,10.6689298739));
#69148=CARTESIAN_POINT('Ctrl Pts',(3.45383608788,-36.2742356128,10.5883247871));
#69149=CARTESIAN_POINT('Ctrl Pts',(3.39986350918,-36.2742356128,10.5077195847));
#69150=CARTESIAN_POINT('Ctrl Pts',(5.21608381041,-36.5742356128,9.26358008756));
#69151=CARTESIAN_POINT('Ctrl Pts',(5.21608394001,-36.4799878332,9.26357986393));
#69152=CARTESIAN_POINT('Ctrl Pts',(5.1851705575,-36.3857400536,9.24078655442));
#69153=CARTESIAN_POINT('Ctrl Pts',(5.12294992148,-36.3112466293,9.1949099969));
#69154=CARTESIAN_POINT('Ctrl Pts',(5.04422937351,-36.2742356128,9.13686787374));
#69155=CARTESIAN_POINT('Ctrl Pts',(4.96550877419,-36.2742356128,9.07882583933));
#69156=CARTESIAN_POINT('Ctrl Pts',(6.08439879036,-36.5742356128,7.24167411427));
#69157=CARTESIAN_POINT('Ctrl Pts',(6.08439869084,-36.4799878332,7.24167428599));
#69158=CARTESIAN_POINT('Ctrl Pts',(6.04833274366,-36.3857400536,7.23086825093));
#69159=CARTESIAN_POINT('Ctrl Pts',(5.97574160406,-36.3112466293,7.20911826662));
#69160=CARTESIAN_POINT('Ctrl Pts',(5.88390062773,-36.2742356128,7.1816004922));
#69161=CARTESIAN_POINT('Ctrl Pts',(5.79205969084,-36.2742356128,7.15408264964));
#69162=CARTESIAN_POINT('Ctrl Pts',(6.28999565278,-36.5742356128,6.30194108143));
#69163=CARTESIAN_POINT('Ctrl Pts',(6.28999570655,-36.4799878425,6.30194140801));
#69164=CARTESIAN_POINT('Ctrl Pts',(6.25270268299,-36.3857400722,6.29672322672));
#69165=CARTESIAN_POINT('Ctrl Pts',(6.1776416364,-36.3112466512,6.28622029667));
#69166=CARTESIAN_POINT('Ctrl Pts',(6.08267565391,-36.2742356274,6.27293185144));
#69167=CARTESIAN_POINT('Ctrl Pts',(5.98770964456,-36.2742356128,6.25964327781));
#69168=CARTESIAN_POINT('Ctrl Pts',(6.31282662857,-36.5742356128,5.34605335178));
#69169=CARTESIAN_POINT('Ctrl Pts',(6.31282662838,-36.479987833,5.34605335063));
#69170=CARTESIAN_POINT('Ctrl Pts',(6.27540577927,-36.3857400531,5.34652194592));
#69171=CARTESIAN_POINT('Ctrl Pts',(6.20008743734,-36.3112466287,5.34746491082));
#69172=CARTESIAN_POINT('Ctrl Pts',(6.10479600032,-36.2742356124,5.34865801627));
#69173=CARTESIAN_POINT('Ctrl Pts',(6.00950456354,-36.2742356128,5.34985112215));
#69174=CARTESIAN_POINT('Ctrl Pts',(6.1620830891,-36.5742356128,4.41893339717));
#69175=CARTESIAN_POINT('Ctrl Pts',(6.1620830891,-36.4799878332,4.41893339717));
#69176=CARTESIAN_POINT('Ctrl Pts',(6.12555180773,-36.3857400536,4.42487316367));
#69177=CARTESIAN_POINT('Ctrl Pts',(6.05202396388,-36.3112466293,4.43682834856));
#69178=CARTESIAN_POINT('Ctrl Pts',(5.95899781977,-36.2742356128,4.45195383973));
#69179=CARTESIAN_POINT('Ctrl Pts',(5.86597167565,-36.2742356128,4.4670793309));
#69180=CARTESIAN_POINT('',(-2.26207941267376E-14,-36.5742356128,11.664345990025));
#69181=CARTESIAN_POINT('Origin',(1.98978387159151E-5,-36.5721143212387,
11.3664672830582));
#69182=CARTESIAN_POINT('Ctrl Pts',(-8.881784197E-16,-36.5742356128,11.6643459897));
#69183=CARTESIAN_POINT('Ctrl Pts',(1.22322324235,-36.5742356127992,11.6642644652));
#69184=CARTESIAN_POINT('Ctrl Pts',(2.4473136708,-36.5742356127992,11.3659246093));
#69185=CARTESIAN_POINT('Ctrl Pts',(3.57166410201,-36.5742356127992,10.7642929822));
#69186=CARTESIAN_POINT('Ctrl Pts',(5.21608381041,-36.5742356127992,9.26358008756));
#69187=CARTESIAN_POINT('Ctrl Pts',(6.08439879036,-36.5742356127992,7.24167411427));
#69188=CARTESIAN_POINT('Ctrl Pts',(6.28999565278,-36.5742356127992,6.30194108143));
#69189=CARTESIAN_POINT('Ctrl Pts',(6.31282662857,-36.5742356127992,5.34605335178));
#69190=CARTESIAN_POINT('Ctrl Pts',(6.16208308783,-36.5742356128,4.4189333977));
#69191=CARTESIAN_POINT('Ctrl Pts',(5.86597173001,-38.2742356128,4.46707975784));
#69192=CARTESIAN_POINT('Ctrl Pts',(5.95899785196,-38.2742356128,4.45195413465));
#69193=CARTESIAN_POINT('Ctrl Pts',(6.05202397392,-38.2372245963,4.43682851147));
#69194=CARTESIAN_POINT('Ctrl Pts',(6.12555180026,-38.1627311721,4.42487322222));
#69195=CARTESIAN_POINT('Ctrl Pts',(6.16208307292,-38.0684833924,4.41893340389));
#69196=CARTESIAN_POINT('Ctrl Pts',(6.16208307292,-37.9742356128,4.41893340389));
#69197=CARTESIAN_POINT('Ctrl Pts',(6.01420213304,-38.2742356128,5.37874078181));
#69198=CARTESIAN_POINT('Ctrl Pts',(6.10956494828,-38.2742356128,5.37798657976));
#69199=CARTESIAN_POINT('Ctrl Pts',(6.20492776352,-38.2372245963,5.37723237772));
#69200=CARTESIAN_POINT('Ctrl Pts',(6.28030251857,-38.1627311721,5.37663629724));
#69201=CARTESIAN_POINT('Ctrl Pts',(6.3177514017,-38.0684833924,5.37634008214));
#69202=CARTESIAN_POINT('Ctrl Pts',(6.3177514017,-37.9742356128,5.37634008214));
#69203=CARTESIAN_POINT('Ctrl Pts',(5.98610106079,-38.2742356128,6.31912512184));
#69204=CARTESIAN_POINT('Ctrl Pts',(6.08104726414,-38.2742356128,6.3333863194));
#69205=CARTESIAN_POINT('Ctrl Pts',(6.17599346749,-38.2372245963,6.34764751696));
#69206=CARTESIAN_POINT('Ctrl Pts',(6.25103891549,-38.1627311721,6.35891950337));
#69207=CARTESIAN_POINT('Ctrl Pts',(6.28832421261,-38.0684833924,6.36451992356));
#69208=CARTESIAN_POINT('Ctrl Pts',(6.28832421261,-37.9742356128,6.36451992356));
#69209=CARTESIAN_POINT('Ctrl Pts',(5.77227970857,-38.2742356128,7.24175688045));
#69210=CARTESIAN_POINT('Ctrl Pts',(5.86379821772,-38.2742356128,7.27066611408));
#69211=CARTESIAN_POINT('Ctrl Pts',(5.95531672688,-38.2372245963,7.2995753477));
#69212=CARTESIAN_POINT('Ctrl Pts',(6.02765295993,-38.1627311721,7.32242521478));
#69213=CARTESIAN_POINT('Ctrl Pts',(6.06359217089,-38.0684833924,7.3337778291));
#69214=CARTESIAN_POINT('Ctrl Pts',(6.06359217089,-37.9742356128,7.3337778291));
#69215=CARTESIAN_POINT('Ctrl Pts',(4.90899024491,-38.2742356128,9.15302960102));
#69216=CARTESIAN_POINT('Ctrl Pts',(4.98682586563,-38.2742356128,9.21224464762));
#69217=CARTESIAN_POINT('Ctrl Pts',(5.06466148636,-38.2372245963,9.27145969422));
#69218=CARTESIAN_POINT('Ctrl Pts',(5.126182715,-38.1627311721,9.31826323529));
#69219=CARTESIAN_POINT('Ctrl Pts',(5.15674872066,-38.0684833924,9.34151694846));
#69220=CARTESIAN_POINT('Ctrl Pts',(5.15674872066,-37.9742356128,9.34151694846));
#69221=CARTESIAN_POINT('Ctrl Pts',(3.31894855665,-38.2742356128,10.5503954389));
#69222=CARTESIAN_POINT('Ctrl Pts',(3.37162983501,-38.2742356128,10.631675793));
#69223=CARTESIAN_POINT('Ctrl Pts',(3.42431111337,-38.2372245963,10.7129561472));
#69224=CARTESIAN_POINT('Ctrl Pts',(3.46595041963,-38.1627311721,10.7772001444));
#69225=CARTESIAN_POINT('Ctrl Pts',(3.48663827384,-38.0684833924,10.8091188417));
#69226=CARTESIAN_POINT('Ctrl Pts',(3.48663827384,-37.9742356128,10.8091188417));
#69227=CARTESIAN_POINT('Ctrl Pts',(2.2714472695,-38.2742356128,11.0941425407));
#69228=CARTESIAN_POINT('Ctrl Pts',(2.30749032166,-38.2742356128,11.1841227887));
#69229=CARTESIAN_POINT('Ctrl Pts',(2.34353337383,-38.2372245963,11.2741030367));
#69230=CARTESIAN_POINT('Ctrl Pts',(2.3720216678,-38.1627311721,11.3452234049));
#69231=CARTESIAN_POINT('Ctrl Pts',(2.38617586782,-38.0684833924,11.3805585656));
#69232=CARTESIAN_POINT('Ctrl Pts',(2.38617586782,-37.9742356128,11.3805585656));
#69233=CARTESIAN_POINT('Ctrl Pts',(1.13551567819,-38.2742356128,11.36427031));
#69234=CARTESIAN_POINT('Ctrl Pts',(1.15345363427,-38.2742356128,11.4585168943));
#69235=CARTESIAN_POINT('Ctrl Pts',(1.17139159035,-38.2372245963,11.5527634786));
#69236=CARTESIAN_POINT('Ctrl Pts',(1.18556983122,-38.1627311721,11.6272559581));
#69237=CARTESIAN_POINT('Ctrl Pts',(1.19261396576,-38.0684833924,11.6642665053));
#69238=CARTESIAN_POINT('Ctrl Pts',(1.19261396576,-37.9742356128,11.6642665053));
#69239=CARTESIAN_POINT('Ctrl Pts',(-1.99941727153E-5,-38.2742356128,11.3643459904));
#69240=CARTESIAN_POINT('Ctrl Pts',(-1.37128181037E-5,-38.2742356128,11.4585937697));
#69241=CARTESIAN_POINT('Ctrl Pts',(-7.43146349169E-6,-38.2372245963,11.5528415491));
#69242=CARTESIAN_POINT('Ctrl Pts',(-2.46668218784E-6,-38.1627311721,11.6273349733));
#69243=CARTESIAN_POINT('Ctrl Pts',(0.,-38.0684833924,11.6643459897));
#69244=CARTESIAN_POINT('Ctrl Pts',(4.4408920985E-16,-37.9742356128,11.6643459897));
#69245=CARTESIAN_POINT('',(-9.29855414889283E-10,-37.9742356128,11.664345985775));
#69246=CARTESIAN_POINT('Origin',(1.94712553347615E-5,-37.9763569038603,
11.3664672676817));
#69247=CARTESIAN_POINT('Ctrl Pts',(-8.881784197E-16,-37.9742356128,11.6643459897));
#69248=CARTESIAN_POINT('Ctrl Pts',(2.16261462464,-37.9742356128,11.6642018574));
#69249=CARTESIAN_POINT('Ctrl Pts',(4.32870534526,-37.9742356128,10.7314087249));
#69250=CARTESIAN_POINT('Ctrl Pts',(5.93623245773,-37.9742356128,8.8412691379));
#69251=CARTESIAN_POINT('Ctrl Pts',(6.5091537474,-37.9742356128,6.55351625923));
#69252=CARTESIAN_POINT('Ctrl Pts',(6.16208308783,-37.9742356128,4.4189333977));
#69253=CARTESIAN_POINT('Ctrl Pts',(6.16208308783,-37.9742356128,4.4189333977));
#69254=CARTESIAN_POINT('Ctrl Pts',(6.16208308783,-36.2942356128,4.4189333977));
#69255=CARTESIAN_POINT('Ctrl Pts',(6.5091537474,-37.9742356128,6.55351625923));
#69256=CARTESIAN_POINT('Ctrl Pts',(6.5091537474,-36.2942356128,6.55351625923));
#69257=CARTESIAN_POINT('Ctrl Pts',(5.93623245773,-37.9742356128,8.8412691379));
#69258=CARTESIAN_POINT('Ctrl Pts',(5.93623245773,-36.2942356128,8.8412691379));
#69259=CARTESIAN_POINT('Ctrl Pts',(4.32870534526,-37.9742356128,10.7314087249));
#69260=CARTESIAN_POINT('Ctrl Pts',(4.32870534526,-36.2942356128,10.7314087249));
#69261=CARTESIAN_POINT('Ctrl Pts',(2.16261462464,-37.9742356128,11.6642018574));
#69262=CARTESIAN_POINT('Ctrl Pts',(2.16261462464,-36.2942356128,11.6642018574));
#69263=CARTESIAN_POINT('Ctrl Pts',(-3.33066907388E-16,-37.9742356128,11.6643459897));
#69264=CARTESIAN_POINT('Ctrl Pts',(-3.33066907388E-16,-36.2942356128,11.6643459897));
#69265=CARTESIAN_POINT('',(-8.881784197E-16,-37.2742356128,11.6643459897));
#69266=CARTESIAN_POINT('Ctrl Pts',(-6.16208308783,-36.5742356128,4.4189333977));
#69267=CARTESIAN_POINT('Ctrl Pts',(-6.16208308783,-36.4799878332,4.4189333977));
#69268=CARTESIAN_POINT('Ctrl Pts',(-6.12555180739,-36.3857400536,4.42487316974));
#69269=CARTESIAN_POINT('Ctrl Pts',(-6.0520239654,-36.3112466293,4.4368283658));
#69270=CARTESIAN_POINT('Ctrl Pts',(-5.95899782364,-36.2742356128,4.45195387109));
#69271=CARTESIAN_POINT('Ctrl Pts',(-5.86597168188,-36.2742356128,4.46707937639));
#69272=CARTESIAN_POINT('Ctrl Pts',(-6.35839402215,-36.5742356128,5.62630124733));
#69273=CARTESIAN_POINT('Ctrl Pts',(-6.35839402215,-36.4799878332,5.62630124733));
#69274=CARTESIAN_POINT('Ctrl Pts',(-6.32070362989,-36.3857400536,5.6251121534));
#69275=CARTESIAN_POINT('Ctrl Pts',(-6.24484280119,-36.3112466293,5.6227188204));
#69276=CARTESIAN_POINT('Ctrl Pts',(-6.1488650054,-36.2742356128,5.61969081738));
#69277=CARTESIAN_POINT('Ctrl Pts',(-6.05288720961,-36.2742356128,5.61666281436));
#69278=CARTESIAN_POINT('Ctrl Pts',(-6.26045506318,-36.5742356128,6.88241111792));
#69279=CARTESIAN_POINT('Ctrl Pts',(-6.26045499686,-36.4799878304,6.88241099615));
#69280=CARTESIAN_POINT('Ctrl Pts',(-6.22333297826,-36.385740048,6.87373516796));
#69281=CARTESIAN_POINT('Ctrl Pts',(-6.14861621702,-36.3112466227,6.85627316104));
#69282=CARTESIAN_POINT('Ctrl Pts',(-6.0540859168,-36.2742356084,6.83418060869));
#69283=CARTESIAN_POINT('Ctrl Pts',(-5.95955564435,-36.2742356128,6.81208810432));
#69284=CARTESIAN_POINT('Ctrl Pts',(-5.84714534581,-36.5742356128,8.08876910145));
#69285=CARTESIAN_POINT('Ctrl Pts',(-5.84714560615,-36.4799878332,8.08876888811));
#69286=CARTESIAN_POINT('Ctrl Pts',(-5.8125000472,-36.3857400536,8.07293070699));
#69287=CARTESIAN_POINT('Ctrl Pts',(-5.74276722117,-36.3112466293,8.04105288192));
#69288=CARTESIAN_POINT('Ctrl Pts',(-5.65454236156,-36.2742356128,8.00072174454));
#69289=CARTESIAN_POINT('Ctrl Pts',(-5.56631739861,-36.2742356128,7.96039069172));
#69290=CARTESIAN_POINT('Ctrl Pts',(-4.62991621251,-36.5742356128,9.95279930682));
#69291=CARTESIAN_POINT('Ctrl Pts',(-4.6299160126,-36.4799878332,9.95279947064));
#69292=CARTESIAN_POINT('Ctrl Pts',(-4.60245517626,-36.3857400536,9.92594663756));
#69293=CARTESIAN_POINT('Ctrl Pts',(-4.54718408945,-36.3112466293,9.87189876027));
#69294=CARTESIAN_POINT('Ctrl Pts',(-4.47725615686,-36.2742356128,9.80351822959));
#69295=CARTESIAN_POINT('Ctrl Pts',(-4.40732830362,-36.2742356128,9.73513763396));
#69296=CARTESIAN_POINT('Ctrl Pts',(-2.77364981049,-36.5742356128,11.1344717293));
#69297=CARTESIAN_POINT('Ctrl Pts',(-2.77364996401,-36.4799878332,11.1344716035));
#69298=CARTESIAN_POINT('Ctrl Pts',(-2.75719363855,-36.3857400536,11.1006084628));
#69299=CARTESIAN_POINT('Ctrl Pts',(-2.72407112966,-36.3112466293,11.0324510365));
#69300=CARTESIAN_POINT('Ctrl Pts',(-2.68216504727,-36.2742356128,10.9462195277));
#69301=CARTESIAN_POINT('Ctrl Pts',(-2.64025890396,-36.2742356128,10.8599880688));
#69302=CARTESIAN_POINT('Ctrl Pts',(-1.87911669731,-36.5742356128,11.4882778234));
#69303=CARTESIAN_POINT('Ctrl Pts',(-1.87911702828,-36.4799878425,11.4882778241));
#69304=CARTESIAN_POINT('Ctrl Pts',(-1.86797905714,-36.3857400722,11.4523063823));
#69305=CARTESIAN_POINT('Ctrl Pts',(-1.84556114865,-36.3112466512,11.379905349));
#69306=CARTESIAN_POINT('Ctrl Pts',(-1.81719807576,-36.2742356274,11.2883048211));
#69307=CARTESIAN_POINT('Ctrl Pts',(-1.78883487183,-36.2742356128,11.1967042873));
#69308=CARTESIAN_POINT('Ctrl Pts',(-0.939294959167,-36.5742356128,11.664282669));
#69309=CARTESIAN_POINT('Ctrl Pts',(-0.939294958001,-36.479987833,11.664282669));
#69310=CARTESIAN_POINT('Ctrl Pts',(-0.933749468027,-36.3857400531,11.6272720345));
#69311=CARTESIAN_POINT('Ctrl Pts',(-0.922587661188,-36.3112466287,11.5527793779));
#69312=CARTESIAN_POINT('Ctrl Pts',(-0.908466021992,-36.2742356124,11.4585325701));
#69313=CARTESIAN_POINT('Ctrl Pts',(-0.894344383251,-36.2742356128,11.3642857625));
#69314=CARTESIAN_POINT('Ctrl Pts',(3.1926341727E-10,-36.5742356128,11.664345991));
#69315=CARTESIAN_POINT('Ctrl Pts',(3.15680505525E-10,-36.4799878332,11.664345991));
#69316=CARTESIAN_POINT('Ctrl Pts',(2.47261842083E-6,-36.3857400536,11.6273349746));
#69317=CARTESIAN_POINT('Ctrl Pts',(7.44871679598E-6,-36.3112466293,11.5528415504));
#69318=CARTESIAN_POINT('Ctrl Pts',(1.37443917449E-5,-36.2742356128,11.458593771));
#69319=CARTESIAN_POINT('Ctrl Pts',(2.00400681003E-5,-36.2742356128,11.3643459915));
#69320=CARTESIAN_POINT('',(-6.162083087295,-36.5742356128,4.41893339689));
#69321=CARTESIAN_POINT('Origin',(-5.86806546560554,-36.5721142937107,4.4667386455464));
#69322=CARTESIAN_POINT('Ctrl Pts',(-6.16208308783,-36.5742356128,4.4189333977));
#69323=CARTESIAN_POINT('Ctrl Pts',(-6.35839402215,-36.5742356127992,5.62630124733));
#69324=CARTESIAN_POINT('Ctrl Pts',(-6.26045506318,-36.5742356127992,6.88241111792));
#69325=CARTESIAN_POINT('Ctrl Pts',(-5.84714534581,-36.5742356127992,8.08876910145));
#69326=CARTESIAN_POINT('Ctrl Pts',(-4.62991621251,-36.5742356127992,9.95279930682));
#69327=CARTESIAN_POINT('Ctrl Pts',(-2.77364981049,-36.5742356127992,11.1344717293));
#69328=CARTESIAN_POINT('Ctrl Pts',(-1.87911669731,-36.5742356127992,11.4882778234));
#69329=CARTESIAN_POINT('Ctrl Pts',(-0.939294959167,-36.5742356127992,11.664282669));
#69330=CARTESIAN_POINT('Ctrl Pts',(-8.881784197E-16,-36.5742356128,11.6643459897));
#69331=CARTESIAN_POINT('Ctrl Pts',(1.96099429597E-5,-38.2742356128,11.3643459766));
#69332=CARTESIAN_POINT('Ctrl Pts',(1.34481291951E-5,-38.2742356128,11.4585937554));
#69333=CARTESIAN_POINT('Ctrl Pts',(7.2863154319E-6,-38.2372245963,11.5528415342));
#69334=CARTESIAN_POINT('Ctrl Pts',(2.41601918738E-6,-38.1627311721,11.6273349578));
#69335=CARTESIAN_POINT('Ctrl Pts',(-3.71941810684E-9,-38.0684833924,11.664345974));
#69336=CARTESIAN_POINT('Ctrl Pts',(-3.71941899502E-9,-37.9742356128,11.664345974));
#69337=CARTESIAN_POINT('Ctrl Pts',(-0.923613472615,-38.2742356128,11.3642840884));
#69338=CARTESIAN_POINT('Ctrl Pts',(-0.938179781412,-38.2742356128,11.4585308814));
#69339=CARTESIAN_POINT('Ctrl Pts',(-0.952746090209,-38.2372245963,11.5527776745));
#69340=CARTESIAN_POINT('Ctrl Pts',(-0.964259338702,-38.1627311721,11.6272703192));
#69341=CARTESIAN_POINT('Ctrl Pts',(-0.969979473568,-38.0684833924,11.6642809481));
#69342=CARTESIAN_POINT('Ctrl Pts',(-0.969979473568,-37.9742356128,11.6642809481));
#69343=CARTESIAN_POINT('Ctrl Pts',(-1.8472868151,-38.2742356128,11.1855666197));
#69344=CARTESIAN_POINT('Ctrl Pts',(-1.87660684553,-38.2742356128,11.2769914473));
#69345=CARTESIAN_POINT('Ctrl Pts',(-1.90592687595,-38.2372245963,11.3684162749));
#69346=CARTESIAN_POINT('Ctrl Pts',(-1.9291013597,-38.1627311721,11.4406784382));
#69347=CARTESIAN_POINT('Ctrl Pts',(-1.94061537058,-38.0684833924,11.4765808844));
#69348=CARTESIAN_POINT('Ctrl Pts',(-1.94061537058,-37.9742356128,11.4765808844));
#69349=CARTESIAN_POINT('Ctrl Pts',(-2.72362004199,-38.2742356128,10.8263883796));
#69350=CARTESIAN_POINT('Ctrl Pts',(-2.76684775976,-38.2742356128,10.9120782024));
#69351=CARTESIAN_POINT('Ctrl Pts',(-2.81007547753,-38.2372245963,10.9977680251));
#69352=CARTESIAN_POINT('Ctrl Pts',(-2.84424267491,-38.1627311721,11.065497263));
#69353=CARTESIAN_POINT('Ctrl Pts',(-2.86121814123,-38.0684833924,11.0991475569));
#69354=CARTESIAN_POINT('Ctrl Pts',(-2.86121814123,-37.9742356128,11.0991475569));
#69355=CARTESIAN_POINT('Ctrl Pts',(-4.47149525948,-38.2742356128,9.66743871091));
#69356=CARTESIAN_POINT('Ctrl Pts',(-4.54243882238,-38.2742356128,9.73475747859));
#69357=CARTESIAN_POINT('Ctrl Pts',(-4.61338238528,-38.2372245963,9.80207624627));
#69358=CARTESIAN_POINT('Ctrl Pts',(-4.66945613866,-38.1627311721,9.85528495994));
#69359=CARTESIAN_POINT('Ctrl Pts',(-4.69731563381,-38.0684833924,9.88172100368));
#69360=CARTESIAN_POINT('Ctrl Pts',(-4.69731563381,-37.9742356128,9.88172100368));
#69361=CARTESIAN_POINT('Ctrl Pts',(-5.5954485446,-38.2742356128,7.87367371291));
#69362=CARTESIAN_POINT('Ctrl Pts',(-5.68413257942,-38.2742356128,7.91262181979));
#69363=CARTESIAN_POINT('Ctrl Pts',(-5.77281661423,-38.2372245963,7.95156992668));
#69364=CARTESIAN_POINT('Ctrl Pts',(-5.84291248439,-38.1627311721,7.98235453304));
#69365=CARTESIAN_POINT('Ctrl Pts',(-5.87773859488,-38.0684833924,7.9976493876));
#69366=CARTESIAN_POINT('Ctrl Pts',(-5.87773859488,-37.9742356128,7.9976493876));
#69367=CARTESIAN_POINT('Ctrl Pts',(-5.96396296691,-38.2742356128,6.75246143244));
#69368=CARTESIAN_POINT('Ctrl Pts',(-6.05856272782,-38.2742356128,6.77359036684));
#69369=CARTESIAN_POINT('Ctrl Pts',(-6.15316248873,-38.2372245963,6.79471930124));
#69370=CARTESIAN_POINT('Ctrl Pts',(-6.22793409869,-38.1627311721,6.81141948144));
#69371=CARTESIAN_POINT('Ctrl Pts',(-6.2650833582,-38.0684833924,6.81971691948));
#69372=CARTESIAN_POINT('Ctrl Pts',(-6.2650833582,-37.9742356128,6.81971691948));
#69373=CARTESIAN_POINT('Ctrl Pts',(-6.04820993657,-38.2742356128,5.58789626039));
#69374=CARTESIAN_POINT('Ctrl Pts',(-6.14411387177,-38.2742356128,5.59046999984));
#69375=CARTESIAN_POINT('Ctrl Pts',(-6.24001780696,-38.2372245963,5.59304373929));
#69376=CARTESIAN_POINT('Ctrl Pts',(-6.31582026979,-38.1627311721,5.59507810563));
#69377=CARTESIAN_POINT('Ctrl Pts',(-6.35348164354,-38.0684833924,5.59608872751));
#69378=CARTESIAN_POINT('Ctrl Pts',(-6.35348164354,-37.9742356128,5.59608872751));
#69379=CARTESIAN_POINT('Ctrl Pts',(-5.86597168188,-38.2742356128,4.46707937639));
#69380=CARTESIAN_POINT('Ctrl Pts',(-5.95899782364,-38.2742356128,4.45195387109));
#69381=CARTESIAN_POINT('Ctrl Pts',(-6.0520239654,-38.2372245963,4.4368283658));
#69382=CARTESIAN_POINT('Ctrl Pts',(-6.12555180739,-38.1627311721,4.42487316974));
#69383=CARTESIAN_POINT('Ctrl Pts',(-6.16208308783,-38.0684833924,4.4189333977));
#69384=CARTESIAN_POINT('Ctrl Pts',(-6.16208308783,-37.9742356128,4.4189333977));
#69385=CARTESIAN_POINT('',(-6.1620830869925,-37.9742356128,4.418933396415));
#69386=CARTESIAN_POINT('Origin',(-5.86806549401996,-37.9763569532034,4.46673864924859));
#69387=CARTESIAN_POINT('Ctrl Pts',(-6.16208308783,-37.9742356128,4.4189333977));
#69388=CARTESIAN_POINT('Ctrl Pts',(-6.5091537474,-37.9742356128,6.55351625923));
#69389=CARTESIAN_POINT('Ctrl Pts',(-5.93623245773,-37.9742356128,8.8412691379));
#69390=CARTESIAN_POINT('Ctrl Pts',(-4.32870534526,-37.9742356128,10.7314087249));
#69391=CARTESIAN_POINT('Ctrl Pts',(-2.16261462464,-37.9742356128,11.6642018574));
#69392=CARTESIAN_POINT('Ctrl Pts',(-8.881784197E-16,-37.9742356128,11.6643459897));
#69393=CARTESIAN_POINT('Ctrl Pts',(-8.881784197E-16,-37.9742356128,11.6643459897));
#69394=CARTESIAN_POINT('Ctrl Pts',(-8.881784197E-16,-36.2942356128,11.6643459897));
#69395=CARTESIAN_POINT('Ctrl Pts',(-2.16261462464,-37.9742356128,11.6642018574));
#69396=CARTESIAN_POINT('Ctrl Pts',(-2.16261462464,-36.2942356128,11.6642018574));
#69397=CARTESIAN_POINT('Ctrl Pts',(-4.32870534526,-37.9742356128,10.7314087249));
#69398=CARTESIAN_POINT('Ctrl Pts',(-4.32870534526,-36.2942356128,10.7314087249));
#69399=CARTESIAN_POINT('Ctrl Pts',(-5.93623245773,-37.9742356128,8.8412691379));
#69400=CARTESIAN_POINT('Ctrl Pts',(-5.93623245773,-36.2942356128,8.8412691379));
#69401=CARTESIAN_POINT('Ctrl Pts',(-6.5091537474,-37.9742356128,6.55351625923));
#69402=CARTESIAN_POINT('Ctrl Pts',(-6.5091537474,-36.2942356128,6.55351625923));
#69403=CARTESIAN_POINT('Ctrl Pts',(-6.16208308783,-37.9742356128,4.4189333977));
#69404=CARTESIAN_POINT('Ctrl Pts',(-6.16208308783,-36.2942356128,4.4189333977));
#69405=CARTESIAN_POINT('',(-6.16208308783,-37.2742356128,4.4189333977));
#69406=CARTESIAN_POINT('Ctrl Pts',(-6.62478636278,-36.5742356128,4.12129363314));
#69407=CARTESIAN_POINT('Ctrl Pts',(-6.62478636278,-36.4799878332,4.12129363314));
#69408=CARTESIAN_POINT('Ctrl Pts',(-6.64533881083,-36.3857400536,4.09051357105));
#69409=CARTESIAN_POINT('Ctrl Pts',(-6.68670547342,-36.3112466293,4.02856141623));
#69410=CARTESIAN_POINT('Ctrl Pts',(-6.7390418526,-36.2742356128,3.95018063176));
#69411=CARTESIAN_POINT('Ctrl Pts',(-6.79137823178,-36.2742356128,3.87179984728));
#69412=CARTESIAN_POINT('Ctrl Pts',(-6.57452017565,-36.5742356128,4.08772991919));
#69413=CARTESIAN_POINT('Ctrl Pts',(-6.57452017565,-36.4799878332,4.08772991919));
#69414=CARTESIAN_POINT('Ctrl Pts',(-6.58892710136,-36.3857400536,4.05284637296));
#69415=CARTESIAN_POINT('Ctrl Pts',(-6.61792442226,-36.3112466293,3.98263496631));
#69416=CARTESIAN_POINT('Ctrl Pts',(-6.65461133659,-36.2742356128,3.89380472879));
#69417=CARTESIAN_POINT('Ctrl Pts',(-6.69129825092,-36.2742356128,3.80497449128));
#69418=CARTESIAN_POINT('Ctrl Pts',(-6.5160654267,-36.5742356128,4.06685309219));
#69419=CARTESIAN_POINT('Ctrl Pts',(-6.51606545157,-36.4799878341,4.06685311826));
#69420=CARTESIAN_POINT('Ctrl Pts',(-6.52325959788,-36.3857400553,4.0293608744));
#69421=CARTESIAN_POINT('Ctrl Pts',(-6.53773954623,-36.3112466313,3.95389885357));
#69422=CARTESIAN_POINT('Ctrl Pts',(-6.55605928475,-36.2742356142,3.85842559837));
#69423=CARTESIAN_POINT('Ctrl Pts',(-6.57437901362,-36.2742356128,3.76295233242));
#69424=CARTESIAN_POINT('Ctrl Pts',(-6.45374447685,-36.5742356128,4.06145161999));
#69425=CARTESIAN_POINT('Ctrl Pts',(-6.45374450233,-36.4799878332,4.06145160386));
#69426=CARTESIAN_POINT('Ctrl Pts',(-6.45313203559,-36.3857400535,4.02328625262));
#69427=CARTESIAN_POINT('Ctrl Pts',(-6.45189903265,-36.3112466293,3.94646790973));
#69428=CARTESIAN_POINT('Ctrl Pts',(-6.45033914294,-36.2742356128,3.84927935169));
#69429=CARTESIAN_POINT('Ctrl Pts',(-6.448779243,-36.2742356128,3.75209080017));
#69430=CARTESIAN_POINT('Ctrl Pts',(-6.31228390912,-36.5742356128,4.0856584563));
#69431=CARTESIAN_POINT('Ctrl Pts',(-6.31228387569,-36.4799878333,4.08565847747));
#69432=CARTESIAN_POINT('Ctrl Pts',(-6.29422735035,-36.3857400538,4.05052572546));
#69433=CARTESIAN_POINT('Ctrl Pts',(-6.25788474007,-36.3112466295,3.97981475152));
#69434=CARTESIAN_POINT('Ctrl Pts',(-6.21190456653,-36.2742356129,3.89035159857));
#69435=CARTESIAN_POINT('Ctrl Pts',(-6.16592440644,-36.2742356128,3.80088843706));
#69436=CARTESIAN_POINT('Ctrl Pts',(-6.20284603213,-36.5742356128,4.18404937306));
#69437=CARTESIAN_POINT('Ctrl Pts',(-6.202846076,-36.4799878331,4.18404934528));
#69438=CARTESIAN_POINT('Ctrl Pts',(-6.17143035383,-36.3857400534,4.16092715811));
#69439=CARTESIAN_POINT('Ctrl Pts',(-6.10819814971,-36.3112466292,4.1143857057));
#69440=CARTESIAN_POINT('Ctrl Pts',(-6.02819808562,-36.2742356127,4.05550338866));
#69441=CARTESIAN_POINT('Ctrl Pts',(-5.94819800384,-36.2742356128,3.99662108289));
#69442=CARTESIAN_POINT('Ctrl Pts',(-6.16233508317,-36.5742356128,4.25881330688));
#69443=CARTESIAN_POINT('Ctrl Pts',(-6.16233507193,-36.4799878312,4.25881328382));
#69444=CARTESIAN_POINT('Ctrl Pts',(-6.12578886815,-36.3857400495,4.24495014557));
#69445=CARTESIAN_POINT('Ctrl Pts',(-6.05223285478,-36.3112466242,4.21705793513));
#69446=CARTESIAN_POINT('Ctrl Pts',(-5.95917030134,-36.2742356096,4.1817647567));
#69447=CARTESIAN_POINT('Ctrl Pts',(-5.86610775343,-36.2742356128,4.14647158762));
#69448=CARTESIAN_POINT('Ctrl Pts',(-6.14934204931,-36.5742356128,4.34057228077));
#69449=CARTESIAN_POINT('Ctrl Pts',(-6.14934204855,-36.4799878345,4.34057227621));
#69450=CARTESIAN_POINT('Ctrl Pts',(-6.11125741298,-36.3857400562,4.33695823749));
#69451=CARTESIAN_POINT('Ctrl Pts',(-6.03460182449,-36.3112466325,4.32967707355));
#69452=CARTESIAN_POINT('Ctrl Pts',(-5.93761903844,-36.2742356148,4.32046804105));
#69453=CARTESIAN_POINT('Ctrl Pts',(-5.840636252,-36.2742356128,4.31125901017));
#69454=CARTESIAN_POINT('Ctrl Pts',(-6.16208308569,-36.5742356128,4.41893339446));
#69455=CARTESIAN_POINT('Ctrl Pts',(-6.1620830857,-36.4799878332,4.41893339453));
#69456=CARTESIAN_POINT('Ctrl Pts',(-6.12555180375,-36.3857400535,4.42487314505));
#69457=CARTESIAN_POINT('Ctrl Pts',(-6.05202395871,-36.3112466292,4.43682829772));
#69458=CARTESIAN_POINT('Ctrl Pts',(-5.95899781312,-36.2742356128,4.45195374807));
#69459=CARTESIAN_POINT('Ctrl Pts',(-5.86597166755,-36.2742356128,4.4670791984));
#69460=CARTESIAN_POINT('',(-6.62478636300403,-36.5742356128,4.12129363280448));
#69461=CARTESIAN_POINT('Origin',(-6.7901996463368,-36.5721143211899,3.87356359757439));
#69462=CARTESIAN_POINT('Ctrl Pts',(-6.62478636278,-36.5742356128,4.12129363314));
#69463=CARTESIAN_POINT('Ctrl Pts',(-6.50898576372,-36.5742356128,4.04397131362));
#69464=CARTESIAN_POINT('Ctrl Pts',(-6.34774592774,-36.5742356128,4.03257337207));
#69465=CARTESIAN_POINT('Ctrl Pts',(-6.19622108576,-36.5742356128,4.13004365321));
#69466=CARTESIAN_POINT('Ctrl Pts',(-6.13973650651,-36.5742356128,4.28149559307));
#69467=CARTESIAN_POINT('Ctrl Pts',(-6.16208308783,-36.5742356128,4.4189333977));
#69468=CARTESIAN_POINT('Ctrl Pts',(-5.86597167956,-38.2742356128,4.46707920117));
#69469=CARTESIAN_POINT('Ctrl Pts',(-5.95899782099,-38.2742356128,4.4519537493));
#69470=CARTESIAN_POINT('Ctrl Pts',(-6.05202396243,-38.2372245963,4.43682829744));
#69471=CARTESIAN_POINT('Ctrl Pts',(-6.12555180416,-38.1627311721,4.42487314362));
#69472=CARTESIAN_POINT('Ctrl Pts',(-6.16208308448,-38.0684833924,4.41893339256));
#69473=CARTESIAN_POINT('Ctrl Pts',(-6.16208308448,-37.9742356128,4.41893339256));
#69474=CARTESIAN_POINT('Ctrl Pts',(-5.84345320673,-38.2742356128,4.32858436112));
#69475=CARTESIAN_POINT('Ctrl Pts',(-5.93999533685,-38.2742356128,4.33508315368));
#69476=CARTESIAN_POINT('Ctrl Pts',(-6.03653746697,-38.2372245963,4.34158194625));
#69477=CARTESIAN_POINT('Ctrl Pts',(-6.11284466996,-38.1627311721,4.34672039209));
#69478=CARTESIAN_POINT('Ctrl Pts',(-6.15075635123,-38.0684833924,4.34927066034));
#69479=CARTESIAN_POINT('Ctrl Pts',(-6.15075635123,-37.9742356128,4.34927066034));
#69480=CARTESIAN_POINT('Ctrl Pts',(-5.86108700083,-38.2742356128,4.1830357728));
#69481=CARTESIAN_POINT('Ctrl Pts',(-5.9549289869,-38.2742356128,4.21254028592));
#69482=CARTESIAN_POINT('Ctrl Pts',(-6.04877097298,-38.2372245963,4.24204479904));
#69483=CARTESIAN_POINT('Ctrl Pts',(-6.12294317876,-38.1627311721,4.26536245256));
#69484=CARTESIAN_POINT('Ctrl Pts',(-6.1597953199,-38.0684833924,4.27695155493));
#69485=CARTESIAN_POINT('Ctrl Pts',(-6.1597953199,-37.9742356128,4.27695155493));
#69486=CARTESIAN_POINT('Ctrl Pts',(-5.92292196944,-38.2742356128,4.04703912854));
#69487=CARTESIAN_POINT('Ctrl Pts',(-6.00693080322,-38.2742356128,4.09800013468));
#69488=CARTESIAN_POINT('Ctrl Pts',(-6.09093963701,-38.2372245963,4.14896114082));
#69489=CARTESIAN_POINT('Ctrl Pts',(-6.15734124187,-38.1627311721,4.18924200394));
#69490=CARTESIAN_POINT('Ctrl Pts',(-6.19033039264,-38.0684833924,4.20925304918));
#69491=CARTESIAN_POINT('Ctrl Pts',(-6.19033039264,-37.9742356128,4.20925304918));
#69492=CARTESIAN_POINT('Ctrl Pts',(-6.11534148986,-38.2742356128,3.83026274895));
#69493=CARTESIAN_POINT('Ctrl Pts',(-6.16918512024,-38.2742356128,3.91514701063));
#69494=CARTESIAN_POINT('Ctrl Pts',(-6.22302875062,-38.2372245963,4.00003127231));
#69495=CARTESIAN_POINT('Ctrl Pts',(-6.26558574119,-38.1627311721,4.0671224893));
#69496=CARTESIAN_POINT('Ctrl Pts',(-6.28673108844,-38.0684833924,4.10045774569));
#69497=CARTESIAN_POINT('Ctrl Pts',(-6.28673108844,-37.9742356128,4.10045774569));
#69498=CARTESIAN_POINT('Ctrl Pts',(-6.39337248546,-38.2742356128,3.74948730929));
#69499=CARTESIAN_POINT('Ctrl Pts',(-6.40368458266,-38.2742356128,3.84705936306));
#69500=CARTESIAN_POINT('Ctrl Pts',(-6.41399667986,-38.2372245963,3.94463141684));
#69501=CARTESIAN_POINT('Ctrl Pts',(-6.4221483252,-38.1627311721,4.02175362115));
#69502=CARTESIAN_POINT('Ctrl Pts',(-6.42619691032,-38.0684833924,4.0600688026));
#69503=CARTESIAN_POINT('Ctrl Pts',(-6.42619691032,-37.9742356128,4.0600688026));
#69504=CARTESIAN_POINT('Ctrl Pts',(-6.53973745527,-38.2742356128,3.75112508254));
#69505=CARTESIAN_POINT('Ctrl Pts',(-6.52687581649,-38.2742356128,3.84847995905));
#69506=CARTESIAN_POINT('Ctrl Pts',(-6.51401417772,-38.2372245963,3.94583483556));
#69507=CARTESIAN_POINT('Ctrl Pts',(-6.50384486271,-38.1627311721,4.02278167233));
#69508=CARTESIAN_POINT('Ctrl Pts',(-6.49879758752,-38.0684833924,4.06101527916));
#69509=CARTESIAN_POINT('Ctrl Pts',(-6.49879758752,-37.9742356128,4.06101527916));
#69510=CARTESIAN_POINT('Ctrl Pts',(-6.67670923675,-38.2742356128,3.79523312185));
#69511=CARTESIAN_POINT('Ctrl Pts',(-6.64230360047,-38.2742356128,3.88558661323));
#69512=CARTESIAN_POINT('Ctrl Pts',(-6.60789796419,-38.2372245963,3.97594010461));
#69513=CARTESIAN_POINT('Ctrl Pts',(-6.58070607097,-38.1627311721,4.04735711157));
#69514=CARTESIAN_POINT('Ctrl Pts',(-6.56719269506,-38.0684833924,4.08283721742));
#69515=CARTESIAN_POINT('Ctrl Pts',(-6.56719269506,-37.9742356128,4.08283721742));
#69516=CARTESIAN_POINT('Ctrl Pts',(-6.79137823178,-38.2742356128,3.87179984728));
#69517=CARTESIAN_POINT('Ctrl Pts',(-6.7390418526,-38.2742356128,3.95018063176));
#69518=CARTESIAN_POINT('Ctrl Pts',(-6.68670547342,-38.2372245963,4.02856141623));
#69519=CARTESIAN_POINT('Ctrl Pts',(-6.64533881083,-38.1627311721,4.09051357105));
#69520=CARTESIAN_POINT('Ctrl Pts',(-6.62478636278,-38.0684833924,4.12129363314));
#69521=CARTESIAN_POINT('Ctrl Pts',(-6.62478636278,-37.9742356128,4.12129363314));
#69522=CARTESIAN_POINT('',(-6.62478636278,-37.9742356128,4.12129363314));
#69523=CARTESIAN_POINT('Origin',(-6.79020165742271,-37.9763569229,3.87356496908019));
#69524=CARTESIAN_POINT('Ctrl Pts',(-6.62478636278,-37.9742356128,4.12129363314));
#69525=CARTESIAN_POINT('Ctrl Pts',(-6.60980787112068,-37.9742356128,4.11129220199465));
#69526=CARTESIAN_POINT('Ctrl Pts',(-6.59393742031848,-37.9742356128,4.10263571211049));
#69527=CARTESIAN_POINT('Ctrl Pts',(-6.57743087233442,-37.9742356128,4.09546961237743));
#69528=CARTESIAN_POINT('Ctrl Pts',(-6.56094526970541,-37.9742356128,4.08831260579356));
#69529=CARTESIAN_POINT('Ctrl Pts',(-6.54382543811632,-37.9742356128,4.08264228477619));
#69530=CARTESIAN_POINT('Ctrl Pts',(-6.52633933526977,-37.9742356128,4.0785532591173));
#69531=CARTESIAN_POINT('Ctrl Pts',(-6.5088749281894,-37.9742356128,4.07446930688987));
#69532=CARTESIAN_POINT('Ctrl Pts',(-6.49104541888437,-37.9742356128,4.07196278396557));
#69533=CARTESIAN_POINT('Ctrl Pts',(-6.47312694977236,-37.9742356128,4.07107677504198));
#69534=CARTESIAN_POINT('Ctrl Pts',(-6.45523981202579,-37.9742356128,4.0701923153506));
#69535=CARTESIAN_POINT('Ctrl Pts',(-6.4372642894345,-37.9742356128,4.07092273833882));
#69536=CARTESIAN_POINT('Ctrl Pts',(-6.4194803008611,-37.9742356128,4.07325923758356));
#69537=CARTESIAN_POINT('Ctrl Pts',(-6.401715949138,-37.9742356128,4.07559315689604));
#69538=CARTESIAN_POINT('Ctrl Pts',(-6.38414297337429,-37.9742356128,4.07952962384662));
#69539=CARTESIAN_POINT('Ctrl Pts',(-6.36704162076337,-37.9742356128,4.0850079039406));
#69540=CARTESIAN_POINT('Ctrl Pts',(-6.34996634542379,-37.9742356128,4.09047783039147));
#69541=CARTESIAN_POINT('Ctrl Pts',(-6.33336151916574,-37.9742356128,4.09748486400625));
#69542=CARTESIAN_POINT('Ctrl Pts',(-6.31750340617419,-37.9742356128,4.10591666015032));
#69543=CARTESIAN_POINT('Ctrl Pts',(-6.31105406776151,-37.9742356128,4.10934578862159));
#69544=CARTESIAN_POINT('Ctrl Pts',(-6.30472818010765,-37.9742356128,4.11300997159109));
#69545=CARTESIAN_POINT('Ctrl Pts',(-6.29854404488772,-37.9742356128,4.11689920017885));
#69546=CARTESIAN_POINT('Ctrl Pts',(-6.28358900896551,-37.9742356128,4.12630448502001));
#69547=CARTESIAN_POINT('Ctrl Pts',(-6.2694662070212,-37.9742356128,4.13702813937559));
#69548=CARTESIAN_POINT('Ctrl Pts',(-6.25640125842688,-37.9742356128,4.14889368279589));
#69549=CARTESIAN_POINT('Ctrl Pts',(-6.2431639186608,-37.9742356128,4.16091579131242));
#69550=CARTESIAN_POINT('Ctrl Pts',(-6.23101274439312,-37.9742356128,4.1741096572297));
#69551=CARTESIAN_POINT('Ctrl Pts',(-6.22013923191321,-37.9742356128,4.18825931672047));
#69552=CARTESIAN_POINT('Ctrl Pts',(-6.20915109541951,-37.9742356128,4.20255813599449));
#69553=CARTESIAN_POINT('Ctrl Pts',(-6.19946788747794,-37.9742356128,4.21783247671418));
#69554=CARTESIAN_POINT('Ctrl Pts',(-6.19124041418449,-37.9742356128,4.23383418171913));
#69555=CARTESIAN_POINT('Ctrl Pts',(-6.18294233481706,-37.9742356128,4.24997320926858));
#69556=CARTESIAN_POINT('Ctrl Pts',(-6.17612524468972,-37.9742356128,4.26685156098772));
#69557=CARTESIAN_POINT('Ctrl Pts',(-6.17089386489525,-37.9742356128,4.28419745826298));
#69558=CARTESIAN_POINT('Ctrl Pts',(-6.16566177951222,-37.9742356128,4.30154569508676));
#69559=CARTESIAN_POINT('Ctrl Pts',(-6.1620159041005,-37.9742356128,4.31936099759098));
#69560=CARTESIAN_POINT('Ctrl Pts',(-6.16000954443398,-37.9742356128,4.33736332366485));
#69561=CARTESIAN_POINT('Ctrl Pts',(-6.15801470288541,-37.9742356128,4.35526230191006));
#69562=CARTESIAN_POINT('Ctrl Pts',(-6.15764060490737,-37.9742356128,4.37334557885617));
#69563=CARTESIAN_POINT('Ctrl Pts',(-6.1588883338163,-37.9742356128,4.39133874672889));
#69564=CARTESIAN_POINT('Ctrl Pts',(-6.15952865917384,-37.9742356128,4.40057270898534));
#69565=CARTESIAN_POINT('Ctrl Pts',(-6.16059528794716,-37.9742356128,4.4097830074333));
#69566=CARTESIAN_POINT('Ctrl Pts',(-6.16208308448,-37.9742356128,4.41893339256));
#69567=CARTESIAN_POINT('Ctrl Pts',(-6.16208308783,-37.9742356128,4.4189333977));
#69568=CARTESIAN_POINT('Ctrl Pts',(-6.16208308783,-36.2942356128,4.4189333977));
#69569=CARTESIAN_POINT('Ctrl Pts',(-6.13973650651,-37.9742356128,4.28149559307));
#69570=CARTESIAN_POINT('Ctrl Pts',(-6.13973650651,-36.2942356128,4.28149559307));
#69571=CARTESIAN_POINT('Ctrl Pts',(-6.19622108576,-37.9742356128,4.13004365321));
#69572=CARTESIAN_POINT('Ctrl Pts',(-6.19622108576,-36.2942356128,4.13004365321));
#69573=CARTESIAN_POINT('Ctrl Pts',(-6.34774592774,-37.9742356128,4.03257337207));
#69574=CARTESIAN_POINT('Ctrl Pts',(-6.34774592774,-36.2942356128,4.03257337207));
#69575=CARTESIAN_POINT('Ctrl Pts',(-6.50898576372,-37.9742356128,4.04397131362));
#69576=CARTESIAN_POINT('Ctrl Pts',(-6.50898576372,-36.2942356128,4.04397131362));
#69577=CARTESIAN_POINT('Ctrl Pts',(-6.62478636278,-37.9742356128,4.12129363314));
#69578=CARTESIAN_POINT('Ctrl Pts',(-6.62478636278,-36.2942356128,4.12129363314));
#69579=CARTESIAN_POINT('',(-6.62478636278,-37.2742356128,4.12129363314));
#69580=CARTESIAN_POINT('Ctrl Pts',(-10.3257952821,-36.5742356128,3.01322822759));
#69581=CARTESIAN_POINT('Ctrl Pts',(-10.3257952821,-36.4799878332,3.01322822759));
#69582=CARTESIAN_POINT('Ctrl Pts',(-10.2942035846,-36.3857400536,2.99394663035));
#69583=CARTESIAN_POINT('Ctrl Pts',(-10.2306178216,-36.3112466293,2.95513785557));
#69584=CARTESIAN_POINT('Ctrl Pts',(-10.1501702245,-36.2742356128,2.90603767139));
#69585=CARTESIAN_POINT('Ctrl Pts',(-10.0697226274,-36.2742356128,2.85693748721));
#69586=CARTESIAN_POINT('Ctrl Pts',(-10.2120403388,-36.5742356128,3.19960862508));
#69587=CARTESIAN_POINT('Ctrl Pts',(-10.2120403388,-36.4799878332,3.19960862508));
#69588=CARTESIAN_POINT('Ctrl Pts',(-10.1811264858,-36.3857400536,3.17921642189));
#69589=CARTESIAN_POINT('Ctrl Pts',(-10.1189050443,-36.3112466293,3.13817229103));
#69590=CARTESIAN_POINT('Ctrl Pts',(-10.0401835634,-36.2742356128,3.08624397291));
#69591=CARTESIAN_POINT('Ctrl Pts',(-9.9614620825,-36.2742356128,3.0343156548));
#69592=CARTESIAN_POINT('Ctrl Pts',(-10.0867279364,-36.5742356128,3.38639921292));
#69593=CARTESIAN_POINT('Ctrl Pts',(-10.0867279138,-36.4799877817,3.38639925793));
#69594=CARTESIAN_POINT('Ctrl Pts',(-10.056625897,-36.3857399505,3.36477264615));
#69595=CARTESIAN_POINT('Ctrl Pts',(-9.99603849534,-36.3112465078,3.32124392015));
#69596=CARTESIAN_POINT('Ctrl Pts',(-9.91938440381,-36.2742355318,3.26617212038));
#69597=CARTESIAN_POINT('Ctrl Pts',(-9.84273034735,-36.2742356128,3.21110032106));
#69598=CARTESIAN_POINT('Ctrl Pts',(-9.94731298405,-36.5742356128,3.57262583962));
#69599=CARTESIAN_POINT('Ctrl Pts',(-9.94731297208,-36.4799878487,3.57262583568));
#69600=CARTESIAN_POINT('Ctrl Pts',(-9.91847739878,-36.3857400847,3.54921512866));
#69601=CARTESIAN_POINT('Ctrl Pts',(-9.86043899652,-36.3112466659,3.50209555723));
#69602=CARTESIAN_POINT('Ctrl Pts',(-9.78700982899,-36.2742356372,3.44248069278));
#69603=CARTESIAN_POINT('Ctrl Pts',(-9.7135806598,-36.2742356128,3.38286582323));
#69604=CARTESIAN_POINT('Ctrl Pts',(-9.66551121862,-36.5742356128,3.88595497216));
#69605=CARTESIAN_POINT('Ctrl Pts',(-9.66551122768,-36.4799878215,3.88595497515));
#69606=CARTESIAN_POINT('Ctrl Pts',(-9.63981184426,-36.3857400301,3.85895077503));
#69607=CARTESIAN_POINT('Ctrl Pts',(-9.58808574642,-36.3112466017,3.80459843069));
#69608=CARTESIAN_POINT('Ctrl Pts',(-9.52264278801,-36.2742355944,3.73583279562));
#69609=CARTESIAN_POINT('Ctrl Pts',(-9.45719983084,-36.2742356128,3.66706716442));
#69610=CARTESIAN_POINT('Ctrl Pts',(-9.3190883522,-36.5742356128,4.15054175699));
#69611=CARTESIAN_POINT('Ctrl Pts',(-9.31908834533,-36.4799878421,4.15054175473));
#69612=CARTESIAN_POINT('Ctrl Pts',(-9.29825794524,-36.3857400714,4.11976487501));
#69613=CARTESIAN_POINT('Ctrl Pts',(-9.2563318491,-36.3112466503,4.05781912505));
#69614=CARTESIAN_POINT('Ctrl Pts',(-9.20328768523,-36.2742356268,3.97944644413));
#69615=CARTESIAN_POINT('Ctrl Pts',(-9.15024352041,-36.2742356128,3.9010737603));
#69616=CARTESIAN_POINT('Ctrl Pts',(-9.15760248753,-36.5742356128,4.25148215543));
#69617=CARTESIAN_POINT('Ctrl Pts',(-9.15760248541,-36.4799878223,4.2514821194));
#69618=CARTESIAN_POINT('Ctrl Pts',(-9.13915536063,-36.3857400317,4.2191945066));
#69619=CARTESIAN_POINT('Ctrl Pts',(-9.10202619378,-36.3112466035,4.15420811433));
#69620=CARTESIAN_POINT('Ctrl Pts',(-9.05505101001,-36.2742355956,4.07198848278));
#69621=CARTESIAN_POINT('Ctrl Pts',(-9.00807582956,-36.2742356128,3.98976887128));
#69622=CARTESIAN_POINT('Ctrl Pts',(-8.57636643433,-36.5742356128,4.53983021603));
#69623=CARTESIAN_POINT('Ctrl Pts',(-8.57636643948,-36.4799878598,4.53983030324));
#69624=CARTESIAN_POINT('Ctrl Pts',(-8.56686869878,-36.3857401067,4.50309713161));
#69625=CARTESIAN_POINT('Ctrl Pts',(-8.54775216416,-36.3112466919,4.42916277982));
#69626=CARTESIAN_POINT('Ctrl Pts',(-8.52356628354,-36.2742356545,4.33562228694));
#69627=CARTESIAN_POINT('Ctrl Pts',(-8.49938039487,-36.2742356128,4.24208174555));
#69628=CARTESIAN_POINT('Ctrl Pts',(-7.90756140161,-36.5742356128,4.62319204336));
#69629=CARTESIAN_POINT('Ctrl Pts',(-7.90756138915,-36.479987769,4.62319183227));
#69630=CARTESIAN_POINT('Ctrl Pts',(-7.90907281157,-36.3857399251,4.58492140719));
#69631=CARTESIAN_POINT('Ctrl Pts',(-7.91211511531,-36.3112464779,4.50789350029));
#69632=CARTESIAN_POINT('Ctrl Pts',(-7.91596412286,-36.2742355119,4.41043924037));
#69633=CARTESIAN_POINT('Ctrl Pts',(-7.91981314987,-36.2742356128,4.31298509787));
#69634=CARTESIAN_POINT('Ctrl Pts',(-7.427051153,-36.5742356128,4.54976665456));
#69635=CARTESIAN_POINT('Ctrl Pts',(-7.42705185339,-36.4799878489,4.54976712257));
#69636=CARTESIAN_POINT('Ctrl Pts',(-7.43643206769,-36.3857400849,4.512928851));
#69637=CARTESIAN_POINT('Ctrl Pts',(-7.4553103639,-36.3112466662,4.43878203837));
#69638=CARTESIAN_POINT('Ctrl Pts',(-7.47919473941,-36.2742356374,4.34497270415));
#69639=CARTESIAN_POINT('Ctrl Pts',(-7.50307884797,-36.2742356128,4.25116318014));
#69640=CARTESIAN_POINT('Ctrl Pts',(-6.99795842984,-36.5742356128,4.37046697706));
#69641=CARTESIAN_POINT('Ctrl Pts',(-6.99795797817,-36.4799878293,4.37046667454));
#69642=CARTESIAN_POINT('Ctrl Pts',(-7.01351947686,-36.3857400458,4.33635407281));
#69643=CARTESIAN_POINT('Ctrl Pts',(-7.04484172418,-36.3112466201,4.26769510081));
#69644=CARTESIAN_POINT('Ctrl Pts',(-7.08447015303,-36.2742356067,4.18082901477));
#69645=CARTESIAN_POINT('Ctrl Pts',(-7.1240987555,-36.2742356128,4.09396304787));
#69646=CARTESIAN_POINT('Ctrl Pts',(-6.62478625212,-36.5742356128,4.12129355731));
#69647=CARTESIAN_POINT('Ctrl Pts',(-6.6247862495,-36.4799878332,4.12129355555));
#69648=CARTESIAN_POINT('Ctrl Pts',(-6.64533862663,-36.3857400536,4.0905134461));
#69649=CARTESIAN_POINT('Ctrl Pts',(-6.68670514971,-36.3112466293,4.02856119812));
#69650=CARTESIAN_POINT('Ctrl Pts',(-6.73904135397,-36.2742356128,3.95018029684));
#69651=CARTESIAN_POINT('Ctrl Pts',(-6.79137755926,-36.2742356128,3.87179939627));
#69652=CARTESIAN_POINT('',(-10.3257952821,-36.5742356128,3.01322822759));
#69653=CARTESIAN_POINT('Origin',(-10.0715345021286,-36.5721143191909,2.85804066652907));
#69654=CARTESIAN_POINT('Ctrl Pts',(-10.3257952821,-36.5742356128,3.01322822759));
#69655=CARTESIAN_POINT('Ctrl Pts',(-10.24741676,-36.5742356128,3.14164655991));
#69656=CARTESIAN_POINT('Ctrl Pts',(-10.163703376,-36.5742356128,3.27006200044));
#69657=CARTESIAN_POINT('Ctrl Pts',(-10.0727130885,-36.5742356128,3.39989142333));
#69658=CARTESIAN_POINT('Ctrl Pts',(-9.92328269257,-36.5742356128,3.5920488793));
#69659=CARTESIAN_POINT('Ctrl Pts',(-9.75297759192,-36.5742356128,3.77433260224));
#69660=CARTESIAN_POINT('Ctrl Pts',(-9.69216005671,-36.5742356128,3.83525523444));
#69661=CARTESIAN_POINT('Ctrl Pts',(-9.50104385577,-36.5742356128,4.01328807602));
#69662=CARTESIAN_POINT('Ctrl Pts',(-9.28446203337,-36.5742356128,4.17257256592));
#69663=CARTESIAN_POINT('Ctrl Pts',(-9.12906626269,-36.5742356128,4.26637622783));
#69664=CARTESIAN_POINT('Ctrl Pts',(-8.80081499429,-36.5742356128,4.42491856124));
#69665=CARTESIAN_POINT('Ctrl Pts',(-8.44551261186,-36.5742356128,4.51817058272));
#69666=CARTESIAN_POINT('Ctrl Pts',(-8.26232955523,-36.5742356128,4.54692356056));
#69667=CARTESIAN_POINT('Ctrl Pts',(-7.98526439172,-36.5742356128,4.56199873534));
#69668=CARTESIAN_POINT('Ctrl Pts',(-7.71036083894,-36.5742356128,4.53610818987));
#69669=CARTESIAN_POINT('Ctrl Pts',(-7.61904353259,-36.5742356128,4.52294971153));
#69670=CARTESIAN_POINT('Ctrl Pts',(-7.35028595871,-36.5742356128,4.47075138071));
#69671=CARTESIAN_POINT('Ctrl Pts',(-7.09318322917,-36.5742356128,4.3815910145));
#69672=CARTESIAN_POINT('Ctrl Pts',(-6.92865784201,-36.5742356128,4.30723684413));
#69673=CARTESIAN_POINT('Ctrl Pts',(-6.77209862643,-36.5742356128,4.21965690596));
#69674=CARTESIAN_POINT('Ctrl Pts',(-6.62478636278,-36.5742356128,4.12129363314));
#69675=CARTESIAN_POINT('Ctrl Pts',(-6.79137909539,-38.2742356128,3.87180043587));
#69676=CARTESIAN_POINT('Ctrl Pts',(-6.73904267861,-38.2742356128,3.95018119693));
#69677=CARTESIAN_POINT('Ctrl Pts',(-6.68670626183,-38.2372245963,4.02856195799));
#69678=CARTESIAN_POINT('Ctrl Pts',(-6.64533956952,-38.1627311721,4.0905140943));
#69679=CARTESIAN_POINT('Ctrl Pts',(-6.62478710671,-38.0684833924,4.12129414719));
#69680=CARTESIAN_POINT('Ctrl Pts',(-6.62478710671,-37.9742356128,4.12129414719));
#69681=CARTESIAN_POINT('Ctrl Pts',(-7.1049579039,-38.2742356128,4.08118318573));
#69682=CARTESIAN_POINT('Ctrl Pts',(-7.06458024318,-38.2742356128,4.16754907896));
#69683=CARTESIAN_POINT('Ctrl Pts',(-7.02420258246,-38.2372245963,4.2539149722));
#69684=CARTESIAN_POINT('Ctrl Pts',(-6.99228789916,-38.1627311721,4.32217842764));
#69685=CARTESIAN_POINT('Ctrl Pts',(-6.97643181802,-38.0684833924,4.35609436218));
#69686=CARTESIAN_POINT('Ctrl Pts',(-6.97643181802,-37.9742356128,4.35609436218));
#69687=CARTESIAN_POINT('Ctrl Pts',(-7.45951427977,-38.2742356128,4.2326662718));
#69688=CARTESIAN_POINT('Ctrl Pts',(-7.43382029577,-38.2742356128,4.32566174563));
#69689=CARTESIAN_POINT('Ctrl Pts',(-7.40812631176,-38.2372245963,4.41865721947));
#69690=CARTESIAN_POINT('Ctrl Pts',(-7.38781807594,-38.1627311721,4.49216101308));
#69691=CARTESIAN_POINT('Ctrl Pts',(-7.37772778853,-38.0684833924,4.52868005872));
#69692=CARTESIAN_POINT('Ctrl Pts',(-7.37772778853,-37.9742356128,4.52868005872));
#69693=CARTESIAN_POINT('Ctrl Pts',(-7.84730605121,-38.2742356128,4.30154970059));
#69694=CARTESIAN_POINT('Ctrl Pts',(-7.84002374033,-38.2742356128,4.39837872821));
#69695=CARTESIAN_POINT('Ctrl Pts',(-7.83274142945,-38.2372245963,4.49520775584));
#69696=CARTESIAN_POINT('Ctrl Pts',(-7.82698541779,-38.1627311721,4.57174135372));
#69697=CARTESIAN_POINT('Ctrl Pts',(-7.82412573574,-38.0684833924,4.60976606821));
#69698=CARTESIAN_POINT('Ctrl Pts',(-7.82412573574,-37.9742356128,4.60976606821));
#69699=CARTESIAN_POINT('Ctrl Pts',(-8.42919235133,-38.2742356128,4.25742949913));
#69700=CARTESIAN_POINT('Ctrl Pts',(-8.44994916242,-38.2742356128,4.35179273091));
#69701=CARTESIAN_POINT('Ctrl Pts',(-8.4707059735,-38.2372245963,4.4461559627));
#69702=CARTESIAN_POINT('Ctrl Pts',(-8.4871121894,-38.1627311721,4.52074066283));
#69703=CARTESIAN_POINT('Ctrl Pts',(-8.49526333308,-38.0684833924,4.55779699483));
#69704=CARTESIAN_POINT('Ctrl Pts',(-8.49526333308,-37.9742356128,4.55779699483));
#69705=CARTESIAN_POINT('Ctrl Pts',(-8.948859956,-38.2742356128,4.02576580976));
#69706=CARTESIAN_POINT('Ctrl Pts',(-8.99328098916,-38.2742356128,4.10956686635));
#69707=CARTESIAN_POINT('Ctrl Pts',(-9.03770202233,-38.2372245963,4.19336792295));
#69708=CARTESIAN_POINT('Ctrl Pts',(-9.07281237888,-38.1627311721,4.25960424824));
#69709=CARTESIAN_POINT('Ctrl Pts',(-9.0902564961,-38.0684833924,4.29251285762));
#69710=CARTESIAN_POINT('Ctrl Pts',(-9.0902564961,-37.9742356128,4.29251285762));
#69711=CARTESIAN_POINT('Ctrl Pts',(-9.11396067931,-38.2742356128,3.92853263445));
#69712=CARTESIAN_POINT('Ctrl Pts',(-9.16552913778,-38.2742356128,4.00804487662));
#69713=CARTESIAN_POINT('Ctrl Pts',(-9.21709759625,-38.2372245963,4.0875571188));
#69714=CARTESIAN_POINT('Ctrl Pts',(-9.2578573361,-38.1627311721,4.1504035075));
#69715=CARTESIAN_POINT('Ctrl Pts',(-9.27810818078,-38.0684833924,4.18162796201));
#69716=CARTESIAN_POINT('Ctrl Pts',(-9.27810818078,-37.9742356128,4.18162796201));
#69717=CARTESIAN_POINT('Ctrl Pts',(-9.44245605888,-38.2742356128,3.68354837841));
#69718=CARTESIAN_POINT('Ctrl Pts',(-9.50744911367,-38.2742356128,3.7528343336));
#69719=CARTESIAN_POINT('Ctrl Pts',(-9.57244216847,-38.2372245963,3.82212028879));
#69720=CARTESIAN_POINT('Ctrl Pts',(-9.62381261275,-38.1627311721,3.87688397742));
#69721=CARTESIAN_POINT('Ctrl Pts',(-9.64933537762,-38.0684833924,3.90409242352));
#69722=CARTESIAN_POINT('Ctrl Pts',(-9.64933537762,-37.9742356128,3.90409242352));
#69723=CARTESIAN_POINT('Ctrl Pts',(-9.71422494881,-38.2742356128,3.38199158831));
#69724=CARTESIAN_POINT('Ctrl Pts',(-9.78766313637,-38.2742356128,3.44159039714));
#69725=CARTESIAN_POINT('Ctrl Pts',(-9.86110132392,-38.2372245963,3.50118920597));
#69726=CARTESIAN_POINT('Ctrl Pts',(-9.91914691568,-38.1627311721,3.54829598872));
#69727=CARTESIAN_POINT('Ctrl Pts',(-9.94798596003,-38.0684833924,3.57170048887));
#69728=CARTESIAN_POINT('Ctrl Pts',(-9.94798596003,-37.9742356128,3.57170048887));
#69729=CARTESIAN_POINT('Ctrl Pts',(-9.84307440206,-38.2742356128,3.21058575408));
#69730=CARTESIAN_POINT('Ctrl Pts',(-9.91972289161,-38.2742356128,3.26565161277));
#69731=CARTESIAN_POINT('Ctrl Pts',(-9.99637138116,-38.2372245963,3.32071747146));
#69732=CARTESIAN_POINT('Ctrl Pts',(-10.0569540934,-38.1627311721,3.36424190319));
#69733=CARTESIAN_POINT('Ctrl Pts',(-10.0870541219,-38.0684833924,3.3858658262));
#69734=CARTESIAN_POINT('Ctrl Pts',(-10.0870541219,-37.9742356128,3.3858658262));
#69735=CARTESIAN_POINT('Ctrl Pts',(-9.96162763734,-38.2742356128,3.03404440349));
#69736=CARTESIAN_POINT('Ctrl Pts',(-10.0403517579,-38.2742356128,3.08596839674));
#69737=CARTESIAN_POINT('Ctrl Pts',(-10.1190758784,-38.2372245963,3.13789239));
#69738=CARTESIAN_POINT('Ctrl Pts',(-10.181299565,-38.1627311721,3.17893284235));
#69739=CARTESIAN_POINT('Ctrl Pts',(-10.2122142958,-38.0684833924,3.19932360733));
#69740=CARTESIAN_POINT('Ctrl Pts',(-10.2122142958,-37.9742356128,3.19932360733));
#69741=CARTESIAN_POINT('Ctrl Pts',(-10.0697226274,-38.2742356128,2.85693748721));
#69742=CARTESIAN_POINT('Ctrl Pts',(-10.1501702245,-38.2742356128,2.90603767139));
#69743=CARTESIAN_POINT('Ctrl Pts',(-10.2306178216,-38.2372245963,2.95513785557));
#69744=CARTESIAN_POINT('Ctrl Pts',(-10.2942035846,-38.1627311721,2.99394663035));
#69745=CARTESIAN_POINT('Ctrl Pts',(-10.3257952821,-38.0684833924,3.01322822759));
#69746=CARTESIAN_POINT('Ctrl Pts',(-10.3257952821,-37.9742356128,3.01322822759));
#69747=CARTESIAN_POINT('',(-10.3257952821,-37.9742356128,3.01322822759));
#69748=CARTESIAN_POINT('Origin',(-10.0715328873088,-37.9763569037572,2.85804330597835));
#69749=CARTESIAN_POINT('Ctrl Pts',(-10.3257952821,-37.9742356128,3.01322822759));
#69750=CARTESIAN_POINT('Ctrl Pts',(-10.24741676,-37.9742356128,3.14164655991));
#69751=CARTESIAN_POINT('Ctrl Pts',(-10.163703376,-37.9742356128,3.27006200044));
#69752=CARTESIAN_POINT('Ctrl Pts',(-10.0727130885,-37.9742356128,3.39989142333));
#69753=CARTESIAN_POINT('Ctrl Pts',(-9.92328269257,-37.9742356128,3.5920488793));
#69754=CARTESIAN_POINT('Ctrl Pts',(-9.75297759192,-37.9742356128,3.77433260224));
#69755=CARTESIAN_POINT('Ctrl Pts',(-9.69216005671,-37.9742356128,3.83525523444));
#69756=CARTESIAN_POINT('Ctrl Pts',(-9.50104385577,-37.9742356128,4.01328807602));
#69757=CARTESIAN_POINT('Ctrl Pts',(-9.28446203337,-37.9742356128,4.17257256592));
#69758=CARTESIAN_POINT('Ctrl Pts',(-9.12906626269,-37.9742356128,4.26637622783));
#69759=CARTESIAN_POINT('Ctrl Pts',(-8.80081499429,-37.9742356128,4.42491856124));
#69760=CARTESIAN_POINT('Ctrl Pts',(-8.44551261186,-37.9742356128,4.51817058272));
#69761=CARTESIAN_POINT('Ctrl Pts',(-8.26232955523,-37.9742356128,4.54692356056));
#69762=CARTESIAN_POINT('Ctrl Pts',(-7.98526439172,-37.9742356128,4.56199873534));
#69763=CARTESIAN_POINT('Ctrl Pts',(-7.71036083894,-37.9742356128,4.53610818987));
#69764=CARTESIAN_POINT('Ctrl Pts',(-7.61904353259,-37.9742356128,4.52294971153));
#69765=CARTESIAN_POINT('Ctrl Pts',(-7.35028595871,-37.9742356128,4.47075138071));
#69766=CARTESIAN_POINT('Ctrl Pts',(-7.09318322917,-37.9742356128,4.3815910145));
#69767=CARTESIAN_POINT('Ctrl Pts',(-6.92865784201,-37.9742356128,4.30723684413));
#69768=CARTESIAN_POINT('Ctrl Pts',(-6.77209862643,-37.9742356128,4.21965690596));
#69769=CARTESIAN_POINT('Ctrl Pts',(-6.62478636278,-37.9742356128,4.12129363314));
#69770=CARTESIAN_POINT('Ctrl Pts',(-6.62478636278,-37.9742356128,4.12129363314));
#69771=CARTESIAN_POINT('Ctrl Pts',(-6.62478636278,-36.2942356128,4.12129363314));
#69772=CARTESIAN_POINT('Ctrl Pts',(-6.77209862643,-37.9742356128,4.21965690596));
#69773=CARTESIAN_POINT('Ctrl Pts',(-6.77209862643,-36.2942356128,4.21965690596));
#69774=CARTESIAN_POINT('Ctrl Pts',(-6.92865784201,-37.9742356128,4.30723684413));
#69775=CARTESIAN_POINT('Ctrl Pts',(-6.92865784201,-36.2942356128,4.30723684413));
#69776=CARTESIAN_POINT('Ctrl Pts',(-7.09318322917,-37.9742356128,4.3815910145));
#69777=CARTESIAN_POINT('Ctrl Pts',(-7.09318322917,-36.2942356128,4.3815910145));
#69778=CARTESIAN_POINT('Ctrl Pts',(-7.35028595871,-37.9742356128,4.47075138071));
#69779=CARTESIAN_POINT('Ctrl Pts',(-7.35028595871,-36.2942356128,4.47075138071));
#69780=CARTESIAN_POINT('Ctrl Pts',(-7.61904353259,-37.9742356128,4.52294971153));
#69781=CARTESIAN_POINT('Ctrl Pts',(-7.61904353259,-36.2942356128,4.52294971153));
#69782=CARTESIAN_POINT('Ctrl Pts',(-7.71036083894,-37.9742356128,4.53610818987));
#69783=CARTESIAN_POINT('Ctrl Pts',(-7.71036083894,-36.2942356128,4.53610818987));
#69784=CARTESIAN_POINT('Ctrl Pts',(-7.98526439172,-37.9742356128,4.56199873534));
#69785=CARTESIAN_POINT('Ctrl Pts',(-7.98526439172,-36.2942356128,4.56199873534));
#69786=CARTESIAN_POINT('Ctrl Pts',(-8.26232955523,-37.9742356128,4.54692356056));
#69787=CARTESIAN_POINT('Ctrl Pts',(-8.26232955523,-36.2942356128,4.54692356056));
#69788=CARTESIAN_POINT('Ctrl Pts',(-8.44551261186,-37.9742356128,4.51817058272));
#69789=CARTESIAN_POINT('Ctrl Pts',(-8.44551261186,-36.2942356128,4.51817058272));
#69790=CARTESIAN_POINT('Ctrl Pts',(-8.80081499429,-37.9742356128,4.42491856124));
#69791=CARTESIAN_POINT('Ctrl Pts',(-8.80081499429,-36.2942356128,4.42491856124));
#69792=CARTESIAN_POINT('Ctrl Pts',(-9.12906626269,-37.9742356128,4.26637622783));
#69793=CARTESIAN_POINT('Ctrl Pts',(-9.12906626269,-36.2942356128,4.26637622783));
#69794=CARTESIAN_POINT('Ctrl Pts',(-9.28446203337,-37.9742356128,4.17257256592));
#69795=CARTESIAN_POINT('Ctrl Pts',(-9.28446203337,-36.2942356128,4.17257256592));
#69796=CARTESIAN_POINT('Ctrl Pts',(-9.50104385577,-37.9742356128,4.01328807602));
#69797=CARTESIAN_POINT('Ctrl Pts',(-9.50104385577,-36.2942356128,4.01328807602));
#69798=CARTESIAN_POINT('Ctrl Pts',(-9.69216005671,-37.9742356128,3.83525523444));
#69799=CARTESIAN_POINT('Ctrl Pts',(-9.69216005671,-36.2942356128,3.83525523444));
#69800=CARTESIAN_POINT('Ctrl Pts',(-9.75297759192,-37.9742356128,3.77433260224));
#69801=CARTESIAN_POINT('Ctrl Pts',(-9.75297759192,-36.2942356128,3.77433260224));
#69802=CARTESIAN_POINT('Ctrl Pts',(-9.92328269257,-37.9742356128,3.5920488793));
#69803=CARTESIAN_POINT('Ctrl Pts',(-9.92328269257,-36.2942356128,3.5920488793));
#69804=CARTESIAN_POINT('Ctrl Pts',(-10.0727130885,-37.9742356128,3.39989142333));
#69805=CARTESIAN_POINT('Ctrl Pts',(-10.0727130885,-36.2942356128,3.39989142333));
#69806=CARTESIAN_POINT('Ctrl Pts',(-10.163703376,-37.9742356128,3.27006200044));
#69807=CARTESIAN_POINT('Ctrl Pts',(-10.163703376,-36.2942356128,3.27006200044));
#69808=CARTESIAN_POINT('Ctrl Pts',(-10.24741676,-37.9742356128,3.14164655991));
#69809=CARTESIAN_POINT('Ctrl Pts',(-10.24741676,-36.2942356128,3.14164655991));
#69810=CARTESIAN_POINT('Ctrl Pts',(-10.3257952821,-37.9742356128,3.01322822759));
#69811=CARTESIAN_POINT('Ctrl Pts',(-10.3257952821,-36.2942356128,3.01322822759));
#69812=CARTESIAN_POINT('',(-10.3257952821,-37.2742356128,3.01322822759));
#69813=CARTESIAN_POINT('Ctrl Pts',(-11.0450673741,-36.5742356128,0.800650704934));
#69814=CARTESIAN_POINT('Ctrl Pts',(-11.0450673741,-36.4799878332,0.800650704934));
#69815=CARTESIAN_POINT('Ctrl Pts',(-11.008502755,-36.3857400536,0.794919738554));
#69816=CARTESIAN_POINT('Ctrl Pts',(-10.9349078112,-36.3112466293,0.783384813269));
#69817=CARTESIAN_POINT('Ctrl Pts',(-10.8417967734,-36.2742356128,0.768791027219));
#69818=CARTESIAN_POINT('Ctrl Pts',(-10.7486857355,-36.2742356128,0.75419724117));
#69819=CARTESIAN_POINT('Ctrl Pts',(-11.0356958718,-36.5742356128,0.860442612609));
#69820=CARTESIAN_POINT('Ctrl Pts',(-11.0356958718,-36.4799878332,0.860442612609));
#69821=CARTESIAN_POINT('Ctrl Pts',(-10.9991532809,-36.3857400536,0.854571102129));
#69822=CARTESIAN_POINT('Ctrl Pts',(-10.9256026745,-36.3112466293,0.842753296288));
#69823=CARTESIAN_POINT('Ctrl Pts',(-10.8325477313,-36.2742356128,0.827801615647));
#69824=CARTESIAN_POINT('Ctrl Pts',(-10.7394927882,-36.2742356128,0.812849935018));
#69825=CARTESIAN_POINT('Ctrl Pts',(-11.026134227,-36.5742356128,0.919561027699));
#69826=CARTESIAN_POINT('Ctrl Pts',(-11.0261342139,-36.4799878338,0.919561111138));
#69827=CARTESIAN_POINT('Ctrl Pts',(-10.9896137808,-36.3857400548,0.913553049122));
#69828=CARTESIAN_POINT('Ctrl Pts',(-10.9161077872,-36.3112466308,0.901460304345));
#69829=CARTESIAN_POINT('Ctrl Pts',(-10.8231092957,-36.2742356138,0.886160722879));
#69830=CARTESIAN_POINT('Ctrl Pts',(-10.7301108089,-36.2742356128,0.870861108564));
#69831=CARTESIAN_POINT('Ctrl Pts',(-11.0156765092,-36.5742356128,0.982678343196));
#69832=CARTESIAN_POINT('Ctrl Pts',(-11.0156765148,-36.4799878335,0.982678307492));
#69833=CARTESIAN_POINT('Ctrl Pts',(-10.9791715737,-36.3857400541,0.976578280666));
#69834=CARTESIAN_POINT('Ctrl Pts',(-10.9056967395,-36.3112466299,0.964300575476));
#69835=CARTESIAN_POINT('Ctrl Pts',(-10.8127376585,-36.2742356132,0.9487670598));
#69836=CARTESIAN_POINT('Ctrl Pts',(-10.7197785752,-36.2742356128,0.933233558116));
#69837=CARTESIAN_POINT('Ctrl Pts',(-10.9943063871,-36.5742356128,1.10902865463));
#69838=CARTESIAN_POINT('Ctrl Pts',(-10.9943063815,-36.479987833,1.10902869053));
#69839=CARTESIAN_POINT('Ctrl Pts',(-10.957836371,-36.3857400532,1.10271910297));
#69840=CARTESIAN_POINT('Ctrl Pts',(-10.884431856,-36.3112466288,1.0900195227));
#69841=CARTESIAN_POINT('Ctrl Pts',(-10.791561749,-36.2742356125,1.07395221337));
#69842=CARTESIAN_POINT('Ctrl Pts',(-10.6986916443,-36.2742356128,1.05788488998));
#69843=CARTESIAN_POINT('Ctrl Pts',(-10.9728702198,-36.5742356128,1.22868657788));
#69844=CARTESIAN_POINT('Ctrl Pts',(-10.9728702255,-36.4799878335,1.2286865418));
#69845=CARTESIAN_POINT('Ctrl Pts',(-10.9364628515,-36.3857400541,1.22202580029));
#69846=CARTESIAN_POINT('Ctrl Pts',(-10.8631843933,-36.3112466299,1.20861952714));
#69847=CARTESIAN_POINT('Ctrl Pts',(-10.7704737642,-36.2742356132,1.19165816618));
#69848=CARTESIAN_POINT('Ctrl Pts',(-10.6777631327,-36.2742356128,1.17469681936));
#69849=CARTESIAN_POINT('Ctrl Pts',(-10.9617509373,-36.5742356128,1.28871328879));
#69850=CARTESIAN_POINT('Ctrl Pts',(-10.9617509376,-36.4799878316,1.28871328613));
#69851=CARTESIAN_POINT('Ctrl Pts',(-10.9253775233,-36.3857400503,1.28186748201));
#69852=CARTESIAN_POINT('Ctrl Pts',(-10.8521674238,-36.3112466254,1.26808868559));
#69853=CARTESIAN_POINT('Ctrl Pts',(-10.7595432847,-36.2742356102,1.2506559946));
#69854=CARTESIAN_POINT('Ctrl Pts',(-10.6669191464,-36.2742356128,1.23322330483));
#69855=CARTESIAN_POINT('Ctrl Pts',(-10.9262749306,-36.5742356128,1.47265339473));
#69856=CARTESIAN_POINT('Ctrl Pts',(-10.9262749299,-36.4799878366,1.47265340004));
#69857=CARTESIAN_POINT('Ctrl Pts',(-10.8900377752,-36.3857400603,1.46509591619));
#69858=CARTESIAN_POINT('Ctrl Pts',(-10.8171019319,-36.3112466372,1.44988468551));
#69859=CARTESIAN_POINT('Ctrl Pts',(-10.7248247757,-36.2742356181,1.43063969881));
#69860=CARTESIAN_POINT('Ctrl Pts',(-10.6325476177,-36.2742356128,1.41139470965));
#69861=CARTESIAN_POINT('Ctrl Pts',(-10.8845365863,-36.5742356128,1.66051012485));
#69862=CARTESIAN_POINT('Ctrl Pts',(-10.8845365878,-36.4799878265,1.66051011422));
#69863=CARTESIAN_POINT('Ctrl Pts',(-10.8485236903,-36.3857400402,1.65192611838));
#69864=CARTESIAN_POINT('Ctrl Pts',(-10.7760392139,-36.3112466136,1.6346488105));
#69865=CARTESIAN_POINT('Ctrl Pts',(-10.6843331221,-36.2742356023,1.61278986878));
#69866=CARTESIAN_POINT('Ctrl Pts',(-10.5926270337,-36.2742356128,1.59093093198));
#69867=CARTESIAN_POINT('Ctrl Pts',(-10.8528256956,-36.5742356128,1.78779287908));
#69868=CARTESIAN_POINT('Ctrl Pts',(-10.8528257075,-36.4799878307,1.78779285781));
#69869=CARTESIAN_POINT('Ctrl Pts',(-10.8170223835,-36.3857400485,1.77834284407));
#69870=CARTESIAN_POINT('Ctrl Pts',(-10.7449597336,-36.3112466233,1.75932244652));
#69871=CARTESIAN_POINT('Ctrl Pts',(-10.6537873116,-36.2742356088,1.73525820021));
#69872=CARTESIAN_POINT('Ctrl Pts',(-10.5626148864,-36.2742356128,1.71119396292));
#69873=CARTESIAN_POINT('Ctrl Pts',(-10.7586931318,-36.5742356128,2.11943860448));
#69874=CARTESIAN_POINT('Ctrl Pts',(-10.758693113,-36.4799878373,2.11943863814));
#69875=CARTESIAN_POINT('Ctrl Pts',(-10.7235741006,-36.3857400617,2.10755898422));
#69876=CARTESIAN_POINT('Ctrl Pts',(-10.6528887702,-36.3112466389,2.08364838728));
#69877=CARTESIAN_POINT('Ctrl Pts',(-10.5634589492,-36.2742356192,2.05339707211));
#69878=CARTESIAN_POINT('Ctrl Pts',(-10.4740291333,-36.2742356128,2.02314574267));
#69879=CARTESIAN_POINT('Ctrl Pts',(-10.6310539149,-36.5742356128,2.44887196143));
#69880=CARTESIAN_POINT('Ctrl Pts',(-10.6310539447,-36.4799878268,2.44887190815));
#69881=CARTESIAN_POINT('Ctrl Pts',(-10.5970339308,-36.3857400409,2.43409852045));
#69882=CARTESIAN_POINT('Ctrl Pts',(-10.5285606254,-36.3112466143,2.40436355679));
#69883=CARTESIAN_POINT('Ctrl Pts',(-10.4419293559,-36.2742356028,2.36674347238));
#69884=CARTESIAN_POINT('Ctrl Pts',(-10.3552980782,-36.2742356128,2.32912341055));
#69885=CARTESIAN_POINT('Ctrl Pts',(-10.5407851495,-36.5742356128,2.64396902292));
#69886=CARTESIAN_POINT('Ctrl Pts',(-10.5407850384,-36.4799878442,2.64396920253));
#69887=CARTESIAN_POINT('Ctrl Pts',(-10.5075973283,-36.3857400755,2.62740472217));
#69888=CARTESIAN_POINT('Ctrl Pts',(-10.440799126,-36.3112466551,2.59406493039));
#69889=CARTESIAN_POINT('Ctrl Pts',(-10.3562873645,-36.27423563,2.55188374368));
#69890=CARTESIAN_POINT('Ctrl Pts',(-10.2717756404,-36.2742356128,2.50970248388));
#69891=CARTESIAN_POINT('Ctrl Pts',(-10.4329248475,-36.5742356128,2.83770348479));
#69892=CARTESIAN_POINT('Ctrl Pts',(-10.432924939,-36.4799878331,2.83770333584));
#69893=CARTESIAN_POINT('Ctrl Pts',(-10.4006746925,-36.3857400534,2.81950071793));
#69894=CARTESIAN_POINT('Ctrl Pts',(-10.3357634803,-36.3112466291,2.78286358468));
#69895=CARTESIAN_POINT('Ctrl Pts',(-10.2536388298,-36.2742356127,2.73651111612));
#69896=CARTESIAN_POINT('Ctrl Pts',(-10.1715141437,-36.2742356128,2.69015870569));
#69897=CARTESIAN_POINT('Ctrl Pts',(-10.3257953578,-36.5742356128,3.01322810549));
#69898=CARTESIAN_POINT('Ctrl Pts',(-10.3257953569,-36.4799878332,3.01322810703));
#69899=CARTESIAN_POINT('Ctrl Pts',(-10.2942037404,-36.3857400536,2.99394637711));
#69900=CARTESIAN_POINT('Ctrl Pts',(-10.2306181415,-36.3112466294,2.9551373334));
#69901=CARTESIAN_POINT('Ctrl Pts',(-10.1501707528,-36.2742356129,2.90603680802));
#69902=CARTESIAN_POINT('Ctrl Pts',(-10.0697233643,-36.2742356128,2.85693628205));
#69903=CARTESIAN_POINT('',(-11.0450673734813,-36.5742356128,0.800650704837023));
#69904=CARTESIAN_POINT('Origin',(-10.7507814379643,-36.5721143212036,0.754525737239802));
#69905=CARTESIAN_POINT('Ctrl Pts',(-11.0450673741,-36.5742356128,0.800650704934));
#69906=CARTESIAN_POINT('Ctrl Pts',(-11.0322998283,-36.5742356128,0.882109994357));
#69907=CARTESIAN_POINT('Ctrl Pts',(-11.0192230843,-36.5742356128,0.962056438391));
#69908=CARTESIAN_POINT('Ctrl Pts',(-11.0034487645,-36.5742356128,1.05599081));
#69909=CARTESIAN_POINT('Ctrl Pts',(-10.9747007144,-36.5742356128,1.22147170177));
#69910=CARTESIAN_POINT('Ctrl Pts',(-10.9420747597,-36.5742356128,1.39194060497));
#69911=CARTESIAN_POINT('Ctrl Pts',(-10.9239906907,-36.5742356128,1.48074082922));
#69912=CARTESIAN_POINT('Ctrl Pts',(-10.8740649015,-36.5742356128,1.70707199422));
#69913=CARTESIAN_POINT('Ctrl Pts',(-10.8111933802,-36.5742356128,1.9383801789));
#69914=CARTESIAN_POINT('Ctrl Pts',(-10.7670166783,-36.5742356128,2.08017125701));
#69915=CARTESIAN_POINT('Ctrl Pts',(-10.6667840474,-36.5742356128,2.35918484011));
#69916=CARTESIAN_POINT('Ctrl Pts',(-10.5420136,-36.5742356128,2.63031881231));
#69917=CARTESIAN_POINT('Ctrl Pts',(-10.4735263391,-36.5742356128,2.76337956772));
#69918=CARTESIAN_POINT('Ctrl Pts',(-10.3992001828,-36.5742356128,2.89295886461));
#69919=CARTESIAN_POINT('Ctrl Pts',(-10.3257952821,-36.5742356128,3.01322822759));
#69920=CARTESIAN_POINT('Ctrl Pts',(-10.0697223221,-38.2742356128,2.85693798735));
#69921=CARTESIAN_POINT('Ctrl Pts',(-10.1501700117,-38.2742356128,2.90603801994));
#69922=CARTESIAN_POINT('Ctrl Pts',(-10.2306177012,-38.2372245963,2.95513805253));
#69923=CARTESIAN_POINT('Ctrl Pts',(-10.2942035374,-38.1627311721,2.9939467075));
#69924=CARTESIAN_POINT('Ctrl Pts',(-10.3257952712,-38.0684833924,3.01322824521));
#69925=CARTESIAN_POINT('Ctrl Pts',(-10.3257952712,-37.9742356128,3.01322824521));
#69926=CARTESIAN_POINT('Ctrl Pts',(-10.1868233028,-38.2742356128,2.66507503056));
#69927=CARTESIAN_POINT('Ctrl Pts',(-10.2691930709,-38.2742356128,2.71102584437));
#69928=CARTESIAN_POINT('Ctrl Pts',(-10.3515628389,-38.2372245963,2.75697665817));
#69929=CARTESIAN_POINT('Ctrl Pts',(-10.4166677835,-38.1627311721,2.79329633777));
#69930=CARTESIAN_POINT('Ctrl Pts',(-10.4490144177,-38.0684833924,2.81134101369));
#69931=CARTESIAN_POINT('Ctrl Pts',(-10.4490144177,-37.9742356128,2.81134101369));
#69932=CARTESIAN_POINT('Ctrl Pts',(-10.301618245,-38.2742356128,2.45520417407));
#69933=CARTESIAN_POINT('Ctrl Pts',(-10.3868740365,-38.2742356128,2.49608900873));
#69934=CARTESIAN_POINT('Ctrl Pts',(-10.472129828,-38.2372245963,2.5369738434));
#69935=CARTESIAN_POINT('Ctrl Pts',(-10.5395161398,-38.1627311721,2.56928895818));
#69936=CARTESIAN_POINT('Ctrl Pts',(-10.5729958579,-38.0684833924,2.58534464476));
#69937=CARTESIAN_POINT('Ctrl Pts',(-10.5729958579,-37.9742356128,2.58534464476));
#69938=CARTESIAN_POINT('Ctrl Pts',(-10.3925251896,-38.2742356128,2.24714722347));
#69939=CARTESIAN_POINT('Ctrl Pts',(-10.4800958587,-38.2742356128,2.28265349733));
#69940=CARTESIAN_POINT('Ctrl Pts',(-10.5676665277,-38.2372245963,2.31815977119));
#69941=CARTESIAN_POINT('Ctrl Pts',(-10.6368823272,-38.1627311721,2.34622398605));
#69942=CARTESIAN_POINT('Ctrl Pts',(-10.6712712865,-38.0684833924,2.36016720339));
#69943=CARTESIAN_POINT('Ctrl Pts',(-10.6712712865,-37.9742356128,2.36016720339));
#69944=CARTESIAN_POINT('Ctrl Pts',(-10.4951845718,-38.2742356128,1.95707474872));
#69945=CARTESIAN_POINT('Ctrl Pts',(-10.5850671643,-38.2742356128,1.98585046507));
#69946=CARTESIAN_POINT('Ctrl Pts',(-10.6749497569,-38.2372245963,2.01462618141));
#69947=CARTESIAN_POINT('Ctrl Pts',(-10.7459929506,-38.1627311721,2.03737048094));
#69948=CARTESIAN_POINT('Ctrl Pts',(-10.7812897498,-38.0684833924,2.04867069867));
#69949=CARTESIAN_POINT('Ctrl Pts',(-10.7812897498,-37.9742356128,2.04867069867));
#69950=CARTESIAN_POINT('Ctrl Pts',(-10.5724029544,-38.2742356128,1.66744116868));
#69951=CARTESIAN_POINT('Ctrl Pts',(-10.6637262076,-38.2742356128,1.69079424142));
#69952=CARTESIAN_POINT('Ctrl Pts',(-10.7550494608,-38.2372245963,1.71414731415));
#69953=CARTESIAN_POINT('Ctrl Pts',(-10.8272313361,-38.1627311721,1.7326055842));
#69954=CARTESIAN_POINT('Ctrl Pts',(-10.8630938978,-38.0684833924,1.74177630792));
#69955=CARTESIAN_POINT('Ctrl Pts',(-10.8630938978,-37.9742356128,1.74177630792));
#69956=CARTESIAN_POINT('Ctrl Pts',(-10.5899310768,-38.2742356128,1.59685627097));
#69957=CARTESIAN_POINT('Ctrl Pts',(-10.6815562054,-38.2742356128,1.61898136728));
#69958=CARTESIAN_POINT('Ctrl Pts',(-10.7731813341,-38.2372245963,1.64110646359));
#69959=CARTESIAN_POINT('Ctrl Pts',(-10.8456018157,-38.1627311721,1.65859413501));
#69960=CARTESIAN_POINT('Ctrl Pts',(-10.8815829196,-38.0684833924,1.66728263986));
#69961=CARTESIAN_POINT('Ctrl Pts',(-10.8815829196,-37.9742356128,1.66728263986));
#69962=CARTESIAN_POINT('Ctrl Pts',(-10.6184801248,-38.2742356128,1.47356398205));
#69963=CARTESIAN_POINT('Ctrl Pts',(-10.7105472499,-38.2742356128,1.49376689715));
#69964=CARTESIAN_POINT('Ctrl Pts',(-10.802614375,-38.2372245963,1.51396981225));
#69965=CARTESIAN_POINT('Ctrl Pts',(-10.8753842104,-38.1627311721,1.52993819193));
#69966=CARTESIAN_POINT('Ctrl Pts',(-10.9115388859,-38.0684833924,1.53787185811));
#69967=CARTESIAN_POINT('Ctrl Pts',(-10.9115388859,-37.9742356128,1.53787185811));
#69968=CARTESIAN_POINT('Ctrl Pts',(-10.6439064683,-38.2742356128,1.35095545652));
#69969=CARTESIAN_POINT('Ctrl Pts',(-10.7362898376,-38.2742356128,1.36962561802));
#69970=CARTESIAN_POINT('Ctrl Pts',(-10.828673207,-38.2372245963,1.38829577952));
#69971=CARTESIAN_POINT('Ctrl Pts',(-10.9016930018,-38.1627311721,1.40305267094));
#69972=CARTESIAN_POINT('Ctrl Pts',(-10.9379718661,-38.0684833924,1.41038442635));
#69973=CARTESIAN_POINT('Ctrl Pts',(-10.9379718661,-37.9742356128,1.41038442635));
#69974=CARTESIAN_POINT('Ctrl Pts',(-10.6541976648,-38.2742356128,1.29920325109));
#69975=CARTESIAN_POINT('Ctrl Pts',(-10.7466984979,-38.2742356128,1.31727486189));
#69976=CARTESIAN_POINT('Ctrl Pts',(-10.8391993311,-38.2372245963,1.33534647269));
#69977=CARTESIAN_POINT('Ctrl Pts',(-10.9123119707,-38.1627311721,1.34963026042));
#69978=CARTESIAN_POINT('Ctrl Pts',(-10.9486369615,-38.0684833924,1.35672697486));
#69979=CARTESIAN_POINT('Ctrl Pts',(-10.9486369615,-37.9742356128,1.35672697486));
#69980=CARTESIAN_POINT('Ctrl Pts',(-10.6809317668,-38.2742356128,1.15917604429));
#69981=CARTESIAN_POINT('Ctrl Pts',(-10.7736762576,-38.2742356128,1.17597190018));
#69982=CARTESIAN_POINT('Ctrl Pts',(-10.8664207484,-38.2372245963,1.19276775608));
#69983=CARTESIAN_POINT('Ctrl Pts',(-10.9397259711,-38.1627311721,1.20604321247));
#69984=CARTESIAN_POINT('Ctrl Pts',(-10.9761466498,-38.0684833924,1.21263891407));
#69985=CARTESIAN_POINT('Ctrl Pts',(-10.9761466498,-37.9742356128,1.21263891407));
#69986=CARTESIAN_POINT('Ctrl Pts',(-10.7044770632,-38.2742356128,1.02478825138));
#69987=CARTESIAN_POINT('Ctrl Pts',(-10.7973834123,-38.2742356128,1.0406433192));
#69988=CARTESIAN_POINT('Ctrl Pts',(-10.8902897614,-38.2372245963,1.05649838701));
#69989=CARTESIAN_POINT('Ctrl Pts',(-10.9637229232,-38.1627311721,1.06903020348));
#69990=CARTESIAN_POINT('Ctrl Pts',(-11.0002071572,-38.0684833924,1.0752564997));
#69991=CARTESIAN_POINT('Ctrl Pts',(-11.0002071572,-37.9742356128,1.0752564997));
#69992=CARTESIAN_POINT('Ctrl Pts',(-10.7213509628,-38.2742356128,0.924627136137));
#69993=CARTESIAN_POINT('Ctrl Pts',(-10.8143014058,-38.2742356128,0.940218025264));
#69994=CARTESIAN_POINT('Ctrl Pts',(-10.9072518487,-38.2372245963,0.955808914391));
#69995=CARTESIAN_POINT('Ctrl Pts',(-10.9807198422,-38.1627311721,0.968132053039));
#69996=CARTESIAN_POINT('Ctrl Pts',(-11.017221412,-38.0684833924,0.974254477573));
#69997=CARTESIAN_POINT('Ctrl Pts',(-11.017221412,-37.9742356128,0.974254477573));
#69998=CARTESIAN_POINT('Ctrl Pts',(-10.7352098055,-38.2742356128,0.840176151798));
#69999=CARTESIAN_POINT('Ctrl Pts',(-10.8282386142,-38.2742356128,0.855294575063));
#70000=CARTESIAN_POINT('Ctrl Pts',(-10.9212674229,-38.2372245963,0.870412998329));
#70001=CARTESIAN_POINT('Ctrl Pts',(-10.9947973836,-38.1627311721,0.882362527918));
#70002=CARTESIAN_POINT('Ctrl Pts',(-11.0313297006,-38.0684833924,0.888299587687));
#70003=CARTESIAN_POINT('Ctrl Pts',(-11.0313297006,-37.9742356128,0.888299587687));
#70004=CARTESIAN_POINT('Ctrl Pts',(-10.7486857355,-38.2742356128,0.75419724117));
#70005=CARTESIAN_POINT('Ctrl Pts',(-10.8417967734,-38.2742356128,0.768791027219));
#70006=CARTESIAN_POINT('Ctrl Pts',(-10.9349078112,-38.2372245963,0.783384813269));
#70007=CARTESIAN_POINT('Ctrl Pts',(-11.008502755,-38.1627311721,0.794919738554));
#70008=CARTESIAN_POINT('Ctrl Pts',(-11.0450673741,-38.0684833924,0.800650704934));
#70009=CARTESIAN_POINT('Ctrl Pts',(-11.0450673741,-37.9742356128,0.800650704934));
#70010=CARTESIAN_POINT('',(-11.0450673741,-37.9742356128,0.800650704934));
#70011=CARTESIAN_POINT('Origin',(-10.750781440652,-37.9763569039346,0.754525717032591));
#70012=CARTESIAN_POINT('Ctrl Pts',(-11.0450673741,-37.9742356128,0.800650704934));
#70013=CARTESIAN_POINT('Ctrl Pts',(-11.043029714617,-37.9742356128,0.813651347081446));
#70014=CARTESIAN_POINT('Ctrl Pts',(-11.0409811405816,-37.9742356128,0.826614446398853));
#70015=CARTESIAN_POINT('Ctrl Pts',(-11.0389082501465,-37.9742356128,0.83962956698804));
#70016=CARTESIAN_POINT('Ctrl Pts',(-11.0367226177714,-37.9742356128,0.853352563844801));
#70017=CARTESIAN_POINT('Ctrl Pts',(-11.0345100122603,-37.9742356128,0.867133053722408));
#70018=CARTESIAN_POINT('Ctrl Pts',(-11.0322638259458,-37.9742356128,0.881017973437018));
#70019=CARTESIAN_POINT('Ctrl Pts',(-11.0298438478065,-37.9742356128,0.895977196525099));
#70020=CARTESIAN_POINT('Ctrl Pts',(-11.0273849786507,-37.9742356128,0.911057150600489));
#70021=CARTESIAN_POINT('Ctrl Pts',(-11.0248881319546,-37.9742356128,0.926257079775398));
#70022=CARTESIAN_POINT('Ctrl Pts',(-11.0220231838727,-37.9742356128,0.943697881408424));
#70023=CARTESIAN_POINT('Ctrl Pts',(-11.0191083835626,-37.9742356128,0.961295875046121));
#70024=CARTESIAN_POINT('Ctrl Pts',(-11.0161550530303,-37.9742356128,0.978983247293589));
#70025=CARTESIAN_POINT('Ctrl Pts',(-11.0123390721258,-37.9742356128,1.00183699630861));
#70026=CARTESIAN_POINT('Ctrl Pts',(-11.0084595370333,-37.9742356128,1.02483590282602));
#70027=CARTESIAN_POINT('Ctrl Pts',(-11.004549929836,-37.9742356128,1.04776199688937));
#70028=CARTESIAN_POINT('Ctrl Pts',(-11.001617724438,-37.9742356128,1.06495656743688));
#70029=CARTESIAN_POINT('Ctrl Pts',(-10.9986689929647,-37.9742356128,1.08210742911664));
#70030=CARTESIAN_POINT('Ctrl Pts',(-10.9957140569788,-37.9742356128,1.09913879058753));
#70031=CARTESIAN_POINT('Ctrl Pts',(-10.993046538305,-37.9742356128,1.1145135651959));
#70032=CARTESIAN_POINT('Ctrl Pts',(-10.9903741100481,-37.9742356128,1.12978998947176));
#70033=CARTESIAN_POINT('Ctrl Pts',(-10.9876978418533,-37.9742356128,1.14494777879044));
#70034=CARTESIAN_POINT('Ctrl Pts',(-10.9851896023423,-37.9742356128,1.15915389092199));
#70035=CARTESIAN_POINT('Ctrl Pts',(-10.9826780825886,-37.9742356128,1.17325519845599));
#70036=CARTESIAN_POINT('Ctrl Pts',(-10.9801565078912,-37.9742356128,1.18727837430054));
#70037=CARTESIAN_POINT('Ctrl Pts',(-10.9781789138184,-37.9742356128,1.19827632310602));
#70038=CARTESIAN_POINT('Ctrl Pts',(-10.9761951318328,-37.9742356128,1.20922624618161));
#70039=CARTESIAN_POINT('Ctrl Pts',(-10.9741973505613,-37.9742356128,1.22016709300421));
#70040=CARTESIAN_POINT('Ctrl Pts',(-10.9724279672361,-37.9742356128,1.22985711873791));
#70041=CARTESIAN_POINT('Ctrl Pts',(-10.9706468302445,-37.9742356128,1.23954425009291));
#70042=CARTESIAN_POINT('Ctrl Pts',(-10.9688458050707,-37.9742356128,1.24927114147751));
#70043=CARTESIAN_POINT('Ctrl Pts',(-10.9658441595318,-37.9742356128,1.26548228641616));
#70044=CARTESIAN_POINT('Ctrl Pts',(-10.9627873829675,-37.9742356128,1.28180320816873));
#70045=CARTESIAN_POINT('Ctrl Pts',(-10.959680869317,-37.9742356128,1.29817179412848));
#70046=CARTESIAN_POINT('Ctrl Pts',(-10.9561464184371,-37.9742356128,1.31679523170439));
#70047=CARTESIAN_POINT('Ctrl Pts',(-10.952547477265,-37.9742356128,1.3354810217601));
#70048=CARTESIAN_POINT('Ctrl Pts',(-10.9488799948937,-37.9742356128,1.35420754643654));
#70049=CARTESIAN_POINT('Ctrl Pts',(-10.9435234773383,-37.9742356128,1.38155845041511));
#70050=CARTESIAN_POINT('Ctrl Pts',(-10.9380201984635,-37.9742356128,1.4089997435351));
#70051=CARTESIAN_POINT('Ctrl Pts',(-10.9323355373801,-37.9742356128,1.43658969318583));
#70052=CARTESIAN_POINT('Ctrl Pts',(-10.9283455568722,-37.9742356128,1.45595467549586));
#70053=CARTESIAN_POINT('Ctrl Pts',(-10.9242655286716,-37.9742356128,1.47539686828966));
#70054=CARTESIAN_POINT('Ctrl Pts',(-10.9200861694079,-37.9742356128,1.4949189254137));
#70055=CARTESIAN_POINT('Ctrl Pts',(-10.9183110532267,-37.9742356128,1.5032106077761));
#70056=CARTESIAN_POINT('Ctrl Pts',(-10.9165181002464,-37.9742356128,1.51151619372324));
#70057=CARTESIAN_POINT('Ctrl Pts',(-10.9147071085259,-37.9742356128,1.51983280126634));
#70058=CARTESIAN_POINT('Ctrl Pts',(-10.9058971470908,-37.9742356128,1.56029073980552));
#70059=CARTESIAN_POINT('Ctrl Pts',(-10.8966600534637,-37.9742356128,1.60100258738621));
#70060=CARTESIAN_POINT('Ctrl Pts',(-10.8869322989095,-37.9742356128,1.64190711298157));
#70061=CARTESIAN_POINT('Ctrl Pts',(-10.8816541363127,-37.9742356128,1.66410141649091));
#70062=CARTESIAN_POINT('Ctrl Pts',(-10.876231590757,-37.9742356128,1.68635379921446));
#70063=CARTESIAN_POINT('Ctrl Pts',(-10.8706519617309,-37.9742356128,1.70866956482949));
#70064=CARTESIAN_POINT('Ctrl Pts',(-10.8566733630686,-37.9742356128,1.76457706870001));
#70065=CARTESIAN_POINT('Ctrl Pts',(-10.8417157749528,-37.9742356128,1.82086392811176));
#70066=CARTESIAN_POINT('Ctrl Pts',(-10.8256187306821,-37.9742356128,1.87740688019527));
#70067=CARTESIAN_POINT('Ctrl Pts',(-10.8242461843505,-37.9742356128,1.88222812688856));
#70068=CARTESIAN_POINT('Ctrl Pts',(-10.8228653339238,-37.9742356128,1.88705120681551));
#70069=CARTESIAN_POINT('Ctrl Pts',(-10.8214760666396,-37.9742356128,1.89187602345432));
#70070=CARTESIAN_POINT('Ctrl Pts',(-10.8097618302743,-37.9742356128,1.93255865031043));
#70071=CARTESIAN_POINT('Ctrl Pts',(-10.7974509858169,-37.9742356128,1.9733604688576));
#70072=CARTESIAN_POINT('Ctrl Pts',(-10.7845441296016,-37.9742356128,2.01414918818009));
#70073=CARTESIAN_POINT('Ctrl Pts',(-10.7702538208126,-37.9742356128,2.0593099449518));
#70074=CARTESIAN_POINT('Ctrl Pts',(-10.7552320337685,-37.9742356128,2.10445505521447));
#70075=CARTESIAN_POINT('Ctrl Pts',(-10.7394592387859,-37.9742356128,2.14946507846607));
#70076=CARTESIAN_POINT('Ctrl Pts',(-10.7259378847107,-37.9742356128,2.18805027924931));
#70077=CARTESIAN_POINT('Ctrl Pts',(-10.7118637692977,-37.9742356128,2.22653783742124));
#70078=CARTESIAN_POINT('Ctrl Pts',(-10.6972233120527,-37.9742356128,2.26487617500612));
#70079=CARTESIAN_POINT('Ctrl Pts',(-10.6877543902685,-37.9742356128,2.28967203444221));
#70080=CARTESIAN_POINT('Ctrl Pts',(-10.6780485763058,-37.9742356128,2.31440587708767));
#70081=CARTESIAN_POINT('Ctrl Pts',(-10.6681039614208,-37.9742356128,2.33906617952837));
#70082=CARTESIAN_POINT('Ctrl Pts',(-10.6597404312459,-37.9742356128,2.35980576431583));
#70083=CARTESIAN_POINT('Ctrl Pts',(-10.6512078054758,-37.9742356128,2.3804940542434));
#70084=CARTESIAN_POINT('Ctrl Pts',(-10.6425013497725,-37.9742356128,2.40113574775587));
#70085=CARTESIAN_POINT('Ctrl Pts',(-10.6241726688637,-37.9742356128,2.44459028616991));
#70086=CARTESIAN_POINT('Ctrl Pts',(-10.605076119422,-37.9742356128,2.48782579272503));
#70087=CARTESIAN_POINT('Ctrl Pts',(-10.5852407699418,-37.9742356128,2.53076593827548));
#70088=CARTESIAN_POINT('Ctrl Pts',(-10.5671928447555,-37.9742356128,2.56983661535895));
#70089=CARTESIAN_POINT('Ctrl Pts',(-10.5485330177449,-37.9742356128,2.60866350649996));
#70090=CARTESIAN_POINT('Ctrl Pts',(-10.5293221190785,-37.9742356128,2.64716762097847));
#70091=CARTESIAN_POINT('Ctrl Pts',(-10.511707986674,-37.9742356128,2.68247136091912));
#70092=CARTESIAN_POINT('Ctrl Pts',(-10.4936305798116,-37.9742356128,2.71750404672932));
#70093=CARTESIAN_POINT('Ctrl Pts',(-10.4751726224105,-37.9742356128,2.7521792368075));
#70094=CARTESIAN_POINT('Ctrl Pts',(-10.4573434347709,-37.9742356128,2.78567321758267));
#70095=CARTESIAN_POINT('Ctrl Pts',(-10.4391590047372,-37.9742356128,2.81883397269397));
#70096=CARTESIAN_POINT('Ctrl Pts',(-10.4207304827102,-37.9742356128,2.85155406272029));
#70097=CARTESIAN_POINT('Ctrl Pts',(-10.4030434198708,-37.9742356128,2.88295768193392));
#70098=CARTESIAN_POINT('Ctrl Pts',(-10.3851314693061,-37.9742356128,2.91395554916307));
#70099=CARTESIAN_POINT('Ctrl Pts',(-10.367128661443,-37.9742356128,2.94442155879934));
#70100=CARTESIAN_POINT('Ctrl Pts',(-10.3533782097523,-37.9742356128,2.96769133965221));
#70101=CARTESIAN_POINT('Ctrl Pts',(-10.3395754397378,-37.9742356128,2.99065025975012));
#70102=CARTESIAN_POINT('Ctrl Pts',(-10.3257952819937,-37.9742356128,3.01322822752513));
#70103=CARTESIAN_POINT('Ctrl Pts',(-10.3257952821,-37.9742356128,3.01322822759));
#70104=CARTESIAN_POINT('Ctrl Pts',(-10.3257952821,-36.2942356128,3.01322822759));
#70105=CARTESIAN_POINT('Ctrl Pts',(-10.3992001828,-37.9742356128,2.89295886461));
#70106=CARTESIAN_POINT('Ctrl Pts',(-10.3992001828,-36.2942356128,2.89295886461));
#70107=CARTESIAN_POINT('Ctrl Pts',(-10.4735263391,-37.9742356128,2.76337956772));
#70108=CARTESIAN_POINT('Ctrl Pts',(-10.4735263391,-36.2942356128,2.76337956772));
#70109=CARTESIAN_POINT('Ctrl Pts',(-10.5420136,-37.9742356128,2.63031881231));
#70110=CARTESIAN_POINT('Ctrl Pts',(-10.5420136,-36.2942356128,2.63031881231));
#70111=CARTESIAN_POINT('Ctrl Pts',(-10.6667840474,-37.9742356128,2.35918484011));
#70112=CARTESIAN_POINT('Ctrl Pts',(-10.6667840474,-36.2942356128,2.35918484011));
#70113=CARTESIAN_POINT('Ctrl Pts',(-10.7670166783,-37.9742356128,2.08017125701));
#70114=CARTESIAN_POINT('Ctrl Pts',(-10.7670166783,-36.2942356128,2.08017125701));
#70115=CARTESIAN_POINT('Ctrl Pts',(-10.8111933802,-37.9742356128,1.9383801789));
#70116=CARTESIAN_POINT('Ctrl Pts',(-10.8111933802,-36.2942356128,1.9383801789));
#70117=CARTESIAN_POINT('Ctrl Pts',(-10.8740649015,-37.9742356128,1.70707199422));
#70118=CARTESIAN_POINT('Ctrl Pts',(-10.8740649015,-36.2942356128,1.70707199422));
#70119=CARTESIAN_POINT('Ctrl Pts',(-10.9239906907,-37.9742356128,1.48074082922));
#70120=CARTESIAN_POINT('Ctrl Pts',(-10.9239906907,-36.2942356128,1.48074082922));
#70121=CARTESIAN_POINT('Ctrl Pts',(-10.9420747597,-37.9742356128,1.39194060497));
#70122=CARTESIAN_POINT('Ctrl Pts',(-10.9420747597,-36.2942356128,1.39194060497));
#70123=CARTESIAN_POINT('Ctrl Pts',(-10.9747007144,-37.9742356128,1.22147170177));
#70124=CARTESIAN_POINT('Ctrl Pts',(-10.9747007144,-36.2942356128,1.22147170177));
#70125=CARTESIAN_POINT('Ctrl Pts',(-11.0034487645,-37.9742356128,1.05599081));
#70126=CARTESIAN_POINT('Ctrl Pts',(-11.0034487645,-36.2942356128,1.05599081));
#70127=CARTESIAN_POINT('Ctrl Pts',(-11.0192230843,-37.9742356128,0.962056438391));
#70128=CARTESIAN_POINT('Ctrl Pts',(-11.0192230843,-36.2942356128,0.962056438391));
#70129=CARTESIAN_POINT('Ctrl Pts',(-11.0322998283,-37.9742356128,0.882109994357));
#70130=CARTESIAN_POINT('Ctrl Pts',(-11.0322998283,-36.2942356128,0.882109994357));
#70131=CARTESIAN_POINT('Ctrl Pts',(-11.0450673741,-37.9742356128,0.800650704934));
#70132=CARTESIAN_POINT('Ctrl Pts',(-11.0450673741,-36.2942356128,0.800650704934));
#70133=CARTESIAN_POINT('',(-11.0450673741,-37.2742356128,0.800650704934));
#70134=CARTESIAN_POINT('Ctrl Pts',(-1.38699292008,-36.5742356128,-10.1328356959));
#70135=CARTESIAN_POINT('Ctrl Pts',(-1.38699292008,-36.4799878332,-10.1328356959));
#70136=CARTESIAN_POINT('Ctrl Pts',(-1.38185951829,-36.3857400536,-10.0961824078));
#70137=CARTESIAN_POINT('Ctrl Pts',(-1.37152733308,-36.3112466293,-10.0224089965));
#70138=CARTESIAN_POINT('Ctrl Pts',(-1.35845523278,-36.2742356128,-9.92907216478));
#70139=CARTESIAN_POINT('Ctrl Pts',(-1.34538313247,-36.2742356128,-9.83573533307));
#70140=CARTESIAN_POINT('Ctrl Pts',(-1.51152029043,-36.5742356128,-10.1153952681));
#70141=CARTESIAN_POINT('Ctrl Pts',(-1.51152029043,-36.4799878332,-10.1153952681));
#70142=CARTESIAN_POINT('Ctrl Pts',(-1.50631651992,-36.3857400536,-10.0787518353));
#70143=CARTESIAN_POINT('Ctrl Pts',(-1.4958427008,-36.3112466293,-10.0049982603));
#70144=CARTESIAN_POINT('Ctrl Pts',(-1.48259140782,-36.2742356128,-9.91168652503));
#70145=CARTESIAN_POINT('Ctrl Pts',(-1.46934011484,-36.2742356128,-9.81837478978));
#70146=CARTESIAN_POINT('Ctrl Pts',(-1.63096792048,-36.5742356128,-10.098359414));
#70147=CARTESIAN_POINT('Ctrl Pts',(-1.63096797981,-36.4799878326,-10.0983594061));
#70148=CARTESIAN_POINT('Ctrl Pts',(-1.62565332197,-36.3857400523,-10.061731723));
#70149=CARTESIAN_POINT('Ctrl Pts',(-1.61495624423,-36.3112466278,-9.98800985755));
#70150=CARTESIAN_POINT('Ctrl Pts',(-1.60142245201,-36.2742356118,-9.89473824575));
#70151=CARTESIAN_POINT('Ctrl Pts',(-1.58788863653,-36.2742356128,-9.80146663746));
#70152=CARTESIAN_POINT('Ctrl Pts',(-1.75323704933,-36.5742356128,-10.0804678237));
#70153=CARTESIAN_POINT('Ctrl Pts',(-1.75323702948,-36.4799878327,-10.0804678262));
#70154=CARTESIAN_POINT('Ctrl Pts',(-1.74780800354,-36.3857400526,-10.0438567886));
#70155=CARTESIAN_POINT('Ctrl Pts',(-1.73688082988,-36.3112466281,-9.97016841334));
#70156=CARTESIAN_POINT('Ctrl Pts',(-1.72305597232,-36.274235612,-9.87693916651));
#70157=CARTESIAN_POINT('Ctrl Pts',(-1.70923112261,-36.2742356128,-9.78370991904));
#70158=CARTESIAN_POINT('Ctrl Pts',(-1.98588197209,-36.5742356128,-10.0450377979));
#70159=CARTESIAN_POINT('Ctrl Pts',(-1.98588199194,-36.4799878338,-10.0450377955));
#70160=CARTESIAN_POINT('Ctrl Pts',(-1.98006948849,-36.3857400547,-10.0084834252));
#70161=CARTESIAN_POINT('Ctrl Pts',(-1.96837042637,-36.3112466306,-9.93490911225));
#70162=CARTESIAN_POINT('Ctrl Pts',(-1.95356896515,-36.2742356137,-9.84182417757));
#70163=CARTESIAN_POINT('Ctrl Pts',(-1.93876749608,-36.2742356128,-9.74873924352));
#70164=CARTESIAN_POINT('Ctrl Pts',(-2.19293659404,-36.5742356128,-10.0096459663));
#70165=CARTESIAN_POINT('Ctrl Pts',(-2.1929365742,-36.4799878327,-10.0096459687));
#70166=CARTESIAN_POINT('Ctrl Pts',(-2.18644879041,-36.3857400526,-9.97320546397));
#70167=CARTESIAN_POINT('Ctrl Pts',(-2.17339061443,-36.3112466281,-9.89986032655));
#70168=CARTESIAN_POINT('Ctrl Pts',(-2.15686965068,-36.274235612,-9.80706533814));
#70169=CARTESIAN_POINT('Ctrl Pts',(-2.14034869478,-36.2742356128,-9.7142703491));
#70170=CARTESIAN_POINT('Ctrl Pts',(-2.29885537085,-36.5742356128,-9.99032970039));
#70171=CARTESIAN_POINT('Ctrl Pts',(-2.29885536708,-36.4799878331,-9.99032970104));
#70172=CARTESIAN_POINT('Ctrl Pts',(-2.29206280416,-36.3857400534,-9.95394533749));
#70173=CARTESIAN_POINT('Ctrl Pts',(-2.27839116924,-36.3112466291,-9.88071319968));
#70174=CARTESIAN_POINT('Ctrl Pts',(-2.26109405783,-36.2742356127,-9.78806117733));
#70175=CARTESIAN_POINT('Ctrl Pts',(-2.24379694792,-36.2742356128,-9.69540915479));
#70176=CARTESIAN_POINT('Ctrl Pts',(-2.69693922631,-36.5742356128,-9.91335054502));
#70177=CARTESIAN_POINT('Ctrl Pts',(-2.69693923691,-36.4799878335,-9.91335054317));
#70178=CARTESIAN_POINT('Ctrl Pts',(-2.6889563496,-36.3857400542,-9.87719590648));
#70179=CARTESIAN_POINT('Ctrl Pts',(-2.67288888841,-36.31124663,-9.80442615135));
#70180=CARTESIAN_POINT('Ctrl Pts',(-2.65256061041,-36.2742356133,-9.71235912888));
#70181=CARTESIAN_POINT('Ctrl Pts',(-2.6322323282,-36.2742356128,-9.62029210697));
#70182=CARTESIAN_POINT('Ctrl Pts',(-3.0919938661,-36.5742356128,-9.81991318886));
#70183=CARTESIAN_POINT('Ctrl Pts',(-3.09199383639,-36.4799878324,-9.81991319404));
#70184=CARTESIAN_POINT('Ctrl Pts',(-3.08278784534,-36.385740052,-9.78404777523));
#70185=CARTESIAN_POINT('Ctrl Pts',(-3.0642586456,-36.3112466275,-9.71186013107));
#70186=CARTESIAN_POINT('Ctrl Pts',(-3.04081584451,-36.2742356116,-9.62052958129));
#70187=CARTESIAN_POINT('Ctrl Pts',(-3.01737305521,-36.2742356128,-9.52919902996));
#70188=CARTESIAN_POINT('Ctrl Pts',(-3.38040989704,-36.5742356128,-9.7419516802));
#70189=CARTESIAN_POINT('Ctrl Pts',(-3.38040989405,-36.4799878327,-9.74195168123));
#70190=CARTESIAN_POINT('Ctrl Pts',(-3.37029179636,-36.3857400526,-9.70633130336));
#70191=CARTESIAN_POINT('Ctrl Pts',(-3.34992673534,-36.3112466282,-9.634636867));
#70192=CARTESIAN_POINT('Ctrl Pts',(-3.32416121766,-36.274235612,-9.54393031759));
#70193=CARTESIAN_POINT('Ctrl Pts',(-3.29839570127,-36.2742356128,-9.45322376807));
#70194=CARTESIAN_POINT('Ctrl Pts',(-3.87968490278,-36.5742356128,-9.58959720128));
#70195=CARTESIAN_POINT('Ctrl Pts',(-3.87968490502,-36.4799878336,-9.58959720052));
#70196=CARTESIAN_POINT('Ctrl Pts',(-3.86796253504,-36.3857400544,-9.55446591569));
#70197=CARTESIAN_POINT('Ctrl Pts',(-3.84436849025,-36.3112466302,-9.48375589692));
#70198=CARTESIAN_POINT('Ctrl Pts',(-3.81451771536,-36.2742356134,-9.39429481622));
#70199=CARTESIAN_POINT('Ctrl Pts',(-3.78466693948,-36.2742356128,-9.30483373562));
#70200=CARTESIAN_POINT('Ctrl Pts',(-4.36855122677,-36.5742356128,-9.40939629264));
#70201=CARTESIAN_POINT('Ctrl Pts',(-4.36855122509,-36.4799878329,-9.40939629322));
#70202=CARTESIAN_POINT('Ctrl Pts',(-4.35523621791,-36.3857400531,-9.37485180944));
#70203=CARTESIAN_POINT('Ctrl Pts',(-4.32843661881,-36.3112466287,-9.30532286492));
#70204=CARTESIAN_POINT('Ctrl Pts',(-4.29453023508,-36.2742356124,-9.21735605819));
#70205=CARTESIAN_POINT('Ctrl Pts',(-4.26062385208,-36.2742356128,-9.12938925139));
#70206=CARTESIAN_POINT('Ctrl Pts',(-4.5760187763,-36.5742356128,-9.32706183536));
#70207=CARTESIAN_POINT('Ctrl Pts',(-4.5760187745,-36.4799878338,-9.3270618362));
#70208=CARTESIAN_POINT('Ctrl Pts',(-4.56202665041,-36.3857400547,-9.29278602584));
#70209=CARTESIAN_POINT('Ctrl Pts',(-4.53386419357,-36.3112466306,-9.22379784981));
#70210=CARTESIAN_POINT('Ctrl Pts',(-4.49823354595,-36.2742356137,-9.13651521345));
#70211=CARTESIAN_POINT('Ctrl Pts',(-4.46260289891,-36.2742356128,-9.04923257645));
#70212=CARTESIAN_POINT('Ctrl Pts',(-5.19275926061,-36.5742356128,-9.06462215196));
#70213=CARTESIAN_POINT('Ctrl Pts',(-5.19275926422,-36.4799878322,-9.06462215026));
#70214=CARTESIAN_POINT('Ctrl Pts',(-5.17675952444,-36.3857400515,-9.03120113486));
#70215=CARTESIAN_POINT('Ctrl Pts',(-5.14455625961,-36.3112466268,-8.96393343893));
#70216=CARTESIAN_POINT('Ctrl Pts',(-5.10381324925,-36.2742356112,-8.87882752609));
#70217=CARTESIAN_POINT('Ctrl Pts',(-5.06307023773,-36.2742356128,-8.79372161452));
#70218=CARTESIAN_POINT('Ctrl Pts',(-5.78834049125,-36.5742356128,-8.75798298595));
#70219=CARTESIAN_POINT('Ctrl Pts',(-5.788340484,-36.4799878354,-8.75798298935));
#70220=CARTESIAN_POINT('Ctrl Pts',(-5.77044437661,-36.3857400579,-8.72553988322));
#70221=CARTESIAN_POINT('Ctrl Pts',(-5.73442423661,-36.3112466344,-8.66024045486));
#70222=CARTESIAN_POINT('Ctrl Pts',(-5.68885218855,-36.2742356162,-8.57762475546));
#70223=CARTESIAN_POINT('Ctrl Pts',(-5.64328014279,-36.2742356128,-8.49500905351));
#70224=CARTESIAN_POINT('Ctrl Pts',(-6.17544881684,-36.5742356128,-8.53471177464));
#70225=CARTESIAN_POINT('Ctrl Pts',(-6.1754488205,-36.4799878347,-8.53471177187));
#70226=CARTESIAN_POINT('Ctrl Pts',(-6.15635088894,-36.3857400565,-8.5029666931));
#70227=CARTESIAN_POINT('Ctrl Pts',(-6.11791178011,-36.3112466328,-8.43907221751));
#70228=CARTESIAN_POINT('Ctrl Pts',(-6.06927928827,-36.2742356151,-8.35823404393));
#70229=CARTESIAN_POINT('Ctrl Pts',(-6.02064679434,-36.2742356128,-8.27739587081));
#70230=CARTESIAN_POINT('Ctrl Pts',(-6.92915280215,-36.5742356128,-8.05308379561));
#70231=CARTESIAN_POINT('Ctrl Pts',(-6.92915279847,-36.4799878318,-8.05308379839));
#70232=CARTESIAN_POINT('Ctrl Pts',(-6.90785214448,-36.3857400507,-8.02275557517));
#70233=CARTESIAN_POINT('Ctrl Pts',(-6.86497954496,-36.3112466259,-7.96171284949));
#70234=CARTESIAN_POINT('Ctrl Pts',(-6.81073788334,-36.2742356106,-7.88448265761));
#70235=CARTESIAN_POINT('Ctrl Pts',(-6.75649622382,-36.2742356128,-7.80725246527));
#70236=CARTESIAN_POINT('Ctrl Pts',(-7.64600571687,-36.5742356128,-7.5075764295));
#70237=CARTESIAN_POINT('Ctrl Pts',(-7.64600572057,-36.4799878347,-7.50757642669));
#70238=CARTESIAN_POINT('Ctrl Pts',(-7.62292488665,-36.3857400566,-7.47861327484));
#70239=CARTESIAN_POINT('Ctrl Pts',(-7.57646924515,-36.3112466328,-7.42031808495));
#70240=CARTESIAN_POINT('Ctrl Pts',(-7.51769437599,-36.2742356151,-7.34656402996));
#70241=CARTESIAN_POINT('Ctrl Pts',(-7.45891950471,-36.2742356128,-7.27280997543));
#70242=CARTESIAN_POINT('Ctrl Pts',(-7.99980083252,-36.5742356128,-7.21703589238));
#70243=CARTESIAN_POINT('Ctrl Pts',(-7.99980082858,-36.4799878295,-7.21703589554));
#70244=CARTESIAN_POINT('Ctrl Pts',(-7.97586366783,-36.3857400462,-7.18878251664));
#70245=CARTESIAN_POINT('Ctrl Pts',(-7.92768447517,-36.3112466206,-7.13191590546));
#70246=CARTESIAN_POINT('Ctrl Pts',(-7.86672900529,-36.274235607,-7.05996926121));
#70247=CARTESIAN_POINT('Ctrl Pts',(-7.80577353846,-36.2742356128,-6.9880226175));
#70248=CARTESIAN_POINT('Ctrl Pts',(-8.84905353168,-36.5742356128,-6.46450747752));
#70249=CARTESIAN_POINT('Ctrl Pts',(-8.84905353743,-36.4799878387,-6.46450747292));
#70250=CARTESIAN_POINT('Ctrl Pts',(-8.82295393196,-36.3857400645,-6.43813308402));
#70251=CARTESIAN_POINT('Ctrl Pts',(-8.77042229601,-36.3112466421,-6.38504839428));
#70252=CARTESIAN_POINT('Ctrl Pts',(-8.70396018261,-36.2742356214,-6.31788657283));
#70253=CARTESIAN_POINT('Ctrl Pts',(-8.63749806478,-36.2742356128,-6.25072475062));
#70254=CARTESIAN_POINT('Ctrl Pts',(-9.61892143257,-36.5742356128,-5.61595506741));
#70255=CARTESIAN_POINT('Ctrl Pts',(-9.61892142418,-36.4799878253,-5.61595507411));
#70256=CARTESIAN_POINT('Ctrl Pts',(-9.59030674766,-36.3857400378,-5.59233308488));
#70257=CARTESIAN_POINT('Ctrl Pts',(-9.53271295384,-36.3112466107,-5.544788236));
#70258=CARTESIAN_POINT('Ctrl Pts',(-9.45984629869,-36.2742356004,-5.48463532196));
#70259=CARTESIAN_POINT('Ctrl Pts',(-9.38697965001,-36.2742356128,-5.42448240903));
#70260=CARTESIAN_POINT('Ctrl Pts',(-10.0435276565,-36.5742356128,-5.07402143134));
#70261=CARTESIAN_POINT('Ctrl Pts',(-10.0435276316,-36.4799878177,-5.07402148559));
#70262=CARTESIAN_POINT('Ctrl Pts',(-10.0130849077,-36.3857400225,-5.05250152625));
#70263=CARTESIAN_POINT('Ctrl Pts',(-9.95181175627,-36.3112465927,-5.00918745144));
#70264=CARTESIAN_POINT('Ctrl Pts',(-9.87429005612,-36.2742355884,-4.95438720865));
#70265=CARTESIAN_POINT('Ctrl Pts',(-9.79676837504,-36.2742356128,-4.89958694614));
#70266=CARTESIAN_POINT('Ctrl Pts',(-10.6579518564,-36.5742356128,-4.04641144733));
#70267=CARTESIAN_POINT('Ctrl Pts',(-10.6579518746,-36.4799878446,-4.04641140784));
#70268=CARTESIAN_POINT('Ctrl Pts',(-10.6240592807,-36.3857400763,-4.03054004281));
#70269=CARTESIAN_POINT('Ctrl Pts',(-10.5558423977,-36.311246656,-3.99859521531));
#70270=CARTESIAN_POINT('Ctrl Pts',(-10.469535573,-36.2742356306,-3.95817920057));
#70271=CARTESIAN_POINT('Ctrl Pts',(-10.3832287344,-36.2742356128,-3.91776320018));
#70272=CARTESIAN_POINT('Ctrl Pts',(-11.0188703723,-36.5742356128,-2.91552801853));
#70273=CARTESIAN_POINT('Ctrl Pts',(-11.0188703591,-36.479987825,-2.91552804728));
#70274=CARTESIAN_POINT('Ctrl Pts',(-10.9828310738,-36.3857400371,-2.90637408447));
#70275=CARTESIAN_POINT('Ctrl Pts',(-10.9102935043,-36.3112466099,-2.88794953427));
#70276=CARTESIAN_POINT('Ctrl Pts',(-10.8185202492,-36.2742355999,-2.86463909812));
#70277=CARTESIAN_POINT('Ctrl Pts',(-10.7267470043,-36.2742356128,-2.84132865151));
#70278=CARTESIAN_POINT('Ctrl Pts',(-11.1211124249,-36.5742356128,-2.42831608424));
#70279=CARTESIAN_POINT('Ctrl Pts',(-11.1211124689,-36.4799878553,-2.42831638526));
#70280=CARTESIAN_POINT('Ctrl Pts',(-11.0844967792,-36.3857400977,-2.42201094849));
#70281=CARTESIAN_POINT('Ctrl Pts',(-11.010798996,-36.3112466813,-2.40931943624));
#70282=CARTESIAN_POINT('Ctrl Pts',(-10.9175578094,-36.2742356474,-2.39326215592));
#70283=CARTESIAN_POINT('Ctrl Pts',(-10.8243165921,-36.2742356128,-2.37720475576));
#70284=CARTESIAN_POINT('Ctrl Pts',(-11.2315884468,-36.5742356128,-1.47511926274));
#70285=CARTESIAN_POINT('Ctrl Pts',(-11.2315884056,-36.4799878126,-1.47511898088));
#70286=CARTESIAN_POINT('Ctrl Pts',(-11.1944459333,-36.3857400124,-1.47378416589));
#70287=CARTESIAN_POINT('Ctrl Pts',(-11.1196879677,-36.3112465807,-1.47109784338));
#70288=CARTESIAN_POINT('Ctrl Pts',(-11.0251055307,-36.2742355804,-1.46769934297));
#70289=CARTESIAN_POINT('Ctrl Pts',(-10.9305231225,-36.2742356128,-1.46430095477));
#70290=CARTESIAN_POINT('Ctrl Pts',(-11.2043755329,-36.5742356128,-0.530546116159));
#70291=CARTESIAN_POINT('Ctrl Pts',(-11.2043755715,-36.4799878525,-0.53054638008));
#70292=CARTESIAN_POINT('Ctrl Pts',(-11.1673834471,-36.3857400923,-0.532820991327));
#70293=CARTESIAN_POINT('Ctrl Pts',(-11.0929280062,-36.3112466749,-0.537398895803));
#70294=CARTESIAN_POINT('Ctrl Pts',(-10.9987282489,-36.2742356432,-0.54319060461));
#70295=CARTESIAN_POINT('Ctrl Pts',(-10.9045284647,-36.2742356128,-0.548982208346));
#70296=CARTESIAN_POINT('Ctrl Pts',(-11.1665128558,-36.5742356128,-0.077344330525));
#70297=CARTESIAN_POINT('Ctrl Pts',(-11.1665126991,-36.4799878387,-0.0773433425996));
#70298=CARTESIAN_POINT('Ctrl Pts',(-11.1296536904,-36.3857400646,-0.0809244862498));
#70299=CARTESIAN_POINT('Ctrl Pts',(-11.055466388,-36.3112466423,-0.0881334573585));
#70300=CARTESIAN_POINT('Ctrl Pts',(-10.9616060106,-36.2742356215,-0.0972547802524));
#70301=CARTESIAN_POINT('Ctrl Pts',(-10.8677456912,-36.2742356128,-0.106376490674));
#70302=CARTESIAN_POINT('Ctrl Pts',(-11.1136931672,-36.5742356128,0.362811362875));
#70303=CARTESIAN_POINT('Ctrl Pts',(-11.113693272,-36.4799878329,0.362810700302));
#70304=CARTESIAN_POINT('Ctrl Pts',(-11.0769608227,-36.385740053,0.358150436098));
#70305=CARTESIAN_POINT('Ctrl Pts',(-11.0030279669,-36.3112466286,0.348771272008));
#70306=CARTESIAN_POINT('Ctrl Pts',(-10.9094893391,-36.2742356123,0.336905358648));
#70307=CARTESIAN_POINT('Ctrl Pts',(-10.8159506704,-36.2742356128,0.325039704942));
#70308=CARTESIAN_POINT('Ctrl Pts',(-11.0450672445,-36.5742356128,0.800651515617));
#70309=CARTESIAN_POINT('Ctrl Pts',(-11.045067244,-36.4799878332,0.800651518699));
#70310=CARTESIAN_POINT('Ctrl Pts',(-11.0085026394,-36.3857400536,0.794920460492));
#70311=CARTESIAN_POINT('Ctrl Pts',(-10.9349077252,-36.3112466293,0.783385346618));
#70312=CARTESIAN_POINT('Ctrl Pts',(-10.8417967252,-36.2742356128,0.768791320097));
#70313=CARTESIAN_POINT('Ctrl Pts',(-10.7486857254,-36.2742356128,0.754197292365));
#70314=CARTESIAN_POINT('',(-1.38699292015031,-36.5742356128,-10.1328356964021));
#70315=CARTESIAN_POINT('Origin',(-1.34567758431402,-36.5721143209619,-9.8378360912598));
#70316=CARTESIAN_POINT('Ctrl Pts',(-1.38699292008,-36.5742356128,-10.1328356959));
#70317=CARTESIAN_POINT('Ctrl Pts',(-1.54048434157,-36.5742356128,-10.1113387667));
#70318=CARTESIAN_POINT('Ctrl Pts',(-1.68405004862,-36.5742356128,-10.0907690318));
#70319=CARTESIAN_POINT('Ctrl Pts',(-1.83768542132,-36.5742356128,-10.0680136807));
#70320=CARTESIAN_POINT('Ctrl Pts',(-2.0472685103,-36.5742356128,-10.0350233698));
#70321=CARTESIAN_POINT('Ctrl Pts',(-2.24744160945,-36.5742356128,-9.99950190736));
#70322=CARTESIAN_POINT('Ctrl Pts',(-2.32512404463,-36.5742356128,-9.9850708371));
#70323=CARTESIAN_POINT('Ctrl Pts',(-2.47861794583,-36.5742356128,-9.95531796778));
#70324=CARTESIAN_POINT('Ctrl Pts',(-2.63158870593,-36.5742356128,-9.9231347794));
#70325=CARTESIAN_POINT('Ctrl Pts',(-2.70802102444,-36.5742356128,-9.90641220658));
#70326=CARTESIAN_POINT('Ctrl Pts',(-3.01253146542,-36.5742356128,-9.83720045464));
#70327=CARTESIAN_POINT('Ctrl Pts',(-3.31446912355,-36.5742356128,-9.75814914822));
#70328=CARTESIAN_POINT('Ctrl Pts',(-3.53901439175,-36.5742356128,-9.69332241166));
#70329=CARTESIAN_POINT('Ctrl Pts',(-4.06616678433,-36.5742356128,-9.5265559109));
#70330=CARTESIAN_POINT('Ctrl Pts',(-4.58136980211,-36.5742356128,-9.32859973654));
#70331=CARTESIAN_POINT('Ctrl Pts',(-4.87486658275,-36.5742356128,-9.20377818652));
#70332=CARTESIAN_POINT('Ctrl Pts',(-5.45178039505,-36.5742356128,-8.9342344636));
#70333=CARTESIAN_POINT('Ctrl Pts',(-6.0085344695,-36.5742356128,-8.62630121912));
#70334=CARTESIAN_POINT('Ctrl Pts',(-6.28153293631,-36.5742356128,-8.46325996649));
#70335=CARTESIAN_POINT('Ctrl Pts',(-6.68293897529,-36.5742356128,-8.20578167081));
#70336=CARTESIAN_POINT('Ctrl Pts',(-7.07391925375,-36.5742356128,-7.9296599837));
#70337=CARTESIAN_POINT('Ctrl Pts',(-7.20312714751,-36.5742356128,-7.83561707231));
#70338=CARTESIAN_POINT('Ctrl Pts',(-7.71835943346,-36.5742356128,-7.44951290203));
#70339=CARTESIAN_POINT('Ctrl Pts',(-8.21985964705,-36.5742356128,-7.02884209138));
#70340=CARTESIAN_POINT('Ctrl Pts',(-8.58741395083,-36.5742356128,-6.694450027));
#70341=CARTESIAN_POINT('Ctrl Pts',(-9.23922565915,-36.5742356128,-6.04471661443));
#70342=CARTESIAN_POINT('Ctrl Pts',(-9.82149842759,-36.5742356128,-5.3259548207));
#70343=CARTESIAN_POINT('Ctrl Pts',(-10.0721843915,-36.5742356128,-4.97806710989));
#70344=CARTESIAN_POINT('Ctrl Pts',(-10.6524574839,-36.5742356128,-4.03375119461));
#70345=CARTESIAN_POINT('Ctrl Pts',(-11.0291793988,-36.5742356128,-2.98459593108));
#70346=CARTESIAN_POINT('Ctrl Pts',(-11.1622899814,-36.5742356128,-2.31636115633));
#70347=CARTESIAN_POINT('Ctrl Pts',(-11.2336540706,-36.5742356128,-1.36618233642));
#70348=CARTESIAN_POINT('Ctrl Pts',(-11.1889875368,-36.5742356128,-0.434883867537));
#70349=CARTESIAN_POINT('Ctrl Pts',(-11.1677658434,-36.5742356128,-0.163547364276));
#70350=CARTESIAN_POINT('Ctrl Pts',(-11.1309935407,-36.5742356128,0.191196052966));
#70351=CARTESIAN_POINT('Ctrl Pts',(-11.0837537732,-36.5742356128,0.541839826065));
#70352=CARTESIAN_POINT('Ctrl Pts',(-11.0714556362,-36.5742356128,0.62831585634));
#70353=CARTESIAN_POINT('Ctrl Pts',(-11.0585597994,-36.5742356128,0.714566551426));
#70354=CARTESIAN_POINT('Ctrl Pts',(-11.0450673741,-36.5742356128,0.800650704934));
#70355=CARTESIAN_POINT('Ctrl Pts',(-10.7486857339,-38.2742356128,0.754197251045));
#70356=CARTESIAN_POINT('Ctrl Pts',(-10.8417967716,-38.2742356128,0.768791038108));
#70357=CARTESIAN_POINT('Ctrl Pts',(-10.9349078093,-38.2372245963,0.783384825171));
#70358=CARTESIAN_POINT('Ctrl Pts',(-11.008502753,-38.1627311721,0.794919751257));
#70359=CARTESIAN_POINT('Ctrl Pts',(-11.045067372,-38.0684833924,0.800650718035));
#70360=CARTESIAN_POINT('Ctrl Pts',(-11.045067372,-37.9742356128,0.800650718035));
#70361=CARTESIAN_POINT('Ctrl Pts',(-10.8644820124,-38.2742356128,0.015396349477));
#70362=CARTESIAN_POINT('Ctrl Pts',(-10.95831508,-38.2742356128,0.0253834674463));
#70363=CARTESIAN_POINT('Ctrl Pts',(-11.0521481476,-38.2372245963,0.0353705854157));
#70364=CARTESIAN_POINT('Ctrl Pts',(-11.1263136449,-38.1627311721,0.0432652827677));
#70365=CARTESIAN_POINT('Ctrl Pts',(-11.1631619431,-38.0684833924,0.0471863333183));
#70366=CARTESIAN_POINT('Ctrl Pts',(-11.1631619431,-37.9742356128,0.0471863333183));
#70367=CARTESIAN_POINT('Ctrl Pts',(-10.9353869016,-38.2742356128,-0.736346737241));
#70368=CARTESIAN_POINT('Ctrl Pts',(-11.0296310539,-38.2742356128,-0.731109451787));
#70369=CARTESIAN_POINT('Ctrl Pts',(-11.1238752062,-38.2372245963,-0.725872166333));
#70370=CARTESIAN_POINT('Ctrl Pts',(-11.1983659715,-38.1627311721,-0.721733939256));
#70371=CARTESIAN_POINT('Ctrl Pts',(-11.2353753555,-38.0684833924,-0.719675939874));
#70372=CARTESIAN_POINT('Ctrl Pts',(-11.2353753555,-37.9742356128,-0.719675939874));
#70373=CARTESIAN_POINT('Ctrl Pts',(-10.9581033367,-38.2742356128,-1.51216421625));
#70374=CARTESIAN_POINT('Ctrl Pts',(-11.0532569791,-38.2742356128,-1.51543079532));
#70375=CARTESIAN_POINT('Ctrl Pts',(-11.1484106216,-38.2372245963,-1.51869737439));
#70376=CARTESIAN_POINT('Ctrl Pts',(-11.2236199878,-38.1627311721,-1.52127894667));
#70377=CARTESIAN_POINT('Ctrl Pts',(-11.2609867877,-38.0684833924,-1.52256206037));
#70378=CARTESIAN_POINT('Ctrl Pts',(-11.2609867877,-37.9742356128,-1.52256206037));
#70379=CARTESIAN_POINT('Ctrl Pts',(-10.831079727,-38.2742356128,-2.52840849741));
#70380=CARTESIAN_POINT('Ctrl Pts',(-10.9245012349,-38.2742356128,-2.54681170763));
#70381=CARTESIAN_POINT('Ctrl Pts',(-11.0179227428,-38.2372245963,-2.56521491785));
#70382=CARTESIAN_POINT('Ctrl Pts',(-11.0917630994,-38.1627311721,-2.57976092087));
#70383=CARTESIAN_POINT('Ctrl Pts',(-11.1284496225,-38.0684833924,-2.58698773492));
#70384=CARTESIAN_POINT('Ctrl Pts',(-11.1284496225,-37.9742356128,-2.58698773492));
#70385=CARTESIAN_POINT('Ctrl Pts',(-10.4997203395,-38.2742356128,-3.49265676226));
#70386=CARTESIAN_POINT('Ctrl Pts',(-10.5879306786,-38.2742356128,-3.52619793269));
#70387=CARTESIAN_POINT('Ctrl Pts',(-10.6761410178,-38.2372245963,-3.55973910313));
#70388=CARTESIAN_POINT('Ctrl Pts',(-10.7458624447,-38.1627311721,-3.58625000051));
#70389=CARTESIAN_POINT('Ctrl Pts',(-10.7805025696,-38.0684833924,-3.59942162369));
#70390=CARTESIAN_POINT('Ctrl Pts',(-10.7805025696,-37.9742356128,-3.59942162369));
#70391=CARTESIAN_POINT('Ctrl Pts',(-10.4039697378,-38.2742356128,-3.72874327308));
#70392=CARTESIAN_POINT('Ctrl Pts',(-10.4906791962,-38.2742356128,-3.76598554153));
#70393=CARTESIAN_POINT('Ctrl Pts',(-10.5773886547,-38.2372245963,-3.80322780998));
#70394=CARTESIAN_POINT('Ctrl Pts',(-10.6459237916,-38.1627311721,-3.83266409077));
#70395=CARTESIAN_POINT('Ctrl Pts',(-10.6799745163,-38.0684833924,-3.8472890954));
#70396=CARTESIAN_POINT('Ctrl Pts',(-10.6799745163,-37.9742356128,-3.8472890954));
#70397=CARTESIAN_POINT('Ctrl Pts',(-10.0688223315,-38.2742356128,-4.4465666977));
#70398=CARTESIAN_POINT('Ctrl Pts',(-10.1503858218,-38.2742356128,-4.49478078091));
#70399=CARTESIAN_POINT('Ctrl Pts',(-10.231949312,-38.2372245963,-4.54299486411));
#70400=CARTESIAN_POINT('Ctrl Pts',(-10.2964170767,-38.1627311721,-4.58110326484));
#70401=CARTESIAN_POINT('Ctrl Pts',(-10.3284469844,-38.0684833924,-4.60003689108));
#70402=CARTESIAN_POINT('Ctrl Pts',(-10.3284469844,-37.9742356128,-4.60003689108));
#70403=CARTESIAN_POINT('Ctrl Pts',(-9.62301691076,-38.2742356128,-5.11189798418));
#70404=CARTESIAN_POINT('Ctrl Pts',(-9.69858882439,-38.2742356128,-5.16881938559));
#70405=CARTESIAN_POINT('Ctrl Pts',(-9.77416073802,-38.2372245963,-5.22574078701));
#70406=CARTESIAN_POINT('Ctrl Pts',(-9.83389276175,-38.1627311721,-5.27073145039));
#70407=CARTESIAN_POINT('Ctrl Pts',(-9.86356978302,-38.0684833924,-5.29308443223));
#70408=CARTESIAN_POINT('Ctrl Pts',(-9.86356978302,-37.9742356128,-5.29308443223));
#70409=CARTESIAN_POINT('Ctrl Pts',(-9.28042553493,-38.2742356128,-5.53648144054));
#70410=CARTESIAN_POINT('Ctrl Pts',(-9.35246734892,-38.2742356128,-5.59750992502));
#70411=CARTESIAN_POINT('Ctrl Pts',(-9.42450916291,-38.2372245963,-5.65853840949));
#70412=CARTESIAN_POINT('Ctrl Pts',(-9.4814509968,-38.1627311721,-5.70677531028));
#70413=CARTESIAN_POINT('Ctrl Pts',(-9.50974175105,-38.0684833924,-5.73074114001));
#70414=CARTESIAN_POINT('Ctrl Pts',(-9.50974175105,-37.9742356128,-5.73074114001));
#70415=CARTESIAN_POINT('Ctrl Pts',(-8.60018141119,-38.2742356128,-6.27983264313));
#70416=CARTESIAN_POINT('Ctrl Pts',(-8.66640539804,-38.2742356128,-6.34716877797));
#70417=CARTESIAN_POINT('Ctrl Pts',(-8.73262938489,-38.2372245963,-6.4145049128));
#70418=CARTESIAN_POINT('Ctrl Pts',(-8.78497280955,-38.1627311721,-6.46772737895));
#70419=CARTESIAN_POINT('Ctrl Pts',(-8.81097890835,-38.0684833924,-6.49417021728));
#70420=CARTESIAN_POINT('Ctrl Pts',(-8.81097890835,-37.9742356128,-6.49417021728));
#70421=CARTESIAN_POINT('Ctrl Pts',(-7.85121695461,-38.2742356128,-6.95010363271));
#70422=CARTESIAN_POINT('Ctrl Pts',(-7.91247104152,-38.2742356128,-7.02180601188));
#70423=CARTESIAN_POINT('Ctrl Pts',(-7.97372512843,-38.2372245963,-7.09350839104));
#70424=CARTESIAN_POINT('Ctrl Pts',(-8.02214034526,-38.1627311721,-7.15018193575));
#70425=CARTESIAN_POINT('Ctrl Pts',(-8.04619476894,-38.0684833924,-7.17833939422));
#70426=CARTESIAN_POINT('Ctrl Pts',(-8.04619476894,-37.9742356128,-7.17833939422));
#70427=CARTESIAN_POINT('Ctrl Pts',(-7.49651322649,-38.2742356128,-7.24338281986));
#70428=CARTESIAN_POINT('Ctrl Pts',(-7.55552872191,-38.2742356128,-7.3169478207));
#70429=CARTESIAN_POINT('Ctrl Pts',(-7.61454421733,-38.2372245963,-7.39051282155));
#70430=CARTESIAN_POINT('Ctrl Pts',(-7.66119005191,-38.1627311721,-7.44865858205));
#70431=CARTESIAN_POINT('Ctrl Pts',(-7.68436538279,-38.0684833924,-7.47754749032));
#70432=CARTESIAN_POINT('Ctrl Pts',(-7.68436538279,-37.9742356128,-7.47754749032));
#70433=CARTESIAN_POINT('Ctrl Pts',(-6.78245213327,-38.2742356128,-7.7898018263));
#70434=CARTESIAN_POINT('Ctrl Pts',(-6.83688001526,-38.2742356128,-7.86690543711));
#70435=CARTESIAN_POINT('Ctrl Pts',(-6.89130789724,-38.2372245963,-7.94400904792));
#70436=CARTESIAN_POINT('Ctrl Pts',(-6.93432768319,-38.1627311721,-8.00495172497));
#70437=CARTESIAN_POINT('Ctrl Pts',(-6.95570146247,-38.0684833924,-8.03523024212));
#70438=CARTESIAN_POINT('Ctrl Pts',(-6.95570146247,-37.9742356128,-8.03523024212));
#70439=CARTESIAN_POINT('Ctrl Pts',(-6.03422296673,-38.2742356128,-8.26953898084));
#70440=CARTESIAN_POINT('Ctrl Pts',(-6.08296773524,-38.2742356128,-8.35031143298));
#70441=CARTESIAN_POINT('Ctrl Pts',(-6.13171250375,-38.2372245963,-8.43108388512));
#70442=CARTESIAN_POINT('Ctrl Pts',(-6.1702403581,-38.1627311721,-8.49492641351));
#70443=CARTESIAN_POINT('Ctrl Pts',(-6.1893823839,-38.0684833924,-8.52664568131));
#70444=CARTESIAN_POINT('Ctrl Pts',(-6.1893823839,-37.9742356128,-8.52664568131));
#70445=CARTESIAN_POINT('Ctrl Pts',(-5.65254018915,-38.2742356128,-8.4902387588));
#70446=CARTESIAN_POINT('Ctrl Pts',(-5.69818840924,-38.2742356128,-8.57281530405));
#70447=CARTESIAN_POINT('Ctrl Pts',(-5.74383662934,-38.2372245963,-8.65539184929));
#70448=CARTESIAN_POINT('Ctrl Pts',(-5.77991697251,-38.1627311721,-8.72066033248));
#70449=CARTESIAN_POINT('Ctrl Pts',(-5.79784298659,-38.0684833924,-8.75308806599));
#70450=CARTESIAN_POINT('Ctrl Pts',(-5.79784298659,-37.9742356128,-8.75308806599));
#70451=CARTESIAN_POINT('Ctrl Pts',(-5.06785956151,-38.2742356128,-8.79168353687));
#70452=CARTESIAN_POINT('Ctrl Pts',(-5.10864378738,-38.2742356128,-8.87677178634));
#70453=CARTESIAN_POINT('Ctrl Pts',(-5.14942801325,-38.2372245963,-8.96186003582));
#70454=CARTESIAN_POINT('Ctrl Pts',(-5.1816638564,-38.1627311721,-9.0291137695));
#70455=CARTESIAN_POINT('Ctrl Pts',(-5.19767978446,-38.0684833924,-9.06252784693));
#70456=CARTESIAN_POINT('Ctrl Pts',(-5.19767978446,-37.9742356128,-9.06252784693));
#70457=CARTESIAN_POINT('Ctrl Pts',(-4.46260362429,-38.2742356128,-9.04923232877));
#70458=CARTESIAN_POINT('Ctrl Pts',(-4.49823406166,-38.2742356128,-9.1365151112));
#70459=CARTESIAN_POINT('Ctrl Pts',(-4.53386449903,-38.2372245963,-9.22379789362));
#70460=CARTESIAN_POINT('Ctrl Pts',(-4.56202678889,-38.1627311721,-9.29278618567));
#70461=CARTESIAN_POINT('Ctrl Pts',(-4.57601882892,-38.0684833924,-9.32706205417));
#70462=CARTESIAN_POINT('Ctrl Pts',(-4.57601882892,-37.9742356128,-9.32706205417));
#70463=CARTESIAN_POINT('Ctrl Pts',(-4.26062386225,-38.2742356128,-9.12938925058));
#70464=CARTESIAN_POINT('Ctrl Pts',(-4.29453024428,-38.2742356128,-9.21735605705));
#70465=CARTESIAN_POINT('Ctrl Pts',(-4.3284366263,-38.2372245963,-9.30532286352));
#70466=CARTESIAN_POINT('Ctrl Pts',(-4.3552362232,-38.1627311721,-9.37485180801));
#70467=CARTESIAN_POINT('Ctrl Pts',(-4.36855122828,-38.0684833924,-9.40939629213));
#70468=CARTESIAN_POINT('Ctrl Pts',(-4.36855122828,-37.9742356128,-9.40939629213));
#70469=CARTESIAN_POINT('Ctrl Pts',(-3.7846669259,-38.2742356128,-9.30483373669));
#70470=CARTESIAN_POINT('Ctrl Pts',(-3.81451770308,-38.2742356128,-9.39429481774));
#70471=CARTESIAN_POINT('Ctrl Pts',(-3.84436848026,-38.2372245963,-9.4837558988));
#70472=CARTESIAN_POINT('Ctrl Pts',(-3.86796252798,-38.1627311721,-9.55446591759));
#70473=CARTESIAN_POINT('Ctrl Pts',(-3.87968490077,-38.0684833924,-9.58959720197));
#70474=CARTESIAN_POINT('Ctrl Pts',(-3.87968490077,-37.9742356128,-9.58959720197));
#70475=CARTESIAN_POINT('Ctrl Pts',(-3.29839571939,-38.2742356128,-9.45322376664));
#70476=CARTESIAN_POINT('Ctrl Pts',(-3.32416123403,-38.2742356128,-9.54393031556));
#70477=CARTESIAN_POINT('Ctrl Pts',(-3.34992674868,-38.2372245963,-9.63463686449));
#70478=CARTESIAN_POINT('Ctrl Pts',(-3.37029180577,-38.1627311721,-9.70633130082));
#70479=CARTESIAN_POINT('Ctrl Pts',(-3.38040989972,-38.0684833924,-9.74195167929));
#70480=CARTESIAN_POINT('Ctrl Pts',(-3.38040989972,-37.9742356128,-9.74195167929));
#70481=CARTESIAN_POINT('Ctrl Pts',(-3.01737322736,-38.2742356128,-9.52919900757));
#70482=CARTESIAN_POINT('Ctrl Pts',(-3.04081598292,-38.2742356128,-9.6205295628));
#70483=CARTESIAN_POINT('Ctrl Pts',(-3.06425873847,-38.2372245963,-9.71186011804));
#70484=CARTESIAN_POINT('Ctrl Pts',(-3.08278788744,-38.1627311721,-9.78404776885));
#70485=CARTESIAN_POINT('Ctrl Pts',(-3.09199383589,-38.0684833924,-9.81991319399));
#70486=CARTESIAN_POINT('Ctrl Pts',(-3.09199383589,-37.9742356128,-9.81991319399));
#70487=CARTESIAN_POINT('Ctrl Pts',(-2.63223226683,-38.2742356128,-9.62029211495));
#70488=CARTESIAN_POINT('Ctrl Pts',(-2.65256056107,-38.2742356128,-9.71235913547));
#70489=CARTESIAN_POINT('Ctrl Pts',(-2.67288885531,-38.2372245963,-9.804426156));
#70490=CARTESIAN_POINT('Ctrl Pts',(-2.68895633456,-38.1627311721,-9.87719590877));
#70491=CARTESIAN_POINT('Ctrl Pts',(-2.69693923708,-38.0684833924,-9.91335054319));
#70492=CARTESIAN_POINT('Ctrl Pts',(-2.69693923708,-37.9742356128,-9.91335054319));
#70493=CARTESIAN_POINT('Ctrl Pts',(-2.24379696979,-38.2742356128,-9.69540915194));
#70494=CARTESIAN_POINT('Ctrl Pts',(-2.26109407541,-38.2742356128,-9.78806117498));
#70495=CARTESIAN_POINT('Ctrl Pts',(-2.27839118104,-38.2372245963,-9.88071319803));
#70496=CARTESIAN_POINT('Ctrl Pts',(-2.29206280953,-38.1627311721,-9.95394533667));
#70497=CARTESIAN_POINT('Ctrl Pts',(-2.29885536701,-38.0684833924,-9.99032970104));
#70498=CARTESIAN_POINT('Ctrl Pts',(-2.29885536701,-37.9742356128,-9.99032970104));
#70499=CARTESIAN_POINT('Ctrl Pts',(-2.14030551313,-38.2742356128,-9.71427636052));
#70500=CARTESIAN_POINT('Ctrl Pts',(-2.15683710444,-38.2742356128,-9.80706985748));
#70501=CARTESIAN_POINT('Ctrl Pts',(-2.17336869575,-38.2372245963,-9.89986335443));
#70502=CARTESIAN_POINT('Ctrl Pts',(-2.18643526145,-38.1627311721,-9.97320731411));
#70503=CARTESIAN_POINT('Ctrl Pts',(-2.19292720261,-38.0684833924,-10.0096472351));
#70504=CARTESIAN_POINT('Ctrl Pts',(-2.19292720261,-37.9742356128,-10.0096472351));
#70505=CARTESIAN_POINT('Ctrl Pts',(-1.93885306926,-38.2742356128,-9.74872598301));
#70506=CARTESIAN_POINT('Ctrl Pts',(-1.95364426813,-38.2742356128,-9.84181234766));
#70507=CARTESIAN_POINT('Ctrl Pts',(-1.968435467,-38.2372245963,-9.93489871231));
#70508=CARTESIAN_POINT('Ctrl Pts',(-1.98012642784,-38.1627311721,-10.0084741544));
#70509=CARTESIAN_POINT('Ctrl Pts',(-1.98593491754,-38.0684833924,-10.0450290844));
#70510=CARTESIAN_POINT('Ctrl Pts',(-1.98593491754,-37.9742356128,-10.0450290844));
#70511=CARTESIAN_POINT('Ctrl Pts',(-1.70928454097,-38.2742356128,-9.78370121332));
#70512=CARTESIAN_POINT('Ctrl Pts',(-1.72312043005,-38.2742356128,-9.87692890895));
#70513=CARTESIAN_POINT('Ctrl Pts',(-1.73695631912,-38.2372245963,-9.97015660458));
#70514=CARTESIAN_POINT('Ctrl Pts',(-1.74789220221,-38.1627311721,-10.0438437548));
#70515=CARTESIAN_POINT('Ctrl Pts',(-1.75332554374,-38.0684833924,-10.0804541852));
#70516=CARTESIAN_POINT('Ctrl Pts',(-1.75332554374,-37.9742356128,-10.0804541852));
#70517=CARTESIAN_POINT('Ctrl Pts',(-1.58829686019,-38.2742356128,-9.80140839538));
#70518=CARTESIAN_POINT('Ctrl Pts',(-1.6018000959,-38.2742356128,-9.89468428557));
#70519=CARTESIAN_POINT('Ctrl Pts',(-1.61530333161,-38.2372245963,-9.98796017577));
#70520=CARTESIAN_POINT('Ctrl Pts',(-1.62597628817,-38.1627311721,-10.0616854186));
#70521=CARTESIAN_POINT('Ctrl Pts',(-1.6312789944,-38.0684833924,-10.0983147753));
#70522=CARTESIAN_POINT('Ctrl Pts',(-1.6312789944,-37.9742356128,-10.0983147753));
#70523=CARTESIAN_POINT('Ctrl Pts',(-1.46928796479,-38.2742356128,-9.81838209355));
#70524=CARTESIAN_POINT('Ctrl Pts',(-1.48253918237,-38.2742356128,-9.91169383936));
#70525=CARTESIAN_POINT('Ctrl Pts',(-1.49579039996,-38.2372245963,-10.0050055852));
#70526=CARTESIAN_POINT('Ctrl Pts',(-1.50626415805,-38.1627311721,-10.0787591687));
#70527=CARTESIAN_POINT('Ctrl Pts',(-1.51146790041,-38.0684833924,-10.1154026054));
#70528=CARTESIAN_POINT('Ctrl Pts',(-1.51146790041,-37.9742356128,-10.1154026054));
#70529=CARTESIAN_POINT('Ctrl Pts',(-1.34538313247,-38.2742356128,-9.83573533307));
#70530=CARTESIAN_POINT('Ctrl Pts',(-1.35845523278,-38.2742356128,-9.92907216478));
#70531=CARTESIAN_POINT('Ctrl Pts',(-1.37152733308,-38.2372245963,-10.0224089965));
#70532=CARTESIAN_POINT('Ctrl Pts',(-1.38185951829,-38.1627311721,-10.0961824078));
#70533=CARTESIAN_POINT('Ctrl Pts',(-1.38699292008,-38.0684833924,-10.1328356959));
#70534=CARTESIAN_POINT('Ctrl Pts',(-1.38699292008,-37.9742356128,-10.1328356959));
#70535=CARTESIAN_POINT('',(-1.38699292008,-37.9742356128,-10.1328356959));
#70536=CARTESIAN_POINT('Origin',(-1.34567653659528,-37.9763568755272,-9.83783619861542));
#70537=CARTESIAN_POINT('Ctrl Pts',(-1.38699292008,-37.9742356128,-10.1328356959));
#70538=CARTESIAN_POINT('Ctrl Pts',(-1.54048434157,-37.9742356128,-10.1113387667));
#70539=CARTESIAN_POINT('Ctrl Pts',(-1.68405004862,-37.9742356128,-10.0907690318));
#70540=CARTESIAN_POINT('Ctrl Pts',(-1.83768542132,-37.9742356128,-10.0680136807));
#70541=CARTESIAN_POINT('Ctrl Pts',(-2.0472685103,-37.9742356128,-10.0350233698));
#70542=CARTESIAN_POINT('Ctrl Pts',(-2.24744160945,-37.9742356128,-9.99950190736));
#70543=CARTESIAN_POINT('Ctrl Pts',(-2.32512404463,-37.9742356128,-9.9850708371));
#70544=CARTESIAN_POINT('Ctrl Pts',(-2.47861794583,-37.9742356128,-9.95531796778));
#70545=CARTESIAN_POINT('Ctrl Pts',(-2.63158870593,-37.9742356128,-9.9231347794));
#70546=CARTESIAN_POINT('Ctrl Pts',(-2.70802102444,-37.9742356128,-9.90641220658));
#70547=CARTESIAN_POINT('Ctrl Pts',(-3.01253146542,-37.9742356128,-9.83720045464));
#70548=CARTESIAN_POINT('Ctrl Pts',(-3.31446912355,-37.9742356128,-9.75814914822));
#70549=CARTESIAN_POINT('Ctrl Pts',(-3.53901439175,-37.9742356128,-9.69332241166));
#70550=CARTESIAN_POINT('Ctrl Pts',(-4.06616678433,-37.9742356128,-9.5265559109));
#70551=CARTESIAN_POINT('Ctrl Pts',(-4.58136980211,-37.9742356128,-9.32859973654));
#70552=CARTESIAN_POINT('Ctrl Pts',(-4.87486658275,-37.9742356128,-9.20377818652));
#70553=CARTESIAN_POINT('Ctrl Pts',(-5.45178039505,-37.9742356128,-8.9342344636));
#70554=CARTESIAN_POINT('Ctrl Pts',(-6.0085344695,-37.9742356128,-8.62630121912));
#70555=CARTESIAN_POINT('Ctrl Pts',(-6.28153293631,-37.9742356128,-8.46325996649));
#70556=CARTESIAN_POINT('Ctrl Pts',(-6.68293897529,-37.9742356128,-8.20578167081));
#70557=CARTESIAN_POINT('Ctrl Pts',(-7.07391925375,-37.9742356128,-7.9296599837));
#70558=CARTESIAN_POINT('Ctrl Pts',(-7.20312714751,-37.9742356128,-7.83561707231));
#70559=CARTESIAN_POINT('Ctrl Pts',(-7.71835943346,-37.9742356128,-7.44951290203));
#70560=CARTESIAN_POINT('Ctrl Pts',(-8.21985964705,-37.9742356128,-7.02884209138));
#70561=CARTESIAN_POINT('Ctrl Pts',(-8.58741395083,-37.9742356128,-6.694450027));
#70562=CARTESIAN_POINT('Ctrl Pts',(-9.23922565915,-37.9742356128,-6.04471661443));
#70563=CARTESIAN_POINT('Ctrl Pts',(-9.82149842759,-37.9742356128,-5.3259548207));
#70564=CARTESIAN_POINT('Ctrl Pts',(-10.0721843915,-37.9742356128,-4.97806710989));
#70565=CARTESIAN_POINT('Ctrl Pts',(-10.6524574839,-37.9742356128,-4.03375119461));
#70566=CARTESIAN_POINT('Ctrl Pts',(-11.0291793988,-37.9742356128,-2.98459593108));
#70567=CARTESIAN_POINT('Ctrl Pts',(-11.1622899814,-37.9742356128,-2.31636115633));
#70568=CARTESIAN_POINT('Ctrl Pts',(-11.2336540706,-37.9742356128,-1.36618233642));
#70569=CARTESIAN_POINT('Ctrl Pts',(-11.1889875368,-37.9742356128,-0.434883867537));
#70570=CARTESIAN_POINT('Ctrl Pts',(-11.1677658434,-37.9742356128,-0.163547364276));
#70571=CARTESIAN_POINT('Ctrl Pts',(-11.1309935407,-37.9742356128,0.191196052966));
#70572=CARTESIAN_POINT('Ctrl Pts',(-11.0837537732,-37.9742356128,0.541839826065));
#70573=CARTESIAN_POINT('Ctrl Pts',(-11.0714556362,-37.9742356128,0.62831585634));
#70574=CARTESIAN_POINT('Ctrl Pts',(-11.0585597994,-37.9742356128,0.714566551426));
#70575=CARTESIAN_POINT('Ctrl Pts',(-11.0450673741,-37.9742356128,0.800650704934));
#70576=CARTESIAN_POINT('Ctrl Pts',(-11.0450673741,-37.9742356128,0.800650704934));
#70577=CARTESIAN_POINT('Ctrl Pts',(-11.0450673741,-36.2942356128,0.800650704934));
#70578=CARTESIAN_POINT('Ctrl Pts',(-11.0585597994,-37.9742356128,0.714566551426));
#70579=CARTESIAN_POINT('Ctrl Pts',(-11.0585597994,-36.2942356128,0.714566551426));
#70580=CARTESIAN_POINT('Ctrl Pts',(-11.0714556362,-37.9742356128,0.62831585634));
#70581=CARTESIAN_POINT('Ctrl Pts',(-11.0714556362,-36.2942356128,0.62831585634));
#70582=CARTESIAN_POINT('Ctrl Pts',(-11.0837537732,-37.9742356128,0.541839826065));
#70583=CARTESIAN_POINT('Ctrl Pts',(-11.0837537732,-36.2942356128,0.541839826065));
#70584=CARTESIAN_POINT('Ctrl Pts',(-11.1309935407,-37.9742356128,0.191196052966));
#70585=CARTESIAN_POINT('Ctrl Pts',(-11.1309935407,-36.2942356128,0.191196052966));
#70586=CARTESIAN_POINT('Ctrl Pts',(-11.1677658434,-37.9742356128,-0.163547364276));
#70587=CARTESIAN_POINT('Ctrl Pts',(-11.1677658434,-36.2942356128,-0.163547364276));
#70588=CARTESIAN_POINT('Ctrl Pts',(-11.1889875368,-37.9742356128,-0.434883867537));
#70589=CARTESIAN_POINT('Ctrl Pts',(-11.1889875368,-36.2942356128,-0.434883867537));
#70590=CARTESIAN_POINT('Ctrl Pts',(-11.2336540706,-37.9742356128,-1.36618233642));
#70591=CARTESIAN_POINT('Ctrl Pts',(-11.2336540706,-36.2942356128,-1.36618233642));
#70592=CARTESIAN_POINT('Ctrl Pts',(-11.1622899814,-37.9742356128,-2.31636115633));
#70593=CARTESIAN_POINT('Ctrl Pts',(-11.1622899814,-36.2942356128,-2.31636115633));
#70594=CARTESIAN_POINT('Ctrl Pts',(-11.0291793988,-37.9742356128,-2.98459593108));
#70595=CARTESIAN_POINT('Ctrl Pts',(-11.0291793988,-36.2942356128,-2.98459593108));
#70596=CARTESIAN_POINT('Ctrl Pts',(-10.6524574839,-37.9742356128,-4.03375119461));
#70597=CARTESIAN_POINT('Ctrl Pts',(-10.6524574839,-36.2942356128,-4.03375119461));
#70598=CARTESIAN_POINT('Ctrl Pts',(-10.0721843915,-37.9742356128,-4.97806710989));
#70599=CARTESIAN_POINT('Ctrl Pts',(-10.0721843915,-36.2942356128,-4.97806710989));
#70600=CARTESIAN_POINT('Ctrl Pts',(-9.82149842759,-37.9742356128,-5.3259548207));
#70601=CARTESIAN_POINT('Ctrl Pts',(-9.82149842759,-36.2942356128,-5.3259548207));
#70602=CARTESIAN_POINT('Ctrl Pts',(-9.23922565915,-37.9742356128,-6.04471661443));
#70603=CARTESIAN_POINT('Ctrl Pts',(-9.23922565915,-36.2942356128,-6.04471661443));
#70604=CARTESIAN_POINT('Ctrl Pts',(-8.58741395083,-37.9742356128,-6.694450027));
#70605=CARTESIAN_POINT('Ctrl Pts',(-8.58741395083,-36.2942356128,-6.694450027));
#70606=CARTESIAN_POINT('Ctrl Pts',(-8.21985964705,-37.9742356128,-7.02884209138));
#70607=CARTESIAN_POINT('Ctrl Pts',(-8.21985964705,-36.2942356128,-7.02884209138));
#70608=CARTESIAN_POINT('Ctrl Pts',(-7.71835943346,-37.9742356128,-7.44951290203));
#70609=CARTESIAN_POINT('Ctrl Pts',(-7.71835943346,-36.2942356128,-7.44951290203));
#70610=CARTESIAN_POINT('Ctrl Pts',(-7.20312714751,-37.9742356128,-7.83561707231));
#70611=CARTESIAN_POINT('Ctrl Pts',(-7.20312714751,-36.2942356128,-7.83561707231));
#70612=CARTESIAN_POINT('Ctrl Pts',(-7.07391925375,-37.9742356128,-7.9296599837));
#70613=CARTESIAN_POINT('Ctrl Pts',(-7.07391925375,-36.2942356128,-7.9296599837));
#70614=CARTESIAN_POINT('Ctrl Pts',(-6.68293897529,-37.9742356128,-8.20578167081));
#70615=CARTESIAN_POINT('Ctrl Pts',(-6.68293897529,-36.2942356128,-8.20578167081));
#70616=CARTESIAN_POINT('Ctrl Pts',(-6.28153293631,-37.9742356128,-8.46325996649));
#70617=CARTESIAN_POINT('Ctrl Pts',(-6.28153293631,-36.2942356128,-8.46325996649));
#70618=CARTESIAN_POINT('Ctrl Pts',(-6.0085344695,-37.9742356128,-8.62630121912));
#70619=CARTESIAN_POINT('Ctrl Pts',(-6.0085344695,-36.2942356128,-8.62630121912));
#70620=CARTESIAN_POINT('Ctrl Pts',(-5.45178039505,-37.9742356128,-8.9342344636));
#70621=CARTESIAN_POINT('Ctrl Pts',(-5.45178039505,-36.2942356128,-8.9342344636));
#70622=CARTESIAN_POINT('Ctrl Pts',(-4.87486658275,-37.9742356128,-9.20377818652));
#70623=CARTESIAN_POINT('Ctrl Pts',(-4.87486658275,-36.2942356128,-9.20377818652));
#70624=CARTESIAN_POINT('Ctrl Pts',(-4.58136980211,-37.9742356128,-9.32859973654));
#70625=CARTESIAN_POINT('Ctrl Pts',(-4.58136980211,-36.2942356128,-9.32859973654));
#70626=CARTESIAN_POINT('Ctrl Pts',(-4.06616678433,-37.9742356128,-9.5265559109));
#70627=CARTESIAN_POINT('Ctrl Pts',(-4.06616678433,-36.2942356128,-9.5265559109));
#70628=CARTESIAN_POINT('Ctrl Pts',(-3.53901439175,-37.9742356128,-9.69332241166));
#70629=CARTESIAN_POINT('Ctrl Pts',(-3.53901439175,-36.2942356128,-9.69332241166));
#70630=CARTESIAN_POINT('Ctrl Pts',(-3.31446912355,-37.9742356128,-9.75814914822));
#70631=CARTESIAN_POINT('Ctrl Pts',(-3.31446912355,-36.2942356128,-9.75814914822));
#70632=CARTESIAN_POINT('Ctrl Pts',(-3.01253146542,-37.9742356128,-9.83720045464));
#70633=CARTESIAN_POINT('Ctrl Pts',(-3.01253146542,-36.2942356128,-9.83720045464));
#70634=CARTESIAN_POINT('Ctrl Pts',(-2.70802102444,-37.9742356128,-9.90641220658));
#70635=CARTESIAN_POINT('Ctrl Pts',(-2.70802102444,-36.2942356128,-9.90641220658));
#70636=CARTESIAN_POINT('Ctrl Pts',(-2.63158870593,-37.9742356128,-9.9231347794));
#70637=CARTESIAN_POINT('Ctrl Pts',(-2.63158870593,-36.2942356128,-9.9231347794));
#70638=CARTESIAN_POINT('Ctrl Pts',(-2.47861794583,-37.9742356128,-9.95531796778));
#70639=CARTESIAN_POINT('Ctrl Pts',(-2.47861794583,-36.2942356128,-9.95531796778));
#70640=CARTESIAN_POINT('Ctrl Pts',(-2.32512404463,-37.9742356128,-9.9850708371));
#70641=CARTESIAN_POINT('Ctrl Pts',(-2.32512404463,-36.2942356128,-9.9850708371));
#70642=CARTESIAN_POINT('Ctrl Pts',(-2.24744160945,-37.9742356128,-9.99950190736));
#70643=CARTESIAN_POINT('Ctrl Pts',(-2.24744160945,-36.2942356128,-9.99950190736));
#70644=CARTESIAN_POINT('Ctrl Pts',(-2.0472685103,-37.9742356128,-10.0350233698));
#70645=CARTESIAN_POINT('Ctrl Pts',(-2.0472685103,-36.2942356128,-10.0350233698));
#70646=CARTESIAN_POINT('Ctrl Pts',(-1.83768542132,-37.9742356128,-10.0680136807));
#70647=CARTESIAN_POINT('Ctrl Pts',(-1.83768542132,-36.2942356128,-10.0680136807));
#70648=CARTESIAN_POINT('Ctrl Pts',(-1.68405004862,-37.9742356128,-10.0907690318));
#70649=CARTESIAN_POINT('Ctrl Pts',(-1.68405004862,-36.2942356128,-10.0907690318));
#70650=CARTESIAN_POINT('Ctrl Pts',(-1.54048434157,-37.9742356128,-10.1113387667));
#70651=CARTESIAN_POINT('Ctrl Pts',(-1.54048434157,-36.2942356128,-10.1113387667));
#70652=CARTESIAN_POINT('Ctrl Pts',(-1.38699292008,-37.9742356128,-10.1328356959));
#70653=CARTESIAN_POINT('Ctrl Pts',(-1.38699292008,-36.2942356128,-10.1328356959));
#70654=CARTESIAN_POINT('',(-1.38699292008,-37.2742356128,-10.1328356959));
#70655=CARTESIAN_POINT('Ctrl Pts',(1.38699292008,-36.5742356128,-10.1328356959));
#70656=CARTESIAN_POINT('Ctrl Pts',(1.38699292008,-36.4799878332,-10.1328356959));
#70657=CARTESIAN_POINT('Ctrl Pts',(1.38185951829,-36.3857400536,-10.0961824078));
#70658=CARTESIAN_POINT('Ctrl Pts',(1.37152733308,-36.3112466293,-10.0224089965));
#70659=CARTESIAN_POINT('Ctrl Pts',(1.35845523278,-36.2742356128,-9.92907216478));
#70660=CARTESIAN_POINT('Ctrl Pts',(1.34538313247,-36.2742356128,-9.83573533307));
#70661=CARTESIAN_POINT('Ctrl Pts',(1.11136534535,-36.5742356128,-10.1714381558));
#70662=CARTESIAN_POINT('Ctrl Pts',(1.11136534535,-36.4799878332,-10.1714381558));
#70663=CARTESIAN_POINT('Ctrl Pts',(1.1072586023,-36.3857400536,-10.1346410811));
#70664=CARTESIAN_POINT('Ctrl Pts',(1.09899281062,-36.3112466293,-10.0605782652));
#70665=CARTESIAN_POINT('Ctrl Pts',(1.08853507531,-36.2742356128,-9.96687528396));
#70666=CARTESIAN_POINT('Ctrl Pts',(1.07807734001,-36.2742356128,-9.87317230266));
#70667=CARTESIAN_POINT('Ctrl Pts',(0.834409330039,-36.5742356128,-10.2003869648));
#70668=CARTESIAN_POINT('Ctrl Pts',(0.834409340739,-36.4799878342,-10.2003869633));
#70669=CARTESIAN_POINT('Ctrl Pts',(0.831329379193,-36.3857400556,-10.1634827365));
#70670=CARTESIAN_POINT('Ctrl Pts',(0.825130215053,-36.3112466317,-10.0892042535));
#70671=CARTESIAN_POINT('Ctrl Pts',(0.817287134283,-36.2742356144,-9.99522841452));
#70672=CARTESIAN_POINT('Ctrl Pts',(0.809444049232,-36.2742356128,-9.90125257547));
#70673=CARTESIAN_POINT('Ctrl Pts',(0.556562377033,-36.5742356128,-10.2196842577));
#70674=CARTESIAN_POINT('Ctrl Pts',(0.556562398806,-36.4799878341,-10.2196842562));
#70675=CARTESIAN_POINT('Ctrl Pts',(0.554510558535,-36.3857400553,-10.1827090256));
#70676=CARTESIAN_POINT('Ctrl Pts',(0.550380660272,-36.3112466314,-10.1082876224));
#70677=CARTESIAN_POINT('Ctrl Pts',(0.545155596145,-36.2742356142,-10.0141309667));
#70678=CARTESIAN_POINT('Ctrl Pts',(0.539930523441,-36.2742356128,-9.91997431098));
#70679=CARTESIAN_POINT('Ctrl Pts',(5.42079519942E-6,-36.5742356128,-10.2389842343));
#70680=CARTESIAN_POINT('Ctrl Pts',(5.4533884471E-6,-36.4799878334,-10.2389842343));
#70681=CARTESIAN_POINT('Ctrl Pts',(4.06209988914E-6,-36.3857400539,-10.2019373985));
#70682=CARTESIAN_POINT('Ctrl Pts',(1.27978273706E-6,-36.3112466296,-10.1273718877));
#70683=CARTESIAN_POINT('Ctrl Pts',(-2.28441439194E-6,-36.274235613,-10.033032902));
#70684=CARTESIAN_POINT('Ctrl Pts',(-5.86138357242E-6,-36.2742356128,-9.93869391623));
#70685=CARTESIAN_POINT('Ctrl Pts',(-0.556573758695,-36.5742356128,-10.2196842429));
#70686=CARTESIAN_POINT('Ctrl Pts',(-0.556573737115,-36.4799878321,-10.2196842444));
#70687=CARTESIAN_POINT('Ctrl Pts',(-0.554519003891,-36.3857400514,-10.1827090156));
#70688=CARTESIAN_POINT('Ctrl Pts',(-0.550383451506,-36.3112466267,-10.1082876123));
#70689=CARTESIAN_POINT('Ctrl Pts',(-0.545151211684,-36.2742356111,-10.0141309554));
#70690=CARTESIAN_POINT('Ctrl Pts',(-0.539918980363,-36.2742356128,-9.91997429864));
#70691=CARTESIAN_POINT('Ctrl Pts',(-0.83438718174,-36.5742356128,-10.2003905389));
#70692=CARTESIAN_POINT('Ctrl Pts',(-0.834387171416,-36.4799878328,-10.2003905404));
#70693=CARTESIAN_POINT('Ctrl Pts',(-0.831312895645,-36.3857400527,-10.1634855111));
#70694=CARTESIAN_POINT('Ctrl Pts',(-0.825124969885,-36.3112466283,-10.0892054421));
#70695=CARTESIAN_POINT('Ctrl Pts',(-0.817296217687,-36.2742356121,-9.99522758151));
#70696=CARTESIAN_POINT('Ctrl Pts',(-0.809467469578,-36.2742356128,-9.90124972058));
#70697=CARTESIAN_POINT('Ctrl Pts',(-1.11138042468,-36.5742356128,-10.1714357354));
#70698=CARTESIAN_POINT('Ctrl Pts',(-1.11138042478,-36.4799878329,-10.1714357354));
#70699=CARTESIAN_POINT('Ctrl Pts',(-1.10726985602,-36.385740053,-10.1346391998));
#70700=CARTESIAN_POINT('Ctrl Pts',(-1.09899651827,-36.3112466286,-10.0605774471));
#70701=CARTESIAN_POINT('Ctrl Pts',(-1.08852917102,-36.2742356123,-9.96687582026));
#70702=CARTESIAN_POINT('Ctrl Pts',(-1.07806182375,-36.2742356128,-9.87317419359));
#70703=CARTESIAN_POINT('Ctrl Pts',(-1.38699292042,-36.5742356128,-10.1328356979));
#70704=CARTESIAN_POINT('Ctrl Pts',(-1.38699292042,-36.4799878332,-10.1328356979));
#70705=CARTESIAN_POINT('Ctrl Pts',(-1.3818595472,-36.3857400536,-10.0961824057));
#70706=CARTESIAN_POINT('Ctrl Pts',(-1.37152741947,-36.3112466294,-10.0224089864));
#70707=CARTESIAN_POINT('Ctrl Pts',(-1.3584553919,-36.2742356128,-9.92907214443));
#70708=CARTESIAN_POINT('Ctrl Pts',(-1.34538336432,-36.2742356128,-9.83573530247));
#70709=CARTESIAN_POINT('',(1.38699292008,-36.5742356128,-10.1328356959));
#70710=CARTESIAN_POINT('Origin',(1.34567723997399,-36.5721143211205,-9.83783613747388));
#70711=CARTESIAN_POINT('Origin',(1.27675647831893E-14,-36.5742356128,-2.72395521665914));
#70712=CARTESIAN_POINT('Ctrl Pts',(-1.34538263085,-38.2742356128,-9.83573538825));
#70713=CARTESIAN_POINT('Ctrl Pts',(-1.35845488787,-38.2742356128,-9.92907219763));
#70714=CARTESIAN_POINT('Ctrl Pts',(-1.37152714489,-38.2372245963,-10.022409007));
#70715=CARTESIAN_POINT('Ctrl Pts',(-1.38185945397,-38.1627311721,-10.0961824006));
#70716=CARTESIAN_POINT('Ctrl Pts',(-1.3869929173,-38.0684833924,-10.13283568));
#70717=CARTESIAN_POINT('Ctrl Pts',(-1.3869929173,-37.9742356128,-10.13283568));
#70718=CARTESIAN_POINT('Ctrl Pts',(-1.07805458856,-38.2742356128,-9.87317534285));
#70719=CARTESIAN_POINT('Ctrl Pts',(-1.08852516046,-38.2742356128,-9.96687652205));
#70720=CARTESIAN_POINT('Ctrl Pts',(-1.09899573236,-38.2372245963,-10.0605777012));
#70721=CARTESIAN_POINT('Ctrl Pts',(-1.10727163244,-38.1627311721,-10.1346390981));
#70722=CARTESIAN_POINT('Ctrl Pts',(-1.11138345406,-38.0684833924,-10.1714354597));
#70723=CARTESIAN_POINT('Ctrl Pts',(-1.11138345406,-37.9742356128,-10.1714354597));
#70724=CARTESIAN_POINT('Ctrl Pts',(-0.809472541664,-38.2742356128,-9.90124868745));
#70725=CARTESIAN_POINT('Ctrl Pts',(-0.817296138563,-38.2742356128,-9.99522725993));
#70726=CARTESIAN_POINT('Ctrl Pts',(-0.825119735463,-38.2372245963,-10.0892058324));
#70727=CARTESIAN_POINT('Ctrl Pts',(-0.83130356121,-38.1627311721,-10.1634864674));
#70728=CARTESIAN_POINT('Ctrl Pts',(-0.83437582405,-38.0684833924,-10.2003917745));
#70729=CARTESIAN_POINT('Ctrl Pts',(-0.83437582405,-37.9742356128,-10.2003917745));
#70730=CARTESIAN_POINT('Ctrl Pts',(-0.539912794952,-38.2742356128,-9.91997481745));
#70731=CARTESIAN_POINT('Ctrl Pts',(-0.545145819039,-38.2742356128,-10.0141312189));
#70732=CARTESIAN_POINT('Ctrl Pts',(-0.550378843126,-38.2372245963,-10.1082876203));
#70733=CARTESIAN_POINT('Ctrl Pts',(-0.554515025793,-38.1627311721,-10.1827088234));
#70734=CARTESIAN_POINT('Ctrl Pts',(-0.556570027967,-38.0684833924,-10.2196839516));
#70735=CARTESIAN_POINT('Ctrl Pts',(-0.556570027967,-37.9742356128,-10.2196839516));
#70736=CARTESIAN_POINT('Ctrl Pts',(-6.58122985814E-6,-38.2742356128,-9.93869363588));
#70737=CARTESIAN_POINT('Ctrl Pts',(-2.11071485614E-6,-38.2742356128,-10.0330328354));
#70738=CARTESIAN_POINT('Ctrl Pts',(2.35980014682E-6,-38.2372245963,-10.1273720349));
#70739=CARTESIAN_POINT('Ctrl Pts',(5.89487381069E-6,-38.1627311721,-10.2019377133));
#70740=CARTESIAN_POINT('Ctrl Pts',(7.64886135792E-6,-38.0684833924,-10.2389846345));
#70741=CARTESIAN_POINT('Ctrl Pts',(7.64886135792E-6,-37.9742356128,-10.2389846345));
#70742=CARTESIAN_POINT('Ctrl Pts',(0.539931096955,-38.2742356128,-9.91997471322));
#70743=CARTESIAN_POINT('Ctrl Pts',(0.545155312685,-38.2742356128,-10.0141311006));
#70744=CARTESIAN_POINT('Ctrl Pts',(0.550379528416,-38.2372245963,-10.1082874879));
#70745=CARTESIAN_POINT('Ctrl Pts',(0.554508745802,-38.1627311721,-10.18270868));
#70746=CARTESIAN_POINT('Ctrl Pts',(0.556560292102,-38.0684833924,-10.2196838026));
#70747=CARTESIAN_POINT('Ctrl Pts',(0.556560292102,-37.9742356128,-10.2196838026));
#70748=CARTESIAN_POINT('Ctrl Pts',(0.809437211467,-38.2742356128,-9.90125321466));
#70749=CARTESIAN_POINT('Ctrl Pts',(0.817279129002,-38.2742356128,-9.99522921039));
#70750=CARTESIAN_POINT('Ctrl Pts',(0.825121046537,-38.2372245963,-10.0892052061));
#70751=CARTESIAN_POINT('Ctrl Pts',(0.831319359229,-38.1627311721,-10.1634838037));
#70752=CARTESIAN_POINT('Ctrl Pts',(0.834398810248,-38.0684833924,-10.2003880997));
#70753=CARTESIAN_POINT('Ctrl Pts',(0.834398810248,-37.9742356128,-10.2003880997));
#70754=CARTESIAN_POINT('Ctrl Pts',(1.07807579453,-38.2742356128,-9.87317251911));
#70755=CARTESIAN_POINT('Ctrl Pts',(1.08853351472,-38.2742356128,-9.96687550252));
#70756=CARTESIAN_POINT('Ctrl Pts',(1.09899123491,-38.2372245963,-10.0605784859));
#70757=CARTESIAN_POINT('Ctrl Pts',(1.10725697278,-38.1627311721,-10.1346413093));
#70758=CARTESIAN_POINT('Ctrl Pts',(1.11136375176,-38.0684833924,-10.171438379));
#70759=CARTESIAN_POINT('Ctrl Pts',(1.11136375176,-37.9742356128,-10.171438379));
#70760=CARTESIAN_POINT('Ctrl Pts',(1.34538313247,-38.2742356128,-9.83573533307));
#70761=CARTESIAN_POINT('Ctrl Pts',(1.35845523278,-38.2742356128,-9.92907216478));
#70762=CARTESIAN_POINT('Ctrl Pts',(1.37152733308,-38.2372245963,-10.0224089965));
#70763=CARTESIAN_POINT('Ctrl Pts',(1.38185951829,-38.1627311721,-10.0961824078));
#70764=CARTESIAN_POINT('Ctrl Pts',(1.38699292008,-38.0684833924,-10.1328356959));
#70765=CARTESIAN_POINT('Ctrl Pts',(1.38699292008,-37.9742356128,-10.1328356959));
#70766=CARTESIAN_POINT('',(1.38700644577,-37.9742356128,-10.1328338118));
#70767=CARTESIAN_POINT('Origin',(1.34569970434081,-37.9763569227614,-9.83783301687873));
#70768=CARTESIAN_POINT('Origin',(0.,-37.9742356128,-2.72395521670843));
#70769=CARTESIAN_POINT('Ctrl Pts',(-1.38699292008,-37.9742356128,-10.1328356959));
#70770=CARTESIAN_POINT('Ctrl Pts',(-1.38699292008,-36.2942356128,-10.1328356959));
#70771=CARTESIAN_POINT('Ctrl Pts',(-0.835781068554,-37.9742356128,-10.2100345517));
#70772=CARTESIAN_POINT('Ctrl Pts',(-0.835781068554,-36.2942356128,-10.2100345517));
#70773=CARTESIAN_POINT('Ctrl Pts',(-0.27919124227,-37.9742356128,-10.2486339796));
#70774=CARTESIAN_POINT('Ctrl Pts',(-0.27919124227,-36.2942356128,-10.2486339796));
#70775=CARTESIAN_POINT('Ctrl Pts',(0.27919124227,-37.9742356128,-10.2486339796));
#70776=CARTESIAN_POINT('Ctrl Pts',(0.27919124227,-36.2942356128,-10.2486339796));
#70777=CARTESIAN_POINT('Ctrl Pts',(0.835781068554,-37.9742356128,-10.2100345517));
#70778=CARTESIAN_POINT('Ctrl Pts',(0.835781068554,-36.2942356128,-10.2100345517));
#70779=CARTESIAN_POINT('Ctrl Pts',(1.38699292008,-37.9742356128,-10.1328356959));
#70780=CARTESIAN_POINT('Ctrl Pts',(1.38699292008,-36.2942356128,-10.1328356959));
#70781=CARTESIAN_POINT('',(1.38699292008,-37.2742356128,-10.1328356959));
#70782=CARTESIAN_POINT('Ctrl Pts',(11.0450673604,-36.5742356128,0.80065078572));
#70783=CARTESIAN_POINT('Ctrl Pts',(11.045067361,-36.4799878332,0.800650781683));
#70784=CARTESIAN_POINT('Ctrl Pts',(11.0085027593,-36.3857400536,0.794919704988));
#70785=CARTESIAN_POINT('Ctrl Pts',(10.9349078496,-36.3112466293,0.783384562601));
#70786=CARTESIAN_POINT('Ctrl Pts',(10.8417968545,-36.2742356128,0.768790504329));
#70787=CARTESIAN_POINT('Ctrl Pts',(10.7486858592,-36.2742356128,0.754196447643));
#70788=CARTESIAN_POINT('Ctrl Pts',(11.1590945635,-36.5742356128,0.0731427823434));
#70789=CARTESIAN_POINT('Ctrl Pts',(11.1590943539,-36.4799878336,0.0731441086594));
#70790=CARTESIAN_POINT('Ctrl Pts',(11.122250057,-36.3857400543,0.0691974113034));
#70791=CARTESIAN_POINT('Ctrl Pts',(11.0480924687,-36.3112466301,0.0612520226421));
#70792=CARTESIAN_POINT('Ctrl Pts',(10.9542697034,-36.2742356134,0.051198890854));
#70793=CARTESIAN_POINT('Ctrl Pts',(10.8604470201,-36.2742356128,0.0411452401641));
#70794=CARTESIAN_POINT('Ctrl Pts',(11.2300205496,-36.5742356128,-0.665529030045));
#70795=CARTESIAN_POINT('Ctrl Pts',(11.2300208596,-36.4799878483,-0.66553104165));
#70796=CARTESIAN_POINT('Ctrl Pts',(11.1930302198,-36.3857400837,-0.667764985107));
#70797=CARTESIAN_POINT('Ctrl Pts',(11.1185774042,-36.3112466648,-0.672258707664));
#70798=CARTESIAN_POINT('Ctrl Pts',(11.0243808176,-36.2742356365,-0.677942925129));
#70799=CARTESIAN_POINT('Ctrl Pts',(10.9301841004,-36.2742356128,-0.683626353818));
#70800=CARTESIAN_POINT('Ctrl Pts',(11.2586691615,-36.5742356128,-1.43857902297));
#70801=CARTESIAN_POINT('Ctrl Pts',(11.2586691082,-36.4799878202,-1.43857844952));
#70802=CARTESIAN_POINT('Ctrl Pts',(11.2213359158,-36.3857400276,-1.43764120566));
#70803=CARTESIAN_POINT('Ctrl Pts',(11.1461941074,-36.3112465987,-1.43575552205));
#70804=CARTESIAN_POINT('Ctrl Pts',(11.0511260388,-36.2742355924,-1.43337012132));
#70805=CARTESIAN_POINT('Ctrl Pts',(10.956057999,-36.2742356128,-1.43098494596));
#70806=CARTESIAN_POINT('Ctrl Pts',(11.1287255199,-36.5742356128,-2.62842434011));
#70807=CARTESIAN_POINT('Ctrl Pts',(11.1287255488,-36.4799878403,-2.62842465101));
#70808=CARTESIAN_POINT('Ctrl Pts',(11.0920269838,-36.3857400677,-2.62101538779));
#70809=CARTESIAN_POINT('Ctrl Pts',(11.0181624037,-36.311246646,-2.60610209162));
#70810=CARTESIAN_POINT('Ctrl Pts',(10.9247102077,-36.2742356239,-2.5872338689));
#70811=CARTESIAN_POINT('Ctrl Pts',(10.831257996,-36.2742356128,-2.56836552398));
#70812=CARTESIAN_POINT('Ctrl Pts',(10.7310385841,-36.5742356128,-3.75973072379));
#70813=CARTESIAN_POINT('Ctrl Pts',(10.7310385684,-36.4799878294,-3.75973055523));
#70814=CARTESIAN_POINT('Ctrl Pts',(10.6966894642,-36.385740046,-3.74560929459));
#70815=CARTESIAN_POINT('Ctrl Pts',(10.6275537888,-36.3112466203,-3.71718713519));
#70816=CARTESIAN_POINT('Ctrl Pts',(10.54008455,-36.2742356068,-3.68122801356));
#70817=CARTESIAN_POINT('Ctrl Pts',(10.4526153195,-36.2742356128,-3.64526895817));
#70818=CARTESIAN_POINT('Ctrl Pts',(10.5562244357,-36.5742356128,-4.14577572839));
#70819=CARTESIAN_POINT('Ctrl Pts',(10.5562244337,-36.4799878354,-4.14577573503));
#70820=CARTESIAN_POINT('Ctrl Pts',(10.5229141043,-36.385740058,-4.12938259431));
#70821=CARTESIAN_POINT('Ctrl Pts',(10.4558691905,-36.3112466344,-4.09638751326));
#70822=CARTESIAN_POINT('Ctrl Pts',(10.3710451368,-36.2742356162,-4.05464270841));
#70823=CARTESIAN_POINT('Ctrl Pts',(10.2862210827,-36.2742356128,-4.01289790025));
#70824=CARTESIAN_POINT('Ctrl Pts',(10.1185165315,-36.5742356128,-4.93605874865));
#70825=CARTESIAN_POINT('Ctrl Pts',(10.1185165338,-36.4799878308,-4.93605874107));
#70826=CARTESIAN_POINT('Ctrl Pts',(10.0876389665,-36.3857400487,-4.9153527052));
#70827=CARTESIAN_POINT('Ctrl Pts',(10.0254905563,-36.3112466235,-4.8736769201));
#70828=CARTESIAN_POINT('Ctrl Pts',(9.94686147247,-36.274235609,-4.82094944962));
#70829=CARTESIAN_POINT('Ctrl Pts',(9.868232389,-36.2742356128,-4.76822198291));
#70830=CARTESIAN_POINT('Ctrl Pts',(9.56890441447,-36.5742356128,-5.65332240208));
#70831=CARTESIAN_POINT('Ctrl Pts',(9.56890441181,-36.4799878361,-5.65332241073));
#70832=CARTESIAN_POINT('Ctrl Pts',(9.54035667914,-36.3857400593,-5.62965790004));
#70833=CARTESIAN_POINT('Ctrl Pts',(9.48289761876,-36.311246636,-5.5820274647));
#70834=CARTESIAN_POINT('Ctrl Pts',(9.41020141946,-36.2742356173,-5.52176626379));
#70835=CARTESIAN_POINT('Ctrl Pts',(9.33750521971,-36.2742356128,-5.46150505857));
#70836=CARTESIAN_POINT('Ctrl Pts',(9.25594847982,-36.5742356128,-6.01159034787));
#70837=CARTESIAN_POINT('Ctrl Pts',(9.2559484841,-36.4799878361,-6.01159034444));
#70838=CARTESIAN_POINT('Ctrl Pts',(9.22850758179,-36.3857400593,-5.98668964763));
#70839=CARTESIAN_POINT('Ctrl Pts',(9.17327627072,-36.311246636,-5.93657111006));
#70840=CARTESIAN_POINT('Ctrl Pts',(9.10339857703,-36.2742356173,-5.87316201272));
#70841=CARTESIAN_POINT('Ctrl Pts',(9.03352088058,-36.2742356128,-5.80975291532));
#70842=CARTESIAN_POINT('Ctrl Pts',(8.60187015157,-36.5742356128,-6.68997127933));
#70843=CARTESIAN_POINT('Ctrl Pts',(8.60187014738,-36.4799878305,-6.68997128269));
#70844=CARTESIAN_POINT('Ctrl Pts',(8.57641889755,-36.3857400481,-6.66302157178));
#70845=CARTESIAN_POINT('Ctrl Pts',(8.52519224274,-36.3112466228,-6.60877890052));
#70846=CARTESIAN_POINT('Ctrl Pts',(8.46038117687,-36.2742356085,-6.54015201885));
#70847=CARTESIAN_POINT('Ctrl Pts',(8.39557011371,-36.2742356128,-6.47152513724));
#70848=CARTESIAN_POINT('Ctrl Pts',(7.89889535824,-36.5742356128,-7.30184497632));
#70849=CARTESIAN_POINT('Ctrl Pts',(7.89889536235,-36.479987836,-7.30184497303));
#70850=CARTESIAN_POINT('Ctrl Pts',(7.87520178124,-36.3857400591,-7.27338138171));
#70851=CARTESIAN_POINT('Ctrl Pts',(7.82751284046,-36.3112466358,-7.21609167633));
#70852=CARTESIAN_POINT('Ctrl Pts',(7.76717762213,-36.2742356171,-7.14360974255));
#70853=CARTESIAN_POINT('Ctrl Pts',(7.70684240115,-36.2742356128,-7.07112780873));
#70854=CARTESIAN_POINT('Ctrl Pts',(7.54206117235,-36.5742356128,-7.58966580122));
#70855=CARTESIAN_POINT('Ctrl Pts',(7.5420611681,-36.4799878303,-7.58966580444));
#70856=CARTESIAN_POINT('Ctrl Pts',(7.51923353688,-36.3857400477,-7.56050216317));
#70857=CARTESIAN_POINT('Ctrl Pts',(7.47328753544,-36.3112466223,-7.50180343345));
#70858=CARTESIAN_POINT('Ctrl Pts',(7.41515745994,-36.2742356082,-7.42753882464));
#70859=CARTESIAN_POINT('Ctrl Pts',(7.35702738724,-36.2742356128,-7.35327421602));
#70860=CARTESIAN_POINT('Ctrl Pts',(6.81974100977,-36.5742356128,-8.12924918963));
#70861=CARTESIAN_POINT('Ctrl Pts',(6.81974101401,-36.4799878362,-8.12924918643));
#70862=CARTESIAN_POINT('Ctrl Pts',(6.79873299015,-36.3857400596,-8.09871470869));
#70863=CARTESIAN_POINT('Ctrl Pts',(6.75644936833,-36.3112466363,-8.03725685438));
#70864=CARTESIAN_POINT('Ctrl Pts',(6.70295286504,-36.2742356175,-7.95950145129));
#70865=CARTESIAN_POINT('Ctrl Pts',(6.64945635896,-36.2742356128,-7.88174604801));
#70866=CARTESIAN_POINT('Ctrl Pts',(6.05811766031,-36.5742356128,-8.60451307516));
#70867=CARTESIAN_POINT('Ctrl Pts',(6.05811765609,-36.4799878303,-8.60451307836));
#70868=CARTESIAN_POINT('Ctrl Pts',(6.03938391395,-36.3857400477,-8.57254968367));
#70869=CARTESIAN_POINT('Ctrl Pts',(6.00167783198,-36.3112466224,-8.50821578835));
#70870=CARTESIAN_POINT('Ctrl Pts',(5.95397275891,-36.2742356082,-8.42682166631));
#70871=CARTESIAN_POINT('Ctrl Pts',(5.90626768861,-36.2742356128,-8.34542754446));
#70872=CARTESIAN_POINT('Ctrl Pts',(5.66726526532,-36.5742356128,-8.82396239702));
#70873=CARTESIAN_POINT('Ctrl Pts',(5.66726527346,-36.4799878325,-8.82396239323));
#70874=CARTESIAN_POINT('Ctrl Pts',(5.64974730298,-36.3857400521,-8.79131270234));
#70875=CARTESIAN_POINT('Ctrl Pts',(5.6144882341,-36.3112466275,-8.72559748206));
#70876=CARTESIAN_POINT('Ctrl Pts',(5.56987907103,-36.2742356116,-8.64245573545));
#70877=CARTESIAN_POINT('Ctrl Pts',(5.52526990488,-36.2742356128,-8.5593139908));
#70878=CARTESIAN_POINT('Ctrl Pts',(5.06534643699,-36.5742356128,-9.12478048112));
#70879=CARTESIAN_POINT('Ctrl Pts',(5.06534643293,-36.4799878336,-9.12478048301));
#70880=CARTESIAN_POINT('Ctrl Pts',(5.04976009616,-36.3857400544,-9.09116389237));
#70881=CARTESIAN_POINT('Ctrl Pts',(5.01838891207,-36.3112466303,-9.02350255063));
#70882=CARTESIAN_POINT('Ctrl Pts',(4.97869864017,-36.2742356134,-8.93789860125));
#70883=CARTESIAN_POINT('Ctrl Pts',(4.93900836982,-36.2742356128,-8.8522946509));
#70884=CARTESIAN_POINT('Ctrl Pts',(4.44254377917,-36.5742356128,-9.38061203627));
#70885=CARTESIAN_POINT('Ctrl Pts',(4.44254378121,-36.479987833,-9.38061203532));
#70886=CARTESIAN_POINT('Ctrl Pts',(4.42898621881,-36.3857400532,-9.3461619704));
#70887=CARTESIAN_POINT('Ctrl Pts',(4.40169841545,-36.3112466289,-9.27682306804));
#70888=CARTESIAN_POINT('Ctrl Pts',(4.36717436193,-36.2742356125,-9.18909670022));
#70889=CARTESIAN_POINT('Ctrl Pts',(4.33265030764,-36.2742356128,-9.10137033288));
#70890=CARTESIAN_POINT('Ctrl Pts',(4.23279656972,-36.5742356128,-9.46077263537));
#70891=CARTESIAN_POINT('Ctrl Pts',(4.23279657536,-36.4799878331,-9.46077263319));
#70892=CARTESIAN_POINT('Ctrl Pts',(4.21992355351,-36.3857400533,-9.42606097103));
#70893=CARTESIAN_POINT('Ctrl Pts',(4.19401354548,-36.3112466289,-9.35619554385));
#70894=CARTESIAN_POINT('Ctrl Pts',(4.16123265235,-36.2742356126,-9.26780302676));
#70895=CARTESIAN_POINT('Ctrl Pts',(4.12845175702,-36.2742356128,-9.17941051062));
#70896=CARTESIAN_POINT('Ctrl Pts',(3.80923512589,-36.5742356128,-9.61074441909));
#70897=CARTESIAN_POINT('Ctrl Pts',(3.80923513444,-36.4799878343,-9.61074441627));
#70898=CARTESIAN_POINT('Ctrl Pts',(3.79773947086,-36.3857400557,-9.57554539274));
#70899=CARTESIAN_POINT('Ctrl Pts',(3.77460171857,-36.3112466318,-9.50469903632));
#70900=CARTESIAN_POINT('Ctrl Pts',(3.74532823308,-36.2742356145,-9.4150654646));
#70901=CARTESIAN_POINT('Ctrl Pts',(3.716054744,-36.2742356128,-9.32543189337));
#70902=CARTESIAN_POINT('Ctrl Pts',(3.37823722599,-36.5742356128,-9.73997950077));
#70903=CARTESIAN_POINT('Ctrl Pts',(3.37823723183,-36.4799878348,-9.73997949916));
#70904=CARTESIAN_POINT('Ctrl Pts',(3.36812208699,-36.3857400568,-9.7043667315));
#70905=CARTESIAN_POINT('Ctrl Pts',(3.34776295853,-36.3112466331,-9.63268761569));
#70906=CARTESIAN_POINT('Ctrl Pts',(3.32200494097,-36.2742356153,-9.54200045039));
#70907=CARTESIAN_POINT('Ctrl Pts',(3.29624692084,-36.2742356128,-9.45131328477));
#70908=CARTESIAN_POINT('Ctrl Pts',(3.16149193513,-36.5742356128,-9.79931128721));
#70909=CARTESIAN_POINT('Ctrl Pts',(3.16149192019,-36.4799878339,-9.7993112903));
#70910=CARTESIAN_POINT('Ctrl Pts',(3.15207526541,-36.3857400549,-9.76350879732));
#70911=CARTESIAN_POINT('Ctrl Pts',(3.13312203699,-36.3112466308,-9.69144780897));
#70912=CARTESIAN_POINT('Ctrl Pts',(3.10914275311,-36.2742356138,-9.60027750259));
#70913=CARTESIAN_POINT('Ctrl Pts',(3.085163475,-36.2742356128,-9.50910719462));
#70914=CARTESIAN_POINT('Ctrl Pts',(2.82069093435,-36.5742356128,-9.88383207656));
#70915=CARTESIAN_POINT('Ctrl Pts',(2.82069094264,-36.4799878329,-9.88383207485));
#70916=CARTESIAN_POINT('Ctrl Pts',(2.81231719671,-36.3857400529,-9.84777000922));
#70917=CARTESIAN_POINT('Ctrl Pts',(2.79546304335,-36.3112466285,-9.77518657496));
#70918=CARTESIAN_POINT('Ctrl Pts',(2.77413945741,-36.2742356123,-9.68335528262));
#70919=CARTESIAN_POINT('Ctrl Pts',(2.75281586826,-36.2742356128,-9.59152399117));
#70920=CARTESIAN_POINT('Ctrl Pts',(2.4779858176,-36.5742356128,-9.95579014891));
#70921=CARTESIAN_POINT('Ctrl Pts',(2.47798581299,-36.4799878334,-9.95579014986));
#70922=CARTESIAN_POINT('Ctrl Pts',(2.47066165835,-36.385740054,-9.91950820283));
#70923=CARTESIAN_POINT('Ctrl Pts',(2.45592006997,-36.3112466298,-9.84648220223));
#70924=CARTESIAN_POINT('Ctrl Pts',(2.43726927277,-36.2742356132,-9.75409098075));
#70925=CARTESIAN_POINT('Ctrl Pts',(2.41861847736,-36.2742356128,-9.66169975877));
#70926=CARTESIAN_POINT('Ctrl Pts',(2.35465529944,-36.5742356128,-9.98006182258));
#70927=CARTESIAN_POINT('Ctrl Pts',(2.35465523153,-36.4799878333,-9.98006183247));
#70928=CARTESIAN_POINT('Ctrl Pts',(2.34769194242,-36.3857400538,-9.94370911603));
#70929=CARTESIAN_POINT('Ctrl Pts',(2.33367676219,-36.3112466296,-9.87054066385));
#70930=CARTESIAN_POINT('Ctrl Pts',(2.31594504154,-36.274235613,-9.77796920984));
#70931=CARTESIAN_POINT('Ctrl Pts',(2.29821334717,-36.2742356128,-9.68539775193));
#70932=CARTESIAN_POINT('Ctrl Pts',(2.10245396246,-36.5742356128,-10.0263413789));
#70933=CARTESIAN_POINT('Ctrl Pts',(2.10245403384,-36.4799878331,-10.0263413685));
#70934=CARTESIAN_POINT('Ctrl Pts',(2.09626771326,-36.3857400534,-9.98984574067));
#70935=CARTESIAN_POINT('Ctrl Pts',(2.08381618659,-36.3112466291,-9.91638967147));
#70936=CARTESIAN_POINT('Ctrl Pts',(2.06806269103,-36.2742356127,-9.82345434149));
#70937=CARTESIAN_POINT('Ctrl Pts',(2.05230916782,-36.2742356128,-9.73051901561));
#70938=CARTESIAN_POINT('Ctrl Pts',(1.84363587601,-36.5742356128,-10.0671337109));
#70939=CARTESIAN_POINT('Ctrl Pts',(1.84363580098,-36.4799878334,-10.0671337218));
#70940=CARTESIAN_POINT('Ctrl Pts',(1.8381321438,-36.3857400539,-10.0305323548));
#70941=CARTESIAN_POINT('Ctrl Pts',(1.82705483329,-36.3112466296,-9.95686343242));
#70942=CARTESIAN_POINT('Ctrl Pts',(1.8130400557,-36.274235613,-9.863658792));
#70943=CARTESIAN_POINT('Ctrl Pts',(1.79902530718,-36.2742356128,-9.77045414726));
#70944=CARTESIAN_POINT('Ctrl Pts',(1.68657601118,-36.5742356128,-10.090407293));
#70945=CARTESIAN_POINT('Ctrl Pts',(1.68657610781,-36.4799878388,-10.0904072805));
#70946=CARTESIAN_POINT('Ctrl Pts',(1.68120354795,-36.3857400648,-10.0537882489));
#70947=CARTESIAN_POINT('Ctrl Pts',(1.67038985815,-36.3112466425,-9.98008380584));
#70948=CARTESIAN_POINT('Ctrl Pts',(1.65670851502,-36.2742356216,-9.88683423583));
#70949=CARTESIAN_POINT('Ctrl Pts',(1.643027135,-36.2742356128,-9.79358466713));
#70950=CARTESIAN_POINT('Ctrl Pts',(1.54071990404,-36.5742356128,-10.1113057482));
#70951=CARTESIAN_POINT('Ctrl Pts',(1.54071964237,-36.4799878332,-10.1113057849));
#70952=CARTESIAN_POINT('Ctrl Pts',(1.53549875184,-36.3857400535,-10.0746647498));
#70953=CARTESIAN_POINT('Ctrl Pts',(1.52499081167,-36.3112466292,-10.0009159536));
#70954=CARTESIAN_POINT('Ctrl Pts',(1.51169650293,-36.2742356128,-9.90761024282));
#70955=CARTESIAN_POINT('Ctrl Pts',(1.49840229593,-36.2742356128,-9.81430451786));
#70956=CARTESIAN_POINT('Ctrl Pts',(1.38699270387,-36.5742356128,-10.132835726));
#70957=CARTESIAN_POINT('Ctrl Pts',(1.38699270126,-36.4799878332,-10.1328357264));
#70958=CARTESIAN_POINT('Ctrl Pts',(1.38185929484,-36.3857400536,-10.0961824389));
#70959=CARTESIAN_POINT('Ctrl Pts',(1.37152710348,-36.3112466293,-10.0224090285));
#70960=CARTESIAN_POINT('Ctrl Pts',(1.35845499699,-36.2742356128,-9.92907219764));
#70961=CARTESIAN_POINT('Ctrl Pts',(1.34538289151,-36.2742356128,-9.83573536665));
#70962=CARTESIAN_POINT('',(11.0450673741,-36.5742356128,0.800650704934));
#70963=CARTESIAN_POINT('Origin',(10.7507791129301,-36.5721142936209,0.754540830736387));
#70964=CARTESIAN_POINT('Ctrl Pts',(11.0450673741,-36.5742356128,0.800650704934));
#70965=CARTESIAN_POINT('Ctrl Pts',(11.0585597994,-36.5742356128,0.714566551433));
#70966=CARTESIAN_POINT('Ctrl Pts',(11.0714556362,-36.5742356128,0.628315856355));
#70967=CARTESIAN_POINT('Ctrl Pts',(11.0837537732,-36.5742356128,0.541839826087));
#70968=CARTESIAN_POINT('Ctrl Pts',(11.1309935407,-36.5742356128,0.191196052993));
#70969=CARTESIAN_POINT('Ctrl Pts',(11.1677658434,-36.5742356128,-0.163547364245));
#70970=CARTESIAN_POINT('Ctrl Pts',(11.1889875368,-36.5742356128,-0.434883867498));
#70971=CARTESIAN_POINT('Ctrl Pts',(11.2336540706,-36.5742356128,-1.36618233638));
#70972=CARTESIAN_POINT('Ctrl Pts',(11.1622899815,-36.5742356128,-2.31636115629));
#70973=CARTESIAN_POINT('Ctrl Pts',(11.0291793988,-36.5742356128,-2.98459593105));
#70974=CARTESIAN_POINT('Ctrl Pts',(10.6524574839,-36.5742356128,-4.03375119457));
#70975=CARTESIAN_POINT('Ctrl Pts',(10.0721843915,-36.5742356128,-4.97806710985));
#70976=CARTESIAN_POINT('Ctrl Pts',(9.82149842762,-36.5742356128,-5.32595482066));
#70977=CARTESIAN_POINT('Ctrl Pts',(9.23922565917,-36.5742356128,-6.0447166144));
#70978=CARTESIAN_POINT('Ctrl Pts',(8.58741395086,-36.5742356128,-6.69445002697));
#70979=CARTESIAN_POINT('Ctrl Pts',(8.21985964708,-36.5742356128,-7.02884209136));
#70980=CARTESIAN_POINT('Ctrl Pts',(7.71835943349,-36.5742356128,-7.44951290201));
#70981=CARTESIAN_POINT('Ctrl Pts',(7.20312714754,-36.5742356128,-7.83561707229));
#70982=CARTESIAN_POINT('Ctrl Pts',(7.07391925378,-36.5742356128,-7.92965998368));
#70983=CARTESIAN_POINT('Ctrl Pts',(6.68293897532,-36.5742356128,-8.20578167079));
#70984=CARTESIAN_POINT('Ctrl Pts',(6.28153293634,-36.5742356128,-8.46325996647));
#70985=CARTESIAN_POINT('Ctrl Pts',(6.00853446953,-36.5742356128,-8.62630121911));
#70986=CARTESIAN_POINT('Ctrl Pts',(5.45178039508,-36.5742356128,-8.93423446359));
#70987=CARTESIAN_POINT('Ctrl Pts',(4.87486658279,-36.5742356128,-9.2037781865));
#70988=CARTESIAN_POINT('Ctrl Pts',(4.58136980215,-36.5742356128,-9.32859973652));
#70989=CARTESIAN_POINT('Ctrl Pts',(4.06616678437,-36.5742356128,-9.52655591089));
#70990=CARTESIAN_POINT('Ctrl Pts',(3.53901439179,-36.5742356128,-9.69332241165));
#70991=CARTESIAN_POINT('Ctrl Pts',(3.31446912359,-36.5742356128,-9.75814914821));
#70992=CARTESIAN_POINT('Ctrl Pts',(3.01253146546,-36.5742356128,-9.83720045464));
#70993=CARTESIAN_POINT('Ctrl Pts',(2.70802102447,-36.5742356128,-9.90641220657));
#70994=CARTESIAN_POINT('Ctrl Pts',(2.63158870596,-36.5742356128,-9.92313477939));
#70995=CARTESIAN_POINT('Ctrl Pts',(2.47861794588,-36.5742356128,-9.95531796777));
#70996=CARTESIAN_POINT('Ctrl Pts',(2.32512404468,-36.5742356128,-9.98507083709));
#70997=CARTESIAN_POINT('Ctrl Pts',(2.24744160945,-36.5742356128,-9.99950190736));
#70998=CARTESIAN_POINT('Ctrl Pts',(2.04726851031,-36.5742356128,-10.0350233698));
#70999=CARTESIAN_POINT('Ctrl Pts',(1.83768542134,-36.5742356128,-10.0680136806));
#71000=CARTESIAN_POINT('Ctrl Pts',(1.68405004863,-36.5742356128,-10.0907690318));
#71001=CARTESIAN_POINT('Ctrl Pts',(1.54048434157,-36.5742356128,-10.1113387667));
#71002=CARTESIAN_POINT('Ctrl Pts',(1.38699292008,-36.5742356128,-10.1328356959));
#71003=CARTESIAN_POINT('Ctrl Pts',(1.3453969549,-38.2742356128,-9.83573340734));
#71004=CARTESIAN_POINT('Ctrl Pts',(1.35846896198,-38.2742356128,-9.92907025215));
#71005=CARTESIAN_POINT('Ctrl Pts',(1.37154096907,-38.2372245963,-10.022407097));
#71006=CARTESIAN_POINT('Ctrl Pts',(1.38187308059,-38.1627311721,-10.0961805186));
#71007=CARTESIAN_POINT('Ctrl Pts',(1.38700644577,-38.0684833924,-10.1328338118));
#71008=CARTESIAN_POINT('Ctrl Pts',(1.38700644577,-37.9742356128,-10.1328338118));
#71009=CARTESIAN_POINT('Ctrl Pts',(1.48744214824,-38.2742356128,-9.81583956161));
#71010=CARTESIAN_POINT('Ctrl Pts',(1.50072194506,-38.2742356128,-9.9091473051));
#71011=CARTESIAN_POINT('Ctrl Pts',(1.51400174188,-38.2372245963,-10.0024550486));
#71012=CARTESIAN_POINT('Ctrl Pts',(1.52449808981,-38.1627311721,-10.0762054686));
#71013=CARTESIAN_POINT('Ctrl Pts',(1.52971305438,-38.0684833924,-10.1128473337));
#71014=CARTESIAN_POINT('Ctrl Pts',(1.52971305438,-37.9742356128,-10.1128473337));
#71015=CARTESIAN_POINT('Ctrl Pts',(1.62218880952,-38.2742356128,-9.79656548787));
#71016=CARTESIAN_POINT('Ctrl Pts',(1.63581885953,-38.2742356128,-9.88982281252));
#71017=CARTESIAN_POINT('Ctrl Pts',(1.64944890954,-38.2372245963,-9.98308013716));
#71018=CARTESIAN_POINT('Ctrl Pts',(1.66022209833,-38.1627311721,-10.056790706));
#71019=CARTESIAN_POINT('Ctrl Pts',(1.66557460619,-38.0684833924,-10.0934127718));
#71020=CARTESIAN_POINT('Ctrl Pts',(1.66557460619,-37.9742356128,-10.0934127718));
#71021=CARTESIAN_POINT('Ctrl Pts',(1.76414135208,-38.2742356128,-9.77563578571));
#71022=CARTESIAN_POINT('Ctrl Pts',(1.77805006872,-38.2742356128,-9.86885473404));
#71023=CARTESIAN_POINT('Ctrl Pts',(1.79195878537,-38.2372245963,-9.96207368237));
#71024=CARTESIAN_POINT('Ctrl Pts',(1.80295222999,-38.1627311721,-10.0357539189));
#71025=CARTESIAN_POINT('Ctrl Pts',(1.8084141722,-38.0684833924,-10.072360914));
#71026=CARTESIAN_POINT('Ctrl Pts',(1.8084141722,-37.9742356128,-10.072360914));
#71027=CARTESIAN_POINT('Ctrl Pts',(1.99446361947,-38.2742356128,-9.73983610905));
#71028=CARTESIAN_POINT('Ctrl Pts',(2.00973240206,-38.2742356128,-9.83284844843));
#71029=CARTESIAN_POINT('Ctrl Pts',(2.02500118465,-38.2372245963,-9.92586078781));
#71030=CARTESIAN_POINT('Ctrl Pts',(2.03706962731,-38.1627311721,-9.99937772036));
#71031=CARTESIAN_POINT('Ctrl Pts',(2.04306566395,-38.0684833924,-10.0359035807));
#71032=CARTESIAN_POINT('Ctrl Pts',(2.04306566395,-37.9742356128,-10.0359035807));
#71033=CARTESIAN_POINT('Ctrl Pts',(2.20684905707,-38.2742356128,-9.70218717363));
#71034=CARTESIAN_POINT('Ctrl Pts',(2.22389967294,-38.2742356128,-9.79488512123));
#71035=CARTESIAN_POINT('Ctrl Pts',(2.2409502888,-38.2372245963,-9.88758306883));
#71036=CARTESIAN_POINT('Ctrl Pts',(2.25442709278,-38.1627311721,-9.96085150608));
#71037=CARTESIAN_POINT('Ctrl Pts',(2.26112285302,-38.0684833924,-9.99725390513));
#71038=CARTESIAN_POINT('Ctrl Pts',(2.26112285302,-37.9742356128,-9.99725390513));
#71039=CARTESIAN_POINT('Ctrl Pts',(2.30711395977,-38.2742356128,-9.6833625585));
#71040=CARTESIAN_POINT('Ctrl Pts',(2.32490006217,-38.2742356128,-9.77592170898));
#71041=CARTESIAN_POINT('Ctrl Pts',(2.34268616457,-38.2372245963,-9.86848085947));
#71042=CARTESIAN_POINT('Ctrl Pts',(2.35674429625,-38.1627311721,-9.94163959163));
#71043=CARTESIAN_POINT('Ctrl Pts',(2.36372888208,-38.0684833924,-9.97798748507));
#71044=CARTESIAN_POINT('Ctrl Pts',(2.36372888208,-37.9742356128,-9.97798748507));
#71045=CARTESIAN_POINT('Ctrl Pts',(2.62538537067,-38.2742356128,-9.62013145829));
#71046=CARTESIAN_POINT('Ctrl Pts',(2.64567868831,-38.2742356128,-9.71219319788));
#71047=CARTESIAN_POINT('Ctrl Pts',(2.66597200595,-38.2372245963,-9.80425493747));
#71048=CARTESIAN_POINT('Ctrl Pts',(2.68201183923,-38.1627311721,-9.87702051628));
#71049=CARTESIAN_POINT('Ctrl Pts',(2.68998100695,-38.0684833924,-9.9131730768));
#71050=CARTESIAN_POINT('Ctrl Pts',(2.68998100695,-37.9742356128,-9.9131730768));
#71051=CARTESIAN_POINT('Ctrl Pts',(2.94353985871,-38.2742356128,-9.54564367384));
#71052=CARTESIAN_POINT('Ctrl Pts',(2.96637211727,-38.2742356128,-9.63711021518));
#71053=CARTESIAN_POINT('Ctrl Pts',(2.98920437583,-38.2372245963,-9.72857675651));
#71054=CARTESIAN_POINT('Ctrl Pts',(3.00725098901,-38.1627311721,-9.80087189053));
#71055=CARTESIAN_POINT('Ctrl Pts',(3.01621719496,-38.0684833924,-9.83679071747));
#71056=CARTESIAN_POINT('Ctrl Pts',(3.01621719496,-37.9742356128,-9.83679071747));
#71057=CARTESIAN_POINT('Ctrl Pts',(3.1599790764,-38.2742356128,-9.48926500243));
#71058=CARTESIAN_POINT('Ctrl Pts',(3.18460764997,-38.2742356128,-9.58026655999));
#71059=CARTESIAN_POINT('Ctrl Pts',(3.20923622353,-38.2372245963,-9.67126811755));
#71060=CARTESIAN_POINT('Ctrl Pts',(3.22870264265,-38.1627311721,-9.74319572864));
#71061=CARTESIAN_POINT('Ctrl Pts',(3.23837426089,-38.0684833924,-9.77893195672));
#71062=CARTESIAN_POINT('Ctrl Pts',(3.23837426089,-37.9742356128,-9.77893195672));
#71063=CARTESIAN_POINT('Ctrl Pts',(3.8074159761,-38.2742356128,-9.30368354848));
#71064=CARTESIAN_POINT('Ctrl Pts',(3.83743195198,-38.2742356128,-9.39314222695));
#71065=CARTESIAN_POINT('Ctrl Pts',(3.86744792787,-38.2372245963,-9.48260090542));
#71066=CARTESIAN_POINT('Ctrl Pts',(3.89117254863,-38.1627311721,-9.55330902521));
#71067=CARTESIAN_POINT('Ctrl Pts',(3.90295979477,-38.0684833924,-9.5884393661));
#71068=CARTESIAN_POINT('Ctrl Pts',(3.90295979477,-37.9742356128,-9.5884393661));
#71069=CARTESIAN_POINT('Ctrl Pts',(4.43772493193,-38.2742356128,-9.0706422086));
#71070=CARTESIAN_POINT('Ctrl Pts',(4.4731429426,-38.2742356128,-9.15810966487));
#71071=CARTESIAN_POINT('Ctrl Pts',(4.50856095327,-38.2372245963,-9.24557712114));
#71072=CARTESIAN_POINT('Ctrl Pts',(4.53655534108,-38.1627311721,-9.31471137936));
#71073=CARTESIAN_POINT('Ctrl Pts',(4.55046396139,-38.0684833924,-9.3490597691));
#71074=CARTESIAN_POINT('Ctrl Pts',(4.55046396139,-37.9742356128,-9.3490597691));
#71075=CARTESIAN_POINT('Ctrl Pts',(4.84930849374,-38.2742356128,-8.89395004026));
#71076=CARTESIAN_POINT('Ctrl Pts',(4.88828590441,-38.2742356128,-8.97987882553));
#71077=CARTESIAN_POINT('Ctrl Pts',(4.92726331508,-38.2372245963,-9.0658076108));
#71078=CARTESIAN_POINT('Ctrl Pts',(4.95807105191,-38.1627311721,-9.13372570379));
#71079=CARTESIAN_POINT('Ctrl Pts',(4.97337744528,-38.0684833924,-9.16746985886));
#71080=CARTESIAN_POINT('Ctrl Pts',(4.97337744528,-37.9742356128,-9.16746985886));
#71081=CARTESIAN_POINT('Ctrl Pts',(5.85544401236,-38.2742356128,-8.40100946237));
#71082=CARTESIAN_POINT('Ctrl Pts',(5.90280719326,-38.2742356128,-8.48282686114));
#71083=CARTESIAN_POINT('Ctrl Pts',(5.95017037416,-38.2372245963,-8.56464425991));
#71084=CARTESIAN_POINT('Ctrl Pts',(5.98760622193,-38.1627311721,-8.62931271392));
#71085=CARTESIAN_POINT('Ctrl Pts',(6.00620569958,-38.0684833924,-8.66144233128));
#71086=CARTESIAN_POINT('Ctrl Pts',(6.00620569958,-37.9742356128,-8.66144233128));
#71087=CARTESIAN_POINT('Ctrl Pts',(6.79666807074,-38.2742356128,-7.78925125486));
#71088=CARTESIAN_POINT('Ctrl Pts',(6.85133327952,-38.2742356128,-7.86627345027));
#71089=CARTESIAN_POINT('Ctrl Pts',(6.9059984883,-38.2372245963,-7.94329564567));
#71090=CARTESIAN_POINT('Ctrl Pts',(6.94920585732,-38.1627311721,-8.00417397196));
#71091=CARTESIAN_POINT('Ctrl Pts',(6.97067283459,-38.0684833924,-8.03442051739));
#71092=CARTESIAN_POINT('Ctrl Pts',(6.97067283459,-37.9742356128,-8.03442051739));
#71093=CARTESIAN_POINT('Ctrl Pts',(7.33820201297,-38.2742356128,-7.38433102414));
#71094=CARTESIAN_POINT('Ctrl Pts',(7.39620233991,-38.2742356128,-7.45876186455));
#71095=CARTESIAN_POINT('Ctrl Pts',(7.45420266686,-38.2372245963,-7.53319270496));
#71096=CARTESIAN_POINT('Ctrl Pts',(7.50004611258,-38.1627311721,-7.5920228247));
#71097=CARTESIAN_POINT('Ctrl Pts',(7.52282278764,-38.0684833924,-7.62125174753));
#71098=CARTESIAN_POINT('Ctrl Pts',(7.52282278764,-37.9742356128,-7.62125174753));
#71099=CARTESIAN_POINT('Ctrl Pts',(8.10467751429,-38.2742356128,-6.74809011842));
#71100=CARTESIAN_POINT('Ctrl Pts',(8.16739900498,-38.2742356128,-6.81870393688));
#71101=CARTESIAN_POINT('Ctrl Pts',(8.23012049567,-38.2372245963,-6.88931775534));
#71102=CARTESIAN_POINT('Ctrl Pts',(8.27969554811,-38.1627311721,-6.94513090196));
#71103=CARTESIAN_POINT('Ctrl Pts',(8.30432621991,-38.0684833924,-6.9728608836));
#71104=CARTESIAN_POINT('Ctrl Pts',(8.30432621991,-37.9742356128,-6.9728608836));
#71105=CARTESIAN_POINT('Ctrl Pts',(8.80837603922,-38.2742356128,-6.03968780603));
#71106=CARTESIAN_POINT('Ctrl Pts',(8.87649577319,-38.2742356128,-6.10488334472));
#71107=CARTESIAN_POINT('Ctrl Pts',(8.94461550716,-38.2372245963,-6.17007888341));
#71108=CARTESIAN_POINT('Ctrl Pts',(8.9984573299,-38.1627311721,-6.22160942286));
#71109=CARTESIAN_POINT('Ctrl Pts',(9.02520788688,-38.0684833924,-6.24721165103));
#71110=CARTESIAN_POINT('Ctrl Pts',(9.02520788688,-37.9742356128,-6.24721165103));
#71111=CARTESIAN_POINT('Ctrl Pts',(9.01511576881,-38.2742356128,-5.81836032423));
#71112=CARTESIAN_POINT('Ctrl Pts',(9.08496935084,-38.2742356128,-5.88172164813));
#71113=CARTESIAN_POINT('Ctrl Pts',(9.15482293286,-38.2372245963,-5.94508297203));
#71114=CARTESIAN_POINT('Ctrl Pts',(9.21003518872,-38.1627311721,-5.9951637485));
#71115=CARTESIAN_POINT('Ctrl Pts',(9.23746662625,-38.0684833924,-6.02004568222));
#71116=CARTESIAN_POINT('Ctrl Pts',(9.23746662625,-37.9742356128,-6.02004568222));
#71117=CARTESIAN_POINT('Ctrl Pts',(9.57792489155,-38.2742356128,-5.17020745095));
#71118=CARTESIAN_POINT('Ctrl Pts',(9.65303226325,-38.2742356128,-5.22756135993));
#71119=CARTESIAN_POINT('Ctrl Pts',(9.72813963496,-38.2372245963,-5.28491526891));
#71120=CARTESIAN_POINT('Ctrl Pts',(9.78750448504,-38.1627311721,-5.33024778594));
#71121=CARTESIAN_POINT('Ctrl Pts',(9.81699908093,-38.0684833924,-5.35277061336));
#71122=CARTESIAN_POINT('Ctrl Pts',(9.81699908093,-37.9742356128,-5.35277061336));
#71123=CARTESIAN_POINT('Ctrl Pts',(10.0628691567,-38.2742356128,-4.45793107296));
#71124=CARTESIAN_POINT('Ctrl Pts',(10.1440778097,-38.2742356128,-4.50658435893));
#71125=CARTESIAN_POINT('Ctrl Pts',(10.2252864627,-38.2372245963,-4.55523764491));
#71126=CARTESIAN_POINT('Ctrl Pts',(10.2894737642,-38.1627311721,-4.59369319157));
#71127=CARTESIAN_POINT('Ctrl Pts',(10.3213643277,-38.0684833924,-4.61279929216));
#71128=CARTESIAN_POINT('Ctrl Pts',(10.3213643277,-37.9742356128,-4.61279929216));
#71129=CARTESIAN_POINT('Ctrl Pts',(10.3284955409,-38.2742356128,-3.96990195467));
#71130=CARTESIAN_POINT('Ctrl Pts',(10.4140079048,-38.2742356128,-4.01100462119));
#71131=CARTESIAN_POINT('Ctrl Pts',(10.4995202688,-38.2372245963,-4.05210728771));
#71132=CARTESIAN_POINT('Ctrl Pts',(10.567109215,-38.1627311721,-4.08459477936));
#71133=CARTESIAN_POINT('Ctrl Pts',(10.6006898492,-38.0684833924,-4.10073580569));
#71134=CARTESIAN_POINT('Ctrl Pts',(10.6006898492,-37.9742356128,-4.10073580569));
#71135=CARTESIAN_POINT('Ctrl Pts',(10.8077466192,-38.2742356128,-2.75452466443));
#71136=CARTESIAN_POINT('Ctrl Pts',(10.9008597457,-38.2742356128,-2.77619835249));
#71137=CARTESIAN_POINT('Ctrl Pts',(10.9939728721,-38.2372245963,-2.79787204055));
#71138=CARTESIAN_POINT('Ctrl Pts',(11.0675694769,-38.1627311721,-2.81500298289));
#71139=CARTESIAN_POINT('Ctrl Pts',(11.104134906,-38.0684833924,-2.82351415623));
#71140=CARTESIAN_POINT('Ctrl Pts',(11.104134906,-37.9742356128,-2.82351415623));
#71141=CARTESIAN_POINT('Ctrl Pts',(10.9568356572,-38.2742356128,-1.46082431358));
#71142=CARTESIAN_POINT('Ctrl Pts',(11.0519582595,-38.2742356128,-1.46349516331));
#71143=CARTESIAN_POINT('Ctrl Pts',(11.1470808617,-38.2372245963,-1.46616601304));
#71144=CARTESIAN_POINT('Ctrl Pts',(11.2222657318,-38.1627311721,-1.46827696463));
#71145=CARTESIAN_POINT('Ctrl Pts',(11.2596203042,-38.0684833924,-1.46932589231));
#71146=CARTESIAN_POINT('Ctrl Pts',(11.2596203042,-37.9742356128,-1.46932589231));
#71147=CARTESIAN_POINT('Ctrl Pts',(10.9320266615,-38.2742356128,-0.702352458466));
#71148=CARTESIAN_POINT('Ctrl Pts',(11.0262542838,-38.2742356128,-0.696917360674));
#71149=CARTESIAN_POINT('Ctrl Pts',(11.1204819061,-38.2372245963,-0.691482262882));
#71150=CARTESIAN_POINT('Ctrl Pts',(11.1949594534,-38.1627311721,-0.68718671173));
#71151=CARTESIAN_POINT('Ctrl Pts',(11.2319624987,-38.0684833924,-0.68505200487));
#71152=CARTESIAN_POINT('Ctrl Pts',(11.2319624987,-37.9742356128,-0.68505200487));
#71153=CARTESIAN_POINT('Ctrl Pts',(10.861915737,-38.2742356128,0.0317722973303));
#71154=CARTESIAN_POINT('Ctrl Pts',(10.9557329316,-38.2742356128,0.041860744283));
#71155=CARTESIAN_POINT('Ctrl Pts',(11.0495501263,-38.2372245963,0.0519491912357));
#71156=CARTESIAN_POINT('Ctrl Pts',(11.1237031794,-38.1627311721,0.0599233301614));
#71157=CARTESIAN_POINT('Ctrl Pts',(11.1605451425,-38.0684833924,0.0638848213432));
#71158=CARTESIAN_POINT('Ctrl Pts',(11.1605451425,-37.9742356128,0.0638848213432));
#71159=CARTESIAN_POINT('Ctrl Pts',(10.7486857138,-38.2742356128,0.754197377643));
#71160=CARTESIAN_POINT('Ctrl Pts',(10.8417967511,-38.2742356128,0.768791167183));
#71161=CARTESIAN_POINT('Ctrl Pts',(10.9349077884,-38.2372245963,0.783384956722));
#71162=CARTESIAN_POINT('Ctrl Pts',(11.0085027318,-38.1627311721,0.794919884766));
#71163=CARTESIAN_POINT('Ctrl Pts',(11.0450673507,-38.0684833924,0.800650852517));
#71164=CARTESIAN_POINT('Ctrl Pts',(11.0450673507,-37.9742356128,0.800650852517));
#71165=CARTESIAN_POINT('',(11.0450673664881,-37.9742356128,0.800650755926446));
#71166=CARTESIAN_POINT('Origin',(10.7507817353365,-37.9763569060012,0.754523858996911));
#71167=CARTESIAN_POINT('Ctrl Pts',(11.045067373838,-37.9742356128,0.800650704892936));
#71168=CARTESIAN_POINT('Ctrl Pts',(11.0576661427342,-37.9742356128,0.720268620987917));
#71169=CARTESIAN_POINT('Ctrl Pts',(11.0696392766439,-37.9742356128,0.639700888506689));
#71170=CARTESIAN_POINT('Ctrl Pts',(11.0809742041238,-37.9742356128,0.558892739368612));
#71171=CARTESIAN_POINT('Ctrl Pts',(11.0875830790094,-37.9742356128,0.511777224220254));
#71172=CARTESIAN_POINT('Ctrl Pts',(11.093974504389,-37.9742356128,0.464580392649293));
#71173=CARTESIAN_POINT('Ctrl Pts',(11.1001422093536,-37.9742356128,0.417294686478159));
#71174=CARTESIAN_POINT('Ctrl Pts',(11.1055449723429,-37.9742356128,0.375873531496338));
#71175=CARTESIAN_POINT('Ctrl Pts',(11.1107759171709,-37.9742356128,0.334385408520878));
#71176=CARTESIAN_POINT('Ctrl Pts',(11.1158312696378,-37.9742356128,0.292809025903721));
#71177=CARTESIAN_POINT('Ctrl Pts',(11.1278544247113,-37.9742356128,0.19392783040354));
#71178=CARTESIAN_POINT('Ctrl Pts',(11.1388834873982,-37.9742356128,0.0945699250618215));
#71179=CARTESIAN_POINT('Ctrl Pts',(11.1488040792331,-37.9742356128,-0.00525704534534066));
#71180=CARTESIAN_POINT('Ctrl Pts',(11.1592276051179,-37.9742356128,-0.110144841089314));
#71181=CARTESIAN_POINT('Ctrl Pts',(11.1684269371819,-37.9742356128,-0.21555045358533));
#71182=CARTESIAN_POINT('Ctrl Pts',(11.1762317393997,-37.9742356128,-0.321420936240089));
#71183=CARTESIAN_POINT('Ctrl Pts',(11.1846838595737,-37.9742356128,-0.436072149340684));
#71184=CARTESIAN_POINT('Ctrl Pts',(11.1914997918907,-37.9742356128,-0.551268619946787));
#71185=CARTESIAN_POINT('Ctrl Pts',(11.1964295589341,-37.9742356128,-0.666891713681186));
#71186=CARTESIAN_POINT('Ctrl Pts',(11.1994520258282,-37.9742356128,-0.737780859136654));
#71187=CARTESIAN_POINT('Ctrl Pts',(11.2017648735253,-37.9742356128,-0.808829359655462));
#71188=CARTESIAN_POINT('Ctrl Pts',(11.2033071963304,-37.9742356128,-0.880001550581649));
#71189=CARTESIAN_POINT('Ctrl Pts',(11.2048492854098,-37.9742356128,-0.951162955976867));
#71190=CARTESIAN_POINT('Ctrl Pts',(11.2056211223806,-37.9742356128,-1.02244172630779));
#71191=CARTESIAN_POINT('Ctrl Pts',(11.2055609332167,-37.9742356128,-1.09383517988263));
#71192=CARTESIAN_POINT('Ctrl Pts',(11.2054459298545,-37.9742356128,-1.23024656479139));
#71193=CARTESIAN_POINT('Ctrl Pts',(11.2022909838307,-37.9742356128,-1.36706187880045));
#71194=CARTESIAN_POINT('Ctrl Pts',(11.1956647789511,-37.9742356128,-1.50402455513197));
#71195=CARTESIAN_POINT('Ctrl Pts',(11.1895754817146,-37.9742356128,-1.62988942976902));
#71196=CARTESIAN_POINT('Ctrl Pts',(11.1805531072994,-37.9742356128,-1.75587729149789));
#71197=CARTESIAN_POINT('Ctrl Pts',(11.1682938698613,-37.9742356128,-1.88176142786058));
#71198=CARTESIAN_POINT('Ctrl Pts',(11.1571777445444,-37.9742356128,-1.99590750279133));
#71199=CARTESIAN_POINT('Ctrl Pts',(11.1433996715383,-37.9742356128,-2.10996747829517));
#71200=CARTESIAN_POINT('Ctrl Pts',(11.1267731665591,-37.9742356128,-2.22376344203655));
#71201=CARTESIAN_POINT('Ctrl Pts',(11.1110191505116,-37.9742356128,-2.33158787303733));
#71202=CARTESIAN_POINT('Ctrl Pts',(11.092707316135,-37.9742356128,-2.43917480080161));
#71203=CARTESIAN_POINT('Ctrl Pts',(11.0717243336485,-37.9742356128,-2.54637308638286));
#71204=CARTESIAN_POINT('Ctrl Pts',(11.0520129790026,-37.9742356128,-2.64707485391739));
#71205=CARTESIAN_POINT('Ctrl Pts',(11.0299442382527,-37.9742356128,-2.74743336288688));
#71206=CARTESIAN_POINT('Ctrl Pts',(11.0054696943795,-37.9742356128,-2.84732875965493));
#71207=CARTESIAN_POINT('Ctrl Pts',(10.9925223436773,-37.9742356128,-2.90017471838646));
#71208=CARTESIAN_POINT('Ctrl Pts',(10.9789025174646,-37.9742356128,-2.95289119232652));
#71209=CARTESIAN_POINT('Ctrl Pts',(10.9646089566338,-37.9742356128,-3.00546151299019));
#71210=CARTESIAN_POINT('Ctrl Pts',(10.9388145384853,-37.9742356128,-3.10033086356308));
#71211=CARTESIAN_POINT('Ctrl Pts',(10.9108232164818,-37.9742356128,-3.19472254000091));
#71212=CARTESIAN_POINT('Ctrl Pts',(10.88061675586,-37.9742356128,-3.28848712616045));
#71213=CARTESIAN_POINT('Ctrl Pts',(10.8496041039679,-37.9742356128,-3.38475422963813));
#71214=CARTESIAN_POINT('Ctrl Pts',(10.8162567039116,-37.9742356128,-3.48036028663188));
#71215=CARTESIAN_POINT('Ctrl Pts',(10.7806034744716,-37.9742356128,-3.57516864650273));
#71216=CARTESIAN_POINT('Ctrl Pts',(10.7432639703021,-37.9742356128,-3.67446111465515));
#71217=CARTESIAN_POINT('Ctrl Pts',(10.703395501285,-37.9742356128,-3.77287851876867));
#71218=CARTESIAN_POINT('Ctrl Pts',(10.6610814766523,-37.9742356128,-3.87029239545888));
#71219=CARTESIAN_POINT('Ctrl Pts',(10.6187243454886,-37.9742356128,-3.96780551050643));
#71220=CARTESIAN_POINT('Ctrl Pts',(10.5739172222098,-37.9742356128,-4.06431314334558));
#71221=CARTESIAN_POINT('Ctrl Pts',(10.5267870850518,-37.9742356128,-4.15971429500487));
#71222=CARTESIAN_POINT('Ctrl Pts',(10.4878597234772,-37.9742356128,-4.23851133123732));
#71223=CARTESIAN_POINT('Ctrl Pts',(10.4473483600161,-37.9742356128,-4.316554711738));
#71224=CARTESIAN_POINT('Ctrl Pts',(10.4053370662145,-37.9742356128,-4.39381058626197));
#71225=CARTESIAN_POINT('Ctrl Pts',(10.3474952495324,-37.9742356128,-4.50017770156528));
#71226=CARTESIAN_POINT('Ctrl Pts',(10.2868118157629,-37.9742356128,-4.60504448980234));
#71227=CARTESIAN_POINT('Ctrl Pts',(10.2235623322584,-37.9742356128,-4.7083274604292));
#71228=CARTESIAN_POINT('Ctrl Pts',(10.1574136573687,-37.9742356128,-4.81634465309378));
#71229=CARTESIAN_POINT('Ctrl Pts',(10.0884593000215,-37.9742356128,-4.9226293675133));
#71230=CARTESIAN_POINT('Ctrl Pts',(10.0170520252819,-37.9742356128,-5.02713305669034));
#71231=CARTESIAN_POINT('Ctrl Pts',(9.94157132886643,-37.9742356128,-5.1375981495793));
#71232=CARTESIAN_POINT('Ctrl Pts',(9.86335135573855,-37.9742356128,-5.24607301541748));
#71233=CARTESIAN_POINT('Ctrl Pts',(9.78283033969483,-37.9742356128,-5.35255452647816));
#71234=CARTESIAN_POINT('Ctrl Pts',(9.73480989402804,-37.9742356128,-5.41605707360986));
#71235=CARTESIAN_POINT('Ctrl Pts',(9.68597136550832,-37.9742356128,-5.47885171054048));
#71236=CARTESIAN_POINT('Ctrl Pts',(9.6364074829053,-37.9742356128,-5.54094653469057));
#71237=CARTESIAN_POINT('Ctrl Pts',(9.55705149948688,-37.9742356128,-5.64036561925043));
#71238=CARTESIAN_POINT('Ctrl Pts',(9.47583217163434,-37.9742356128,-5.73799546041952));
#71239=CARTESIAN_POINT('Ctrl Pts',(9.39295246670258,-37.9742356128,-5.83397638243802));
#71240=CARTESIAN_POINT('Ctrl Pts',(9.34842440213017,-37.9742356128,-5.88554322497057));
#71241=CARTESIAN_POINT('Ctrl Pts',(9.30341933348068,-37.9742356128,-5.93663173824686));
#71242=CARTESIAN_POINT('Ctrl Pts',(9.25796679639709,-37.9742356128,-5.98726452990667));
#71243=CARTESIAN_POINT('Ctrl Pts',(9.16705589418052,-37.9742356128,-6.08853660550218));
#71244=CARTESIAN_POINT('Ctrl Pts',(9.0743387174743,-37.9742356128,-6.1880080646955));
#71245=CARTESIAN_POINT('Ctrl Pts',(8.98008824482996,-37.9742356128,-6.28577047569799));
#71246=CARTESIAN_POINT('Ctrl Pts',(8.90029866668485,-37.9742356128,-6.36853315384152));
#71247=CARTESIAN_POINT('Ctrl Pts',(8.8194114197026,-37.9742356128,-6.45007008726216));
#71248=CARTESIAN_POINT('Ctrl Pts',(8.73756131692268,-37.9742356128,-6.53041646823511));
#71249=CARTESIAN_POINT('Ctrl Pts',(8.68636996822059,-37.9742356128,-6.58066734716676));
#71250=CARTESIAN_POINT('Ctrl Pts',(8.63480131053765,-37.9742356128,-6.63045217403649));
#71251=CARTESIAN_POINT('Ctrl Pts',(8.58287807592455,-37.9742356128,-6.67977647996842));
#71252=CARTESIAN_POINT('Ctrl Pts',(8.50456388436919,-37.9742356128,-6.75417078864104));
#71253=CARTESIAN_POINT('Ctrl Pts',(8.42544574969429,-37.9742356128,-6.82751663928241));
#71254=CARTESIAN_POINT('Ctrl Pts',(8.34567252955157,-37.9742356128,-6.8997996171541));
#71255=CARTESIAN_POINT('Ctrl Pts',(8.26266734472803,-37.9742356128,-6.97501109698531));
#71256=CARTESIAN_POINT('Ctrl Pts',(8.17895266977429,-37.9742356128,-7.04907193014341));
#71257=CARTESIAN_POINT('Ctrl Pts',(8.09463951602057,-37.9742356128,-7.12197066509028));
#71258=CARTESIAN_POINT('Ctrl Pts',(8.0029222082522,-37.9742356128,-7.20127117054375));
#71259=CARTESIAN_POINT('Ctrl Pts',(7.91049666065247,-37.9742356128,-7.27919663775101));
#71260=CARTESIAN_POINT('Ctrl Pts',(7.81744159254399,-37.9742356128,-7.35573617280705));
#71261=CARTESIAN_POINT('Ctrl Pts',(7.71969237318238,-37.9742356128,-7.43613673512038));
#71262=CARTESIAN_POINT('Ctrl Pts',(7.62124779569011,-37.9742356128,-7.5150082397789));
#71263=CARTESIAN_POINT('Ctrl Pts',(7.52213761733522,-37.9742356128,-7.59233927662337));
#71264=CARTESIAN_POINT('Ctrl Pts',(7.48114563527072,-37.9742356128,-7.62432340305695));
#71265=CARTESIAN_POINT('Ctrl Pts',(7.44003642245277,-37.9742356128,-7.65604603818923));
#71266=CARTESIAN_POINT('Ctrl Pts',(7.39882688005116,-37.9742356128,-7.68749334749781));
#71267=CARTESIAN_POINT('Ctrl Pts',(7.28758125498532,-37.9742356128,-7.77238571409046));
#71268=CARTESIAN_POINT('Ctrl Pts',(7.17557863982231,-37.9742356128,-7.85529688978051));
#71269=CARTESIAN_POINT('Ctrl Pts',(7.06265199352647,-37.9742356128,-7.93630090391787));
#71270=CARTESIAN_POINT('Ctrl Pts',(6.98391249723267,-37.9742356128,-7.99278195139573));
#71271=CARTESIAN_POINT('Ctrl Pts',(6.90472242863274,-37.9742356128,-8.04833530896636));
#71272=CARTESIAN_POINT('Ctrl Pts',(6.82501533972286,-37.9742356128,-8.10297764790911));
#71273=CARTESIAN_POINT('Ctrl Pts',(6.68910314957339,-37.9742356128,-8.19615079050117));
#71274=CARTESIAN_POINT('Ctrl Pts',(6.55169566021097,-37.9742356128,-8.28666925523598));
#71275=CARTESIAN_POINT('Ctrl Pts',(6.41265719431847,-37.9742356128,-8.37444381217628));
#71276=CARTESIAN_POINT('Ctrl Pts',(6.3053066284567,-37.9742356128,-8.44221389504739));
#71277=CARTESIAN_POINT('Ctrl Pts',(6.19698246692728,-37.9742356128,-8.50834800082493));
#71278=CARTESIAN_POINT('Ctrl Pts',(6.08764898154051,-37.9742356128,-8.57278393309764));
#71279=CARTESIAN_POINT('Ctrl Pts',(5.98836838379676,-37.9742356128,-8.63129517372608));
#71280=CARTESIAN_POINT('Ctrl Pts',(5.88825509703659,-37.9742356128,-8.68840608318665));
#71281=CARTESIAN_POINT('Ctrl Pts',(5.7873158382133,-37.9742356128,-8.74405315587561));
#71282=CARTESIAN_POINT('Ctrl Pts',(5.62003536011473,-37.9742356128,-8.83627365593388));
#71283=CARTESIAN_POINT('Ctrl Pts',(5.45049527652575,-37.9742356128,-8.92446710527229));
#71284=CARTESIAN_POINT('Ctrl Pts',(5.27878630562228,-37.9742356128,-9.00845329983273));
#71285=CARTESIAN_POINT('Ctrl Pts',(5.11226631012109,-37.9742356128,-9.08990146568441));
#71286=CARTESIAN_POINT('Ctrl Pts',(4.94370656192245,-37.9742356128,-9.16739135702801));
#71287=CARTESIAN_POINT('Ctrl Pts',(4.77325954530881,-37.9742356128,-9.24076338864954));
#71288=CARTESIAN_POINT('Ctrl Pts',(4.61325613185901,-37.9742356128,-9.30963978053032));
#71289=CARTESIAN_POINT('Ctrl Pts',(4.45159154314567,-37.9742356128,-9.37488596251091));
#71290=CARTESIAN_POINT('Ctrl Pts',(4.28841412642254,-37.9742356128,-9.4364074687214));
#71291=CARTESIAN_POINT('Ctrl Pts',(4.21192131899931,-37.9742356128,-9.46524695411987));
#71292=CARTESIAN_POINT('Ctrl Pts',(4.13509623384778,-37.9742356128,-9.49326864559091));
#71293=CARTESIAN_POINT('Ctrl Pts',(4.0579543036934,-37.9742356128,-9.52046726498404));
#71294=CARTESIAN_POINT('Ctrl Pts',(4.00538316554377,-37.9742356128,-9.53900274075881));
#71295=CARTESIAN_POINT('Ctrl Pts',(3.95266776619419,-37.9742356128,-9.55715511842427));
#71296=CARTESIAN_POINT('Ctrl Pts',(3.89979238982722,-37.9742356128,-9.57493036523837));
#71297=CARTESIAN_POINT('Ctrl Pts',(3.82665212994116,-37.9742356128,-9.59951810835909));
#71298=CARTESIAN_POINT('Ctrl Pts',(3.75321493143739,-37.9742356128,-9.62338071508881));
#71299=CARTESIAN_POINT('Ctrl Pts',(3.67950687086322,-37.9742356128,-9.64651331815322));
#71300=CARTESIAN_POINT('Ctrl Pts',(3.61652703617181,-37.9742356128,-9.66627896529724));
#71301=CARTESIAN_POINT('Ctrl Pts',(3.55335456166025,-37.9742356128,-9.68551083921918));
#71302=CARTESIAN_POINT('Ctrl Pts',(3.49002949975775,-37.9742356128,-9.70420212536654));
#71303=CARTESIAN_POINT('Ctrl Pts',(3.40965967613772,-37.9742356128,-9.72792441360065));
#71304=CARTESIAN_POINT('Ctrl Pts',(3.32904208220192,-37.9742356128,-9.7507761888097));
#71305=CARTESIAN_POINT('Ctrl Pts',(3.2481676520397,-37.9742356128,-9.77276406314082));
#71306=CARTESIAN_POINT('Ctrl Pts',(3.1749308511008,-37.9742356128,-9.79267544393483));
#71307=CARTESIAN_POINT('Ctrl Pts',(3.10147823214554,-37.9742356128,-9.81187941582968));
#71308=CARTESIAN_POINT('Ctrl Pts',(3.02780135377895,-37.9742356128,-9.83038392558351));
#71309=CARTESIAN_POINT('Ctrl Pts',(2.97692025161001,-37.9742356128,-9.84316310233806));
#71310=CARTESIAN_POINT('Ctrl Pts',(2.92593218832356,-37.9742356128,-9.85560874262589));
#71311=CARTESIAN_POINT('Ctrl Pts',(2.87485126513147,-37.9742356128,-9.86772100278545));
#71312=CARTESIAN_POINT('Ctrl Pts',(2.8467281991402,-37.9742356128,-9.874389517575));
#71313=CARTESIAN_POINT('Ctrl Pts',(2.81857376808186,-37.9742356128,-9.88095778691781));
#71314=CARTESIAN_POINT('Ctrl Pts',(2.79038631636844,-37.9742356128,-9.88742682636709));
#71315=CARTESIAN_POINT('Ctrl Pts',(2.73551854970118,-37.9742356128,-9.90001901634839));
#71316=CARTESIAN_POINT('Ctrl Pts',(2.68053097377708,-37.9742356128,-9.91223375160826));
#71317=CARTESIAN_POINT('Ctrl Pts',(2.62549899348512,-37.9742356128,-9.92406002398358));
#71318=CARTESIAN_POINT('Ctrl Pts',(2.60518339835759,-37.9742356128,-9.92842580839057));
#71319=CARTESIAN_POINT('Ctrl Pts',(2.58486223162589,-37.9742356128,-9.93273857235789));
#71320=CARTESIAN_POINT('Ctrl Pts',(2.56454112002745,-37.9742356128,-9.93699744921689));
#71321=CARTESIAN_POINT('Ctrl Pts',(2.54041972653535,-37.9742356128,-9.94205278509517));
#71322=CARTESIAN_POINT('Ctrl Pts',(2.51629397351212,-37.9742356128,-9.94703300268813));
#71323=CARTESIAN_POINT('Ctrl Pts',(2.49212731680301,-37.9742356128,-9.95194519152246));
#71324=CARTESIAN_POINT('Ctrl Pts',(2.4713374613571,-37.9742356128,-9.95617100136525));
#71325=CARTESIAN_POINT('Ctrl Pts',(2.45051702575423,-37.9742356128,-9.96034657813116));
#71326=CARTESIAN_POINT('Ctrl Pts',(2.42965942383348,-37.9742356128,-9.96447343814513));
#71327=CARTESIAN_POINT('Ctrl Pts',(2.39359814483382,-37.9742356128,-9.97160847940834));
#71328=CARTESIAN_POINT('Ctrl Pts',(2.35743385663318,-37.9742356128,-9.9785963109437));
#71329=CARTESIAN_POINT('Ctrl Pts',(2.32123184643125,-37.9742356128,-9.98542552600865));
#71330=CARTESIAN_POINT('Ctrl Pts',(2.29491518968168,-37.9742356128,-9.99038994946831));
#71331=CARTESIAN_POINT('Ctrl Pts',(2.26858128058276,-37.9742356128,-9.99527006010204));
#71332=CARTESIAN_POINT('Ctrl Pts',(2.24223429025926,-37.9742356128,-10.0000650689695));
#71333=CARTESIAN_POINT('Ctrl Pts',(2.21853740664891,-37.9742356128,-10.0043777728362));
#71334=CARTESIAN_POINT('Ctrl Pts',(2.1948308803507,-37.9742356128,-10.008621462852));
#71335=CARTESIAN_POINT('Ctrl Pts',(2.17107873562539,-37.9742356128,-10.0128024884733));
#71336=CARTESIAN_POINT('Ctrl Pts',(2.15245143750088,-37.9742356128,-10.0160814012458));
#71337=CARTESIAN_POINT('Ctrl Pts',(2.13379556879273,-37.9742356128,-10.0193218644102));
#71338=CARTESIAN_POINT('Ctrl Pts',(2.11506900102166,-37.9742356128,-10.0225313604444));
#71339=CARTESIAN_POINT('Ctrl Pts',(2.09995902895158,-37.9742356128,-10.025121017878));
#71340=CARTESIAN_POINT('Ctrl Pts',(2.08480873377376,-37.9742356128,-10.027689584587));
#71341=CARTESIAN_POINT('Ctrl Pts',(2.06954473665795,-37.9742356128,-10.0302496637803));
#71342=CARTESIAN_POINT('Ctrl Pts',(2.06589127481877,-37.9742356128,-10.0308624227822));
#71343=CARTESIAN_POINT('Ctrl Pts',(2.06223161231065,-37.9742356128,-10.031474641092));
#71344=CARTESIAN_POINT('Ctrl Pts',(2.05856513736635,-37.9742356128,-10.0320864240192));
#71345=CARTESIAN_POINT('Ctrl Pts',(2.0385286174435,-37.9742356128,-10.0354296899615));
#71346=CARTESIAN_POINT('Ctrl Pts',(2.01828403398492,-37.9742356128,-10.0387606184883));
#71347=CARTESIAN_POINT('Ctrl Pts',(1.99776023211584,-37.9742356128,-10.0420924842183));
#71348=CARTESIAN_POINT('Ctrl Pts',(1.9761101819271,-37.9742356128,-10.045607186842));
#71349=CARTESIAN_POINT('Ctrl Pts',(1.95414977844573,-37.9742356128,-10.0491228843939));
#71350=CARTESIAN_POINT('Ctrl Pts',(1.93185281336172,-37.9742356128,-10.0526469463018));
#71351=CARTESIAN_POINT('Ctrl Pts',(1.90630644189858,-37.9742356128,-10.0566845807608));
#71352=CARTESIAN_POINT('Ctrl Pts',(1.88031839144298,-37.9742356128,-10.0607331823361));
#71353=CARTESIAN_POINT('Ctrl Pts',(1.85392023551879,-37.9742356128,-10.0647936010473));
#71354=CARTESIAN_POINT('Ctrl Pts',(1.82217491673056,-37.9742356128,-10.069676490851));
#71355=CARTESIAN_POINT('Ctrl Pts',(1.78983837541185,-37.9742356128,-10.0745762225125));
#71356=CARTESIAN_POINT('Ctrl Pts',(1.757049426948,-37.9742356128,-10.0794819772469));
#71357=CARTESIAN_POINT('Ctrl Pts',(1.7270948216314,-37.9742356128,-10.0839636686013));
#71358=CARTESIAN_POINT('Ctrl Pts',(1.69676713389206,-37.9742356128,-10.0884497474174));
#71359=CARTESIAN_POINT('Ctrl Pts',(1.66618126682606,-37.9742356128,-10.0929303149498));
#71360=CARTESIAN_POINT('Ctrl Pts',(1.64013828901344,-37.9742356128,-10.0967453881202));
#71361=CARTESIAN_POINT('Ctrl Pts',(1.61390964456225,-37.9742356128,-10.1005562459663));
#71362=CARTESIAN_POINT('Ctrl Pts',(1.58753817424305,-37.9742356128,-10.1043605387549));
#71363=CARTESIAN_POINT('Ctrl Pts',(1.56338079239737,-37.9742356128,-10.1078454318016));
#71364=CARTESIAN_POINT('Ctrl Pts',(1.53910435580598,-37.9742356128,-10.1113247014488));
#71365=CARTESIAN_POINT('Ctrl Pts',(1.5147016560395,-37.9742356128,-10.1148020695187));
#71366=CARTESIAN_POINT('Ctrl Pts',(1.49244002770215,-37.9742356128,-10.1179743363705));
#71367=CARTESIAN_POINT('Ctrl Pts',(1.47007358539911,-37.9742356128,-10.121144981694));
#71368=CARTESIAN_POINT('Ctrl Pts',(1.44755531188353,-37.9742356128,-10.124322600884));
#71369=CARTESIAN_POINT('Ctrl Pts',(1.42751533029559,-37.9742356128,-10.1271505010788));
#71370=CARTESIAN_POINT('Ctrl Pts',(1.40735494258601,-37.9742356128,-10.1299839452806));
#71371=CARTESIAN_POINT('Ctrl Pts',(1.38700644577,-37.9742356128,-10.1328338118));
#71372=CARTESIAN_POINT('Ctrl Pts',(1.38699292008,-37.9742356128,-10.1328356959));
#71373=CARTESIAN_POINT('Ctrl Pts',(1.38699292008,-36.2942356128,-10.1328356959));
#71374=CARTESIAN_POINT('Ctrl Pts',(1.54048434157,-37.9742356128,-10.1113387667));
#71375=CARTESIAN_POINT('Ctrl Pts',(1.54048434157,-36.2942356128,-10.1113387667));
#71376=CARTESIAN_POINT('Ctrl Pts',(1.68405004863,-37.9742356128,-10.0907690318));
#71377=CARTESIAN_POINT('Ctrl Pts',(1.68405004863,-36.2942356128,-10.0907690318));
#71378=CARTESIAN_POINT('Ctrl Pts',(1.83768542134,-37.9742356128,-10.0680136806));
#71379=CARTESIAN_POINT('Ctrl Pts',(1.83768542134,-36.2942356128,-10.0680136806));
#71380=CARTESIAN_POINT('Ctrl Pts',(2.04726851031,-37.9742356128,-10.0350233698));
#71381=CARTESIAN_POINT('Ctrl Pts',(2.04726851031,-36.2942356128,-10.0350233698));
#71382=CARTESIAN_POINT('Ctrl Pts',(2.24744160945,-37.9742356128,-9.99950190736));
#71383=CARTESIAN_POINT('Ctrl Pts',(2.24744160945,-36.2942356128,-9.99950190736));
#71384=CARTESIAN_POINT('Ctrl Pts',(2.32512404468,-37.9742356128,-9.98507083709));
#71385=CARTESIAN_POINT('Ctrl Pts',(2.32512404468,-36.2942356128,-9.98507083709));
#71386=CARTESIAN_POINT('Ctrl Pts',(2.47861794588,-37.9742356128,-9.95531796777));
#71387=CARTESIAN_POINT('Ctrl Pts',(2.47861794588,-36.2942356128,-9.95531796777));
#71388=CARTESIAN_POINT('Ctrl Pts',(2.63158870596,-37.9742356128,-9.92313477939));
#71389=CARTESIAN_POINT('Ctrl Pts',(2.63158870596,-36.2942356128,-9.92313477939));
#71390=CARTESIAN_POINT('Ctrl Pts',(2.70802102447,-37.9742356128,-9.90641220657));
#71391=CARTESIAN_POINT('Ctrl Pts',(2.70802102447,-36.2942356128,-9.90641220657));
#71392=CARTESIAN_POINT('Ctrl Pts',(3.01253146546,-37.9742356128,-9.83720045464));
#71393=CARTESIAN_POINT('Ctrl Pts',(3.01253146546,-36.2942356128,-9.83720045464));
#71394=CARTESIAN_POINT('Ctrl Pts',(3.31446912359,-37.9742356128,-9.75814914821));
#71395=CARTESIAN_POINT('Ctrl Pts',(3.31446912359,-36.2942356128,-9.75814914821));
#71396=CARTESIAN_POINT('Ctrl Pts',(3.53901439179,-37.9742356128,-9.69332241165));
#71397=CARTESIAN_POINT('Ctrl Pts',(3.53901439179,-36.2942356128,-9.69332241165));
#71398=CARTESIAN_POINT('Ctrl Pts',(4.06616678437,-37.9742356128,-9.52655591089));
#71399=CARTESIAN_POINT('Ctrl Pts',(4.06616678437,-36.2942356128,-9.52655591089));
#71400=CARTESIAN_POINT('Ctrl Pts',(4.58136980215,-37.9742356128,-9.32859973652));
#71401=CARTESIAN_POINT('Ctrl Pts',(4.58136980215,-36.2942356128,-9.32859973652));
#71402=CARTESIAN_POINT('Ctrl Pts',(4.87486658279,-37.9742356128,-9.2037781865));
#71403=CARTESIAN_POINT('Ctrl Pts',(4.87486658279,-36.2942356128,-9.2037781865));
#71404=CARTESIAN_POINT('Ctrl Pts',(5.45178039508,-37.9742356128,-8.93423446359));
#71405=CARTESIAN_POINT('Ctrl Pts',(5.45178039508,-36.2942356128,-8.93423446359));
#71406=CARTESIAN_POINT('Ctrl Pts',(6.00853446953,-37.9742356128,-8.62630121911));
#71407=CARTESIAN_POINT('Ctrl Pts',(6.00853446953,-36.2942356128,-8.62630121911));
#71408=CARTESIAN_POINT('Ctrl Pts',(6.28153293634,-37.9742356128,-8.46325996647));
#71409=CARTESIAN_POINT('Ctrl Pts',(6.28153293634,-36.2942356128,-8.46325996647));
#71410=CARTESIAN_POINT('Ctrl Pts',(6.68293897532,-37.9742356128,-8.20578167079));
#71411=CARTESIAN_POINT('Ctrl Pts',(6.68293897532,-36.2942356128,-8.20578167079));
#71412=CARTESIAN_POINT('Ctrl Pts',(7.07391925378,-37.9742356128,-7.92965998368));
#71413=CARTESIAN_POINT('Ctrl Pts',(7.07391925378,-36.2942356128,-7.92965998368));
#71414=CARTESIAN_POINT('Ctrl Pts',(7.20312714754,-37.9742356128,-7.83561707229));
#71415=CARTESIAN_POINT('Ctrl Pts',(7.20312714754,-36.2942356128,-7.83561707229));
#71416=CARTESIAN_POINT('Ctrl Pts',(7.71835943349,-37.9742356128,-7.44951290201));
#71417=CARTESIAN_POINT('Ctrl Pts',(7.71835943349,-36.2942356128,-7.44951290201));
#71418=CARTESIAN_POINT('Ctrl Pts',(8.21985964708,-37.9742356128,-7.02884209136));
#71419=CARTESIAN_POINT('Ctrl Pts',(8.21985964708,-36.2942356128,-7.02884209136));
#71420=CARTESIAN_POINT('Ctrl Pts',(8.58741395086,-37.9742356128,-6.69445002697));
#71421=CARTESIAN_POINT('Ctrl Pts',(8.58741395086,-36.2942356128,-6.69445002697));
#71422=CARTESIAN_POINT('Ctrl Pts',(9.23922565917,-37.9742356128,-6.0447166144));
#71423=CARTESIAN_POINT('Ctrl Pts',(9.23922565917,-36.2942356128,-6.0447166144));
#71424=CARTESIAN_POINT('Ctrl Pts',(9.82149842762,-37.9742356128,-5.32595482066));
#71425=CARTESIAN_POINT('Ctrl Pts',(9.82149842762,-36.2942356128,-5.32595482066));
#71426=CARTESIAN_POINT('Ctrl Pts',(10.0721843915,-37.9742356128,-4.97806710985));
#71427=CARTESIAN_POINT('Ctrl Pts',(10.0721843915,-36.2942356128,-4.97806710985));
#71428=CARTESIAN_POINT('Ctrl Pts',(10.6524574839,-37.9742356128,-4.03375119457));
#71429=CARTESIAN_POINT('Ctrl Pts',(10.6524574839,-36.2942356128,-4.03375119457));
#71430=CARTESIAN_POINT('Ctrl Pts',(11.0291793988,-37.9742356128,-2.98459593105));
#71431=CARTESIAN_POINT('Ctrl Pts',(11.0291793988,-36.2942356128,-2.98459593105));
#71432=CARTESIAN_POINT('Ctrl Pts',(11.1622899815,-37.9742356128,-2.31636115629));
#71433=CARTESIAN_POINT('Ctrl Pts',(11.1622899815,-36.2942356128,-2.31636115629));
#71434=CARTESIAN_POINT('Ctrl Pts',(11.2336540706,-37.9742356128,-1.36618233638));
#71435=CARTESIAN_POINT('Ctrl Pts',(11.2336540706,-36.2942356128,-1.36618233638));
#71436=CARTESIAN_POINT('Ctrl Pts',(11.1889875368,-37.9742356128,-0.434883867498));
#71437=CARTESIAN_POINT('Ctrl Pts',(11.1889875368,-36.2942356128,-0.434883867498));
#71438=CARTESIAN_POINT('Ctrl Pts',(11.1677658434,-37.9742356128,-0.163547364245));
#71439=CARTESIAN_POINT('Ctrl Pts',(11.1677658434,-36.2942356128,-0.163547364245));
#71440=CARTESIAN_POINT('Ctrl Pts',(11.1309935407,-37.9742356128,0.191196052993));
#71441=CARTESIAN_POINT('Ctrl Pts',(11.1309935407,-36.2942356128,0.191196052993));
#71442=CARTESIAN_POINT('Ctrl Pts',(11.0837537732,-37.9742356128,0.541839826087));
#71443=CARTESIAN_POINT('Ctrl Pts',(11.0837537732,-36.2942356128,0.541839826087));
#71444=CARTESIAN_POINT('Ctrl Pts',(11.0714556362,-37.9742356128,0.628315856355));
#71445=CARTESIAN_POINT('Ctrl Pts',(11.0714556362,-36.2942356128,0.628315856355));
#71446=CARTESIAN_POINT('Ctrl Pts',(11.0585597994,-37.9742356128,0.714566551433));
#71447=CARTESIAN_POINT('Ctrl Pts',(11.0585597994,-36.2942356128,0.714566551433));
#71448=CARTESIAN_POINT('Ctrl Pts',(11.0450673741,-37.9742356128,0.800650704934));
#71449=CARTESIAN_POINT('Ctrl Pts',(11.0450673741,-36.2942356128,0.800650704934));
#71450=CARTESIAN_POINT('',(11.0450673741,-37.2742356128,0.800650704934));
#71451=CARTESIAN_POINT('Ctrl Pts',(10.3257952821,-36.5742356128,3.01322822759));
#71452=CARTESIAN_POINT('Ctrl Pts',(10.3257952821,-36.4799878332,3.01322822759));
#71453=CARTESIAN_POINT('Ctrl Pts',(10.2942035846,-36.3857400536,2.99394663035));
#71454=CARTESIAN_POINT('Ctrl Pts',(10.2306178216,-36.3112466293,2.95513785557));
#71455=CARTESIAN_POINT('Ctrl Pts',(10.1501702245,-36.2742356128,2.90603767139));
#71456=CARTESIAN_POINT('Ctrl Pts',(10.0697226274,-36.2742356128,2.85693748721));
#71457=CARTESIAN_POINT('Ctrl Pts',(10.3937468068,-36.5742356128,2.90189388187));
#71458=CARTESIAN_POINT('Ctrl Pts',(10.3937468068,-36.4799878332,2.90189388187));
#71459=CARTESIAN_POINT('Ctrl Pts',(10.361743269,-36.3857400536,2.88328705955));
#71460=CARTESIAN_POINT('Ctrl Pts',(10.2973285787,-36.3112466293,2.84583643038));
#71461=CARTESIAN_POINT('Ctrl Pts',(10.2158322378,-36.2742356128,2.79845454767));
#71462=CARTESIAN_POINT('Ctrl Pts',(10.1343358969,-36.2742356128,2.75107266497));
#71463=CARTESIAN_POINT('Ctrl Pts',(10.4620487356,-36.5742356128,2.78329337524));
#71464=CARTESIAN_POINT('Ctrl Pts',(10.4620487075,-36.4799878222,2.78329342192));
#71465=CARTESIAN_POINT('Ctrl Pts',(10.4295091719,-36.3857400315,2.76560455904));
#71466=CARTESIAN_POINT('Ctrl Pts',(10.3640156965,-36.3112466033,2.7300014792));
#71467=CARTESIAN_POINT('Ctrl Pts',(10.2811545152,-36.2742355955,2.68495705923));
#71468=CARTESIAN_POINT('Ctrl Pts',(10.1982933508,-36.2742356128,2.63991262435));
#71469=CARTESIAN_POINT('Ctrl Pts',(10.5258464853,-36.5742356128,2.66146373578));
#71470=CARTESIAN_POINT('Ctrl Pts',(10.5258464925,-36.4799878342,2.66146372337));
#71471=CARTESIAN_POINT('Ctrl Pts',(10.49275753,-36.3857400555,2.64481822146));
#71472=CARTESIAN_POINT('Ctrl Pts',(10.4261581581,-36.3112466315,2.61131522692));
#71473=CARTESIAN_POINT('Ctrl Pts',(10.3418977911,-36.2742356143,2.5689278305));
#71474=CARTESIAN_POINT('Ctrl Pts',(10.257637421,-36.2742356128,2.52654043836));
#71475=CARTESIAN_POINT('Ctrl Pts',(10.6432548222,-36.5742356128,2.41313758791));
#71476=CARTESIAN_POINT('Ctrl Pts',(10.643254815,-36.4799878323,2.41313760034));
#71477=CARTESIAN_POINT('Ctrl Pts',(10.6091443507,-36.3857400518,2.39865283441));
#71478=CARTESIAN_POINT('Ctrl Pts',(10.5404889831,-36.3112466272,2.36949880159));
#71479=CARTESIAN_POINT('Ctrl Pts',(10.4536274153,-36.2742356114,2.33261362134));
#71480=CARTESIAN_POINT('Ctrl Pts',(10.3667658506,-36.2742356128,2.29572843681));
#71481=CARTESIAN_POINT('Ctrl Pts',(10.7398872019,-36.5742356128,2.15784469508));
#71482=CARTESIAN_POINT('Ctrl Pts',(10.7398872091,-36.4799878342,2.15784468263));
#71483=CARTESIAN_POINT('Ctrl Pts',(10.7049465072,-36.3857400555,2.1455561634));
#71484=CARTESIAN_POINT('Ctrl Pts',(10.6346200712,-36.3112466315,2.12082262831));
#71485=CARTESIAN_POINT('Ctrl Pts',(10.5456442881,-36.2742356143,2.08953019835));
#71486=CARTESIAN_POINT('Ctrl Pts',(10.4566685018,-36.2742356128,2.05823777268));
#71487=CARTESIAN_POINT('Ctrl Pts',(10.7831182422,-36.5742356128,2.02819080292));
#71488=CARTESIAN_POINT('Ctrl Pts',(10.7831182402,-36.479987836,2.02819080957));
#71489=CARTESIAN_POINT('Ctrl Pts',(10.7478302137,-36.3857400592,2.0169555735));
#71490=CARTESIAN_POINT('Ctrl Pts',(10.6768047166,-36.311246636,1.9943419946));
#71491=CARTESIAN_POINT('Ctrl Pts',(10.5869444982,-36.2742356173,1.96573168544));
#71492=CARTESIAN_POINT('Ctrl Pts',(10.4970842789,-36.2742356128,1.93712137311));
#71493=CARTESIAN_POINT('Ctrl Pts',(10.8542127323,-36.5742356128,1.78659505536));
#71494=CARTESIAN_POINT('Ctrl Pts',(10.8542127341,-36.4799878308,1.78659504957));
#71495=CARTESIAN_POINT('Ctrl Pts',(10.818391418,-36.3857400487,1.77719284878));
#71496=CARTESIAN_POINT('Ctrl Pts',(10.746292545,-36.3112466236,1.75826870283));
#71497=CARTESIAN_POINT('Ctrl Pts',(10.6550743098,-36.274235609,1.73432620773));
#71498=CARTESIAN_POINT('Ctrl Pts',(10.5638560753,-36.2742356128,1.71038371539));
#71499=CARTESIAN_POINT('Ctrl Pts',(10.9096968315,-36.5742356128,1.5493422145));
#71500=CARTESIAN_POINT('Ctrl Pts',(10.9096968299,-36.4799878354,1.54934221954));
#71501=CARTESIAN_POINT('Ctrl Pts',(10.8735444913,-36.3857400579,1.54137680968));
#71502=CARTESIAN_POINT('Ctrl Pts',(10.8007793611,-36.3112466344,1.52534453328));
#71503=CARTESIAN_POINT('Ctrl Pts',(10.7087181892,-36.2742356162,1.50506077338));
#71504=CARTESIAN_POINT('Ctrl Pts',(10.6166570167,-36.2742356128,1.48477701108));
#71505=CARTESIAN_POINT('Ctrl Pts',(10.9325897702,-36.5742356128,1.44085989855));
#71506=CARTESIAN_POINT('Ctrl Pts',(10.9325897728,-36.4799878363,1.44085988415));
#71507=CARTESIAN_POINT('Ctrl Pts',(10.8963180592,-36.3857400597,1.43348398822));
#71508=CARTESIAN_POINT('Ctrl Pts',(10.8233126521,-36.3112466366,1.41863827973));
#71509=CARTESIAN_POINT('Ctrl Pts',(10.7309474837,-36.2742356176,1.3998557533));
#71510=CARTESIAN_POINT('Ctrl Pts',(10.6385823125,-36.2742356128,1.38107323223));
#71511=CARTESIAN_POINT('Ctrl Pts',(10.9702924284,-36.5742356128,1.24661939192));
#71512=CARTESIAN_POINT('Ctrl Pts',(10.9702924263,-36.4799878308,1.24661940331));
#71513=CARTESIAN_POINT('Ctrl Pts',(10.9338862965,-36.3857400488,1.23993800485));
#71514=CARTESIAN_POINT('Ctrl Pts',(10.8606103532,-36.3112466236,1.22649008978));
#71515=CARTESIAN_POINT('Ctrl Pts',(10.7679029112,-36.274235609,1.20947601848));
#71516=CARTESIAN_POINT('Ctrl Pts',(10.6751954713,-36.2742356128,1.19246194295));
#71517=CARTESIAN_POINT('Ctrl Pts',(11.0025979433,-36.5742356128,1.06106603291));
#71518=CARTESIAN_POINT('Ctrl Pts',(11.0025979449,-36.4799878351,1.0610660239));
#71519=CARTESIAN_POINT('Ctrl Pts',(10.9661101376,-36.3857400575,1.05486169103));
#71520=CARTESIAN_POINT('Ctrl Pts',(10.8926697928,-36.3112466339,1.04237401943));
#71521=CARTESIAN_POINT('Ctrl Pts',(10.7997543496,-36.2742356158,1.02657483871));
#71522=CARTESIAN_POINT('Ctrl Pts',(10.7068389045,-36.2742356128,1.01077566133));
#71523=CARTESIAN_POINT('Ctrl Pts',(11.0186198552,-36.5742356128,0.965719195611));
#71524=CARTESIAN_POINT('Ctrl Pts',(11.0186198914,-36.4799878336,0.965718974446));
#71525=CARTESIAN_POINT('Ctrl Pts',(10.9821161692,-36.3857400544,0.959609890492));
#71526=CARTESIAN_POINT('Ctrl Pts',(10.9086437537,-36.3112466303,0.947314164305));
#71527=CARTESIAN_POINT('Ctrl Pts',(10.8156877131,-36.2742356135,0.931757969109));
#71528=CARTESIAN_POINT('Ctrl Pts',(10.722731658,-36.2742356128,0.916201860672));
#71529=CARTESIAN_POINT('Ctrl Pts',(11.0320114918,-36.5742356128,0.883950471231));
#71530=CARTESIAN_POINT('Ctrl Pts',(11.0320115123,-36.4799878331,0.883950339438));
#71531=CARTESIAN_POINT('Ctrl Pts',(10.9954782575,-36.3857400535,0.878019250857));
#71532=CARTESIAN_POINT('Ctrl Pts',(10.9219464145,-36.3112466291,0.866081706745));
#71533=CARTESIAN_POINT('Ctrl Pts',(10.828915199,-36.2742356127,0.85097860876));
#71534=CARTESIAN_POINT('Ctrl Pts',(10.7358839755,-36.2742356128,0.835875562575));
#71535=CARTESIAN_POINT('Ctrl Pts',(11.0450658874,-36.5742356128,0.800660309528));
#71536=CARTESIAN_POINT('Ctrl Pts',(11.0450658931,-36.4799878332,0.800660273261));
#71537=CARTESIAN_POINT('Ctrl Pts',(11.0085012867,-36.3857400536,0.794929224556));
#71538=CARTESIAN_POINT('Ctrl Pts',(10.9349063615,-36.3112466293,0.783394177901));
#71539=CARTESIAN_POINT('Ctrl Pts',(10.8417953438,-36.2742356128,0.768800260322));
#71540=CARTESIAN_POINT('Ctrl Pts',(10.7486843238,-36.2742356128,0.754206356986));
#71541=CARTESIAN_POINT('Ctrl Pts',(10.3257952821,-36.5742356128,3.01322822759));
#71542=CARTESIAN_POINT('Ctrl Pts',(10.3992001828,-36.5742356128,2.89295886461));
#71543=CARTESIAN_POINT('Ctrl Pts',(10.4735263391,-36.5742356128,2.76337956773));
#71544=CARTESIAN_POINT('Ctrl Pts',(10.5420136,-36.5742356128,2.63031881231));
#71545=CARTESIAN_POINT('Ctrl Pts',(10.6667840474,-36.5742356128,2.3591848401));
#71546=CARTESIAN_POINT('Ctrl Pts',(10.7670166783,-36.5742356128,2.08017125701));
#71547=CARTESIAN_POINT('Ctrl Pts',(10.8111933802,-36.5742356128,1.9383801789));
#71548=CARTESIAN_POINT('Ctrl Pts',(10.8740649015,-36.5742356128,1.70707199422));
#71549=CARTESIAN_POINT('Ctrl Pts',(10.9239906907,-36.5742356128,1.48074082922));
#71550=CARTESIAN_POINT('Ctrl Pts',(10.9420747597,-36.5742356128,1.39194060496));
#71551=CARTESIAN_POINT('Ctrl Pts',(10.9747007143,-36.5742356128,1.22147170256));
#71552=CARTESIAN_POINT('Ctrl Pts',(11.0034487643,-36.5742356128,1.05599081154));
#71553=CARTESIAN_POINT('Ctrl Pts',(11.0192230845,-36.5742356128,0.962056436866));
#71554=CARTESIAN_POINT('Ctrl Pts',(11.0322998284,-36.5742356128,0.882109993579));
#71555=CARTESIAN_POINT('Ctrl Pts',(11.0450673741,-36.5742356128,0.800650704934));
#71556=CARTESIAN_POINT('Ctrl Pts',(10.7486858853,-38.2742356128,0.75419629452));
#71557=CARTESIAN_POINT('Ctrl Pts',(10.8417968709,-38.2742356128,0.768790414629));
#71558=CARTESIAN_POINT('Ctrl Pts',(10.9349078565,-38.2372245963,0.783384534738));
#71559=CARTESIAN_POINT('Ctrl Pts',(11.0085027591,-38.1627311721,0.794919724064));
#71560=CARTESIAN_POINT('Ctrl Pts',(11.0450673576,-38.0684833924,0.800650821629));
#71561=CARTESIAN_POINT('Ctrl Pts',(11.0450673576,-37.9742356128,0.800650821629));
#71562=CARTESIAN_POINT('Ctrl Pts',(10.7357744891,-38.2742356128,0.836572947324));
#71563=CARTESIAN_POINT('Ctrl Pts',(10.8288041791,-38.2742356128,0.851685759842));
#71564=CARTESIAN_POINT('Ctrl Pts',(10.9218338691,-38.2372245963,0.86679857236));
#71565=CARTESIAN_POINT('Ctrl Pts',(10.9953645154,-38.1627311721,0.878743737491));
#71566=CARTESIAN_POINT('Ctrl Pts',(11.0318971895,-38.0684833924,0.884678523649));
#71567=CARTESIAN_POINT('Ctrl Pts',(11.0318971895,-37.9742356128,0.884678523649));
#71568=CARTESIAN_POINT('Ctrl Pts',(10.722464663,-38.2742356128,0.917844462815));
#71569=CARTESIAN_POINT('Ctrl Pts',(10.8154219344,-38.2742356128,0.933393309198));
#71570=CARTESIAN_POINT('Ctrl Pts',(10.9083792058,-38.2372245963,0.948942155581));
#71571=CARTESIAN_POINT('Ctrl Pts',(10.9818526127,-38.1627311721,0.961231959982));
#71572=CARTESIAN_POINT('Ctrl Pts',(11.0183568478,-38.0684833924,0.96733797804));
#71573=CARTESIAN_POINT('Ctrl Pts',(11.0183568478,-37.9742356128,0.96733797804));
#71574=CARTESIAN_POINT('Ctrl Pts',(10.7064160578,-38.2742356128,1.01327576595));
#71575=CARTESIAN_POINT('Ctrl Pts',(10.7993296705,-38.2742356128,1.02908657461));
#71576=CARTESIAN_POINT('Ctrl Pts',(10.8922432832,-38.2372245963,1.04489738327));
#71577=CARTESIAN_POINT('Ctrl Pts',(10.9656821815,-38.1627311721,1.05739424674));
#71578=CARTESIAN_POINT('Ctrl Pts',(11.0021692726,-38.0684833924,1.06360313301));
#71579=CARTESIAN_POINT('Ctrl Pts',(11.0021692726,-37.9742356128,1.06360313301));
#71580=CARTESIAN_POINT('Ctrl Pts',(10.6699861172,-38.2742356128,1.22225589069));
#71581=CARTESIAN_POINT('Ctrl Pts',(10.7626589385,-38.2742356128,1.23947073278));
#71582=CARTESIAN_POINT('Ctrl Pts',(10.8553317597,-38.2372245963,1.25668557487));
#71583=CARTESIAN_POINT('Ctrl Pts',(10.9285803371,-38.1627311721,1.27029218249));
#71584=CARTESIAN_POINT('Ctrl Pts',(10.964972869,-38.0684833924,1.27705243495));
#71585=CARTESIAN_POINT('Ctrl Pts',(10.964972869,-37.9742356128,1.27705243495));
#71586=CARTESIAN_POINT('Ctrl Pts',(10.6268374654,-38.2742356128,1.44080864883));
#71587=CARTESIAN_POINT('Ctrl Pts',(10.7190870973,-38.2742356128,1.46018401586));
#71588=CARTESIAN_POINT('Ctrl Pts',(10.8113367292,-38.2372245963,1.4795593829));
#71589=CARTESIAN_POINT('Ctrl Pts',(10.8842508199,-38.1627311721,1.49487365862));
#71590=CARTESIAN_POINT('Ctrl Pts',(10.9204771637,-38.0684833924,1.50248235758));
#71591=CARTESIAN_POINT('Ctrl Pts',(10.9204771637,-37.9742356128,1.50248235758));
#71592=CARTESIAN_POINT('Ctrl Pts',(10.5978372142,-38.2742356128,1.57143060617));
#71593=CARTESIAN_POINT('Ctrl Pts',(10.689631737,-38.2742356128,1.59298148681));
#71594=CARTESIAN_POINT('Ctrl Pts',(10.7814262599,-38.2372245963,1.61453236745));
#71595=CARTESIAN_POINT('Ctrl Pts',(10.8539806029,-38.1627311721,1.63156622296));
#71596=CARTESIAN_POINT('Ctrl Pts',(10.8900282554,-38.0684833924,1.64002918981));
#71597=CARTESIAN_POINT('Ctrl Pts',(10.8900282554,-37.9742356128,1.64002918981));
#71598=CARTESIAN_POINT('Ctrl Pts',(10.5099314906,-38.2742356128,1.91769651998));
#71599=CARTESIAN_POINT('Ctrl Pts',(10.6001579466,-38.2742356128,1.94553878808));
#71600=CARTESIAN_POINT('Ctrl Pts',(10.6903844027,-38.2372245963,1.97338105617));
#71601=CARTESIAN_POINT('Ctrl Pts',(10.761699418,-38.1627311721,1.9953875076));
#71602=CARTESIAN_POINT('Ctrl Pts',(10.7971312201,-38.0684833924,2.00632121187));
#71603=CARTESIAN_POINT('Ctrl Pts',(10.7971312201,-37.9742356128,2.00632121187));
#71604=CARTESIAN_POINT('Ctrl Pts',(10.3851598454,-38.2742356128,2.26389944964));
#71605=CARTESIAN_POINT('Ctrl Pts',(10.4725421188,-38.2742356128,2.29983157374));
#71606=CARTESIAN_POINT('Ctrl Pts',(10.5599243922,-38.2372245963,2.33576369785));
#71607=CARTESIAN_POINT('Ctrl Pts',(10.628991251,-38.1627311721,2.36416455541));
#71608=CARTESIAN_POINT('Ctrl Pts',(10.6633062605,-38.0684833924,2.37827495298));
#71609=CARTESIAN_POINT('Ctrl Pts',(10.6633062605,-37.9742356128,2.37827495298));
#71610=CARTESIAN_POINT('Ctrl Pts',(10.2956098407,-38.2742356128,2.46622288607));
#71611=CARTESIAN_POINT('Ctrl Pts',(10.3807463521,-38.2742356128,2.50731926973));
#71612=CARTESIAN_POINT('Ctrl Pts',(10.4658828634,-38.2372245963,2.54841565339));
#71613=CARTESIAN_POINT('Ctrl Pts',(10.5331750304,-38.1627311721,2.58089775529));
#71614=CARTESIAN_POINT('Ctrl Pts',(10.5666077732,-38.0684833924,2.59703673813));
#71615=CARTESIAN_POINT('Ctrl Pts',(10.5666077732,-37.9742356128,2.59703673813));
#71616=CARTESIAN_POINT('Ctrl Pts',(10.1838372262,-38.2742356128,2.66996781664));
#71617=CARTESIAN_POINT('Ctrl Pts',(10.2661370276,-38.2742356128,2.71603327924));
#71618=CARTESIAN_POINT('Ctrl Pts',(10.348436829,-38.2372245963,2.76209874184));
#71619=CARTESIAN_POINT('Ctrl Pts',(10.4134863826,-38.1627311721,2.79850918724));
#71620=CARTESIAN_POINT('Ctrl Pts',(10.4458056304,-38.0684833924,2.8165987382));
#71621=CARTESIAN_POINT('Ctrl Pts',(10.4458056304,-37.9742356128,2.8165987382));
#71622=CARTESIAN_POINT('Ctrl Pts',(10.0697226274,-38.2742356128,2.85693748721));
#71623=CARTESIAN_POINT('Ctrl Pts',(10.1501702245,-38.2742356128,2.90603767139));
#71624=CARTESIAN_POINT('Ctrl Pts',(10.2306178216,-38.2372245963,2.95513785557));
#71625=CARTESIAN_POINT('Ctrl Pts',(10.2942035846,-38.1627311721,2.99394663035));
#71626=CARTESIAN_POINT('Ctrl Pts',(10.3257952821,-38.0684833924,3.01322822759));
#71627=CARTESIAN_POINT('Ctrl Pts',(10.3257952821,-37.9742356128,3.01322822759));
#71628=CARTESIAN_POINT('Ctrl Pts',(10.3257952821,-37.9742356128,3.01322822759));
#71629=CARTESIAN_POINT('Ctrl Pts',(10.3435108770889,-37.9742356128,2.98420232735513));
#71630=CARTESIAN_POINT('Ctrl Pts',(10.3612660726275,-37.9742356128,2.95454361401332));
#71631=CARTESIAN_POINT('Ctrl Pts',(10.3789029130837,-37.9742356128,2.92440130957732));
#71632=CARTESIAN_POINT('Ctrl Pts',(10.3970692021044,-37.9742356128,2.89335414920351));
#71633=CARTESIAN_POINT('Ctrl Pts',(10.4151099921331,-37.9742356128,2.86179373744858));
#71634=CARTESIAN_POINT('Ctrl Pts',(10.4328934056652,-37.9742356128,2.82984504858017));
#71635=CARTESIAN_POINT('Ctrl Pts',(10.4513725247225,-37.9742356128,2.7966464939688));
#71636=CARTESIAN_POINT('Ctrl Pts',(10.4695738352306,-37.9742356128,2.76302842606344));
#71637=CARTESIAN_POINT('Ctrl Pts',(10.4873915130274,-37.9742356128,2.72909395600771));
#71638=CARTESIAN_POINT('Ctrl Pts',(10.506746145179,-37.9742356128,2.69223229576914));
#71639=CARTESIAN_POINT('Ctrl Pts',(10.5256480261522,-37.9742356128,2.65499706078238));
#71640=CARTESIAN_POINT('Ctrl Pts',(10.5440106698345,-37.9742356128,2.61748093307006));
#71641=CARTESIAN_POINT('Ctrl Pts',(10.5638797850415,-37.9742356128,2.57688698175579));
#71642=CARTESIAN_POINT('Ctrl Pts',(10.5831177873975,-37.9742356128,2.53596344249259));
#71643=CARTESIAN_POINT('Ctrl Pts',(10.6016693303391,-37.9742356128,2.49479084421754));
#71644=CARTESIAN_POINT('Ctrl Pts',(10.6162942510062,-37.9742356128,2.46233284407569));
#71645=CARTESIAN_POINT('Ctrl Pts',(10.6304938506889,-37.9742356128,2.42971906581169));
#71646=CARTESIAN_POINT('Ctrl Pts',(10.6442593718278,-37.9742356128,2.39698023320332));
#71647=CARTESIAN_POINT('Ctrl Pts',(10.6569750338918,-37.9742356128,2.36673830283123));
#71648=CARTESIAN_POINT('Ctrl Pts',(10.6693194231973,-37.9742356128,2.33639290955639));
#71649=CARTESIAN_POINT('Ctrl Pts',(10.6813046418276,-37.9742356128,2.30593898856114));
#71650=CARTESIAN_POINT('Ctrl Pts',(10.7005865729481,-37.9742356128,2.25694443743201));
#71651=CARTESIAN_POINT('Ctrl Pts',(10.718933686294,-37.9742356128,2.2076779701046));
#71652=CARTESIAN_POINT('Ctrl Pts',(10.7363740820652,-37.9742356128,2.15823655988335));
#71653=CARTESIAN_POINT('Ctrl Pts',(10.7508645620954,-37.9742356128,2.11715780359402));
#71654=CARTESIAN_POINT('Ctrl Pts',(10.7647302536249,-37.9742356128,2.07595786403464));
#71655=CARTESIAN_POINT('Ctrl Pts',(10.7779838592388,-37.9742356128,2.03472677202854));
#71656=CARTESIAN_POINT('Ctrl Pts',(10.7900447242869,-37.9742356128,1.99720621717286));
#71657=CARTESIAN_POINT('Ctrl Pts',(10.8015991768384,-37.9742356128,1.95965960974327));
#71658=CARTESIAN_POINT('Ctrl Pts',(10.8126441119714,-37.9742356128,1.92219040368875));
#71659=CARTESIAN_POINT('Ctrl Pts',(10.8236166119916,-37.9742356128,1.88496692892495));
#71660=CARTESIAN_POINT('Ctrl Pts',(10.8340837193902,-37.9742356128,1.84782839628653));
#71661=CARTESIAN_POINT('Ctrl Pts',(10.8440841088843,-37.9742356128,1.81083470663686));
#71662=CARTESIAN_POINT('Ctrl Pts',(10.8559248749312,-37.9742356128,1.76703305025062));
#71663=CARTESIAN_POINT('Ctrl Pts',(10.8671115731973,-37.9742356128,1.72343299507352));
#71664=CARTESIAN_POINT('Ctrl Pts',(10.8777255157072,-37.9742356128,1.68005510341546));
#71665=CARTESIAN_POINT('Ctrl Pts',(10.8816732452895,-37.9742356128,1.66392121292609));
#71666=CARTESIAN_POINT('Ctrl Pts',(10.8855420335377,-37.9742356128,1.64781665780391));
#71667=CARTESIAN_POINT('Ctrl Pts',(10.88933297735,-37.9742356128,1.63175608320554));
#71668=CARTESIAN_POINT('Ctrl Pts',(10.8993385050894,-37.9742356128,1.58936702849724));
#71669=CARTESIAN_POINT('Ctrl Pts',(10.9088091071911,-37.9742356128,1.54725502348625));
#71670=CARTESIAN_POINT('Ctrl Pts',(10.9178378693608,-37.9742356128,1.50538883341575));
#71671=CARTESIAN_POINT('Ctrl Pts',(10.9255930579366,-37.9742356128,1.46942817869433));
#71672=CARTESIAN_POINT('Ctrl Pts',(10.9330224352445,-37.9742356128,1.43364757364882));
#71673=CARTESIAN_POINT('Ctrl Pts',(10.9401770982342,-37.9742356128,1.39806231067591));
#71674=CARTESIAN_POINT('Ctrl Pts',(10.9465294246673,-37.9742356128,1.36646764200538));
#71675=CARTESIAN_POINT('Ctrl Pts',(10.9526652330497,-37.9742356128,1.33502659574014));
#71676=CARTESIAN_POINT('Ctrl Pts',(10.9586123994879,-37.9742356128,1.30378932417771));
#71677=CARTESIAN_POINT('Ctrl Pts',(10.9632698278339,-37.9742356128,1.2793263542004));
#71678=CARTESIAN_POINT('Ctrl Pts',(10.9678114424312,-37.9742356128,1.25498893556002));
#71679=CARTESIAN_POINT('Ctrl Pts',(10.9722463818661,-37.9742356128,1.23082335732336));
#71680=CARTESIAN_POINT('Ctrl Pts',(10.9744000643225,-37.9742356128,1.2190881391401));
#71681=CARTESIAN_POINT('Ctrl Pts',(10.9765290742772,-37.9742356128,1.20739061189226));
#71682=CARTESIAN_POINT('Ctrl Pts',(10.9786472561583,-37.9742356128,1.19565808724385));
#71683=CARTESIAN_POINT('Ctrl Pts',(10.981079762963,-37.9742356128,1.1821845294256));
#71684=CARTESIAN_POINT('Ctrl Pts',(10.9834978391073,-37.9742356128,1.16866563142089));
#71685=CARTESIAN_POINT('Ctrl Pts',(10.98591187279,-37.9742356128,1.15505222871516));
#71686=CARTESIAN_POINT('Ctrl Pts',(10.9886383738725,-37.9742356128,1.13967673603612));
#71687=CARTESIAN_POINT('Ctrl Pts',(10.9913597243006,-37.9742356128,1.12418073304783));
#71688=CARTESIAN_POINT('Ctrl Pts',(10.9940787041515,-37.9742356128,1.10856313499871));
#71689=CARTESIAN_POINT('Ctrl Pts',(10.9972032177,-37.9742356128,1.09061618453343));
#71690=CARTESIAN_POINT('Ctrl Pts',(11.0003244602367,-37.9742356128,1.07250966807065));
#71691=CARTESIAN_POINT('Ctrl Pts',(11.0034323169338,-37.9742356128,1.05432169160246));
#71692=CARTESIAN_POINT('Ctrl Pts',(11.0072388611408,-37.9742356128,1.03204481618283));
#71693=CARTESIAN_POINT('Ctrl Pts',(11.0110245978049,-37.9742356128,1.00965060914404));
#71694=CARTESIAN_POINT('Ctrl Pts',(11.0147570943917,-37.9742356128,0.987350997854593));
#71695=CARTESIAN_POINT('Ctrl Pts',(11.017586140657,-37.9742356128,0.97044900462676));
#71696=CARTESIAN_POINT('Ctrl Pts',(11.0203841001757,-37.9742356128,0.953604041000246));
#71697=CARTESIAN_POINT('Ctrl Pts',(11.0231387163433,-37.9742356128,0.936890599639805));
#71698=CARTESIAN_POINT('Ctrl Pts',(11.0256260652016,-37.9742356128,0.921798784026464));
#71699=CARTESIAN_POINT('Ctrl Pts',(11.0280779020287,-37.9742356128,0.906815173063734));
#71700=CARTESIAN_POINT('Ctrl Pts',(11.0304906336531,-37.9742356128,0.891957832231274));
#71701=CARTESIAN_POINT('Ctrl Pts',(11.0327503987612,-37.9742356128,0.878042442690342));
#71702=CARTESIAN_POINT('Ctrl Pts',(11.0349757566118,-37.9742356128,0.864238410878224));
#71703=CARTESIAN_POINT('Ctrl Pts',(11.0371706175412,-37.9742356128,0.850516112005006));
#71704=CARTESIAN_POINT('Ctrl Pts',(11.039226797446,-37.9742356128,0.837660848688127));
#71705=CARTESIAN_POINT('Ctrl Pts',(11.0412561654325,-37.9742356128,0.824877574458748));
#71706=CARTESIAN_POINT('Ctrl Pts',(11.0432691636105,-37.9742356128,0.812095953182369));
#71707=CARTESIAN_POINT('Ctrl Pts',(11.0438698244563,-37.9742356128,0.80828203048223));
#71708=CARTESIAN_POINT('Ctrl Pts',(11.0444690817224,-37.9742356128,0.804467913923509));
#71709=CARTESIAN_POINT('Ctrl Pts',(11.0450673576,-37.9742356128,0.800650821629));
#71710=CARTESIAN_POINT('Ctrl Pts',(11.0450673741,-37.9742356128,0.800650704934));
#71711=CARTESIAN_POINT('Ctrl Pts',(11.0450673741,-36.2942356128,0.800650704934));
#71712=CARTESIAN_POINT('Ctrl Pts',(11.0322998284,-37.9742356128,0.882109993579));
#71713=CARTESIAN_POINT('Ctrl Pts',(11.0322998284,-36.2942356128,0.882109993579));
#71714=CARTESIAN_POINT('Ctrl Pts',(11.0192230845,-37.9742356128,0.962056436866));
#71715=CARTESIAN_POINT('Ctrl Pts',(11.0192230845,-36.2942356128,0.962056436866));
#71716=CARTESIAN_POINT('Ctrl Pts',(11.0034487643,-37.9742356128,1.05599081154));
#71717=CARTESIAN_POINT('Ctrl Pts',(11.0034487643,-36.2942356128,1.05599081154));
#71718=CARTESIAN_POINT('Ctrl Pts',(10.9747007143,-37.9742356128,1.22147170256));
#71719=CARTESIAN_POINT('Ctrl Pts',(10.9747007143,-36.2942356128,1.22147170256));
#71720=CARTESIAN_POINT('Ctrl Pts',(10.9420747597,-37.9742356128,1.39194060496));
#71721=CARTESIAN_POINT('Ctrl Pts',(10.9420747597,-36.2942356128,1.39194060496));
#71722=CARTESIAN_POINT('Ctrl Pts',(10.9239906907,-37.9742356128,1.48074082922));
#71723=CARTESIAN_POINT('Ctrl Pts',(10.9239906907,-36.2942356128,1.48074082922));
#71724=CARTESIAN_POINT('Ctrl Pts',(10.8740649015,-37.9742356128,1.70707199422));
#71725=CARTESIAN_POINT('Ctrl Pts',(10.8740649015,-36.2942356128,1.70707199422));
#71726=CARTESIAN_POINT('Ctrl Pts',(10.8111933802,-37.9742356128,1.9383801789));
#71727=CARTESIAN_POINT('Ctrl Pts',(10.8111933802,-36.2942356128,1.9383801789));
#71728=CARTESIAN_POINT('Ctrl Pts',(10.7670166783,-37.9742356128,2.08017125701));
#71729=CARTESIAN_POINT('Ctrl Pts',(10.7670166783,-36.2942356128,2.08017125701));
#71730=CARTESIAN_POINT('Ctrl Pts',(10.6667840474,-37.9742356128,2.3591848401));
#71731=CARTESIAN_POINT('Ctrl Pts',(10.6667840474,-36.2942356128,2.3591848401));
#71732=CARTESIAN_POINT('Ctrl Pts',(10.5420136,-37.9742356128,2.63031881231));
#71733=CARTESIAN_POINT('Ctrl Pts',(10.5420136,-36.2942356128,2.63031881231));
#71734=CARTESIAN_POINT('Ctrl Pts',(10.4735263391,-37.9742356128,2.76337956773));
#71735=CARTESIAN_POINT('Ctrl Pts',(10.4735263391,-36.2942356128,2.76337956773));
#71736=CARTESIAN_POINT('Ctrl Pts',(10.3992001828,-37.9742356128,2.89295886461));
#71737=CARTESIAN_POINT('Ctrl Pts',(10.3992001828,-36.2942356128,2.89295886461));
#71738=CARTESIAN_POINT('Ctrl Pts',(10.3257952821,-37.9742356128,3.01322822759));
#71739=CARTESIAN_POINT('Ctrl Pts',(10.3257952821,-36.2942356128,3.01322822759));
#98282=UNCERTAINTY_MEASURE_WITH_UNIT(LENGTH_MEASURE(0.01),#98303,
'DISTANCE_ACCURACY_VALUE',
'Maximum model space distance between geometric entities at asserted c
onnectivities');
#98290=UNCERTAINTY_MEASURE_WITH_UNIT(LENGTH_MEASURE(0.01),#98303,
'DISTANCE_ACCURACY_VALUE',
'Maximum model space distance between geometric entities at asserted c
onnectivities');
#98294=(
GEOMETRIC_REPRESENTATION_CONTEXT(3)
GLOBAL_UNCERTAINTY_ASSIGNED_CONTEXT((#98282))
GLOBAL_UNIT_ASSIGNED_CONTEXT((#98303,#98305,#98306))
REPRESENTATION_CONTEXT('','3D')
);
#98302=(
GEOMETRIC_REPRESENTATION_CONTEXT(3)
GLOBAL_UNCERTAINTY_ASSIGNED_CONTEXT((#98290))
GLOBAL_UNIT_ASSIGNED_CONTEXT((#98303,#98305,#98306))
REPRESENTATION_CONTEXT('','3D')
);
#98303=(
LENGTH_UNIT()
NAMED_UNIT(*)
SI_UNIT(.MILLI.,.METRE.)
);
#98305=(
NAMED_UNIT(*)
PLANE_ANGLE_UNIT()
SI_UNIT($,.RADIAN.)
);
#98306=(
NAMED_UNIT(*)
SI_UNIT($,.STERADIAN.)
SOLID_ANGLE_UNIT()
);
#98310=SHAPE_DEFINITION_REPRESENTATION(#98321,#98342);
#98321=PRODUCT_DEFINITION_SHAPE('',$,#98354);
#98342=SHAPE_REPRESENTATION('',(#34823),#98294);
#98350=PRODUCT_DEFINITION_CONTEXT('part definition',#98385,'design');
#98354=PRODUCT_DEFINITION('Inner Gasket','Inner Gasket',#98365,#98350);
#98365=PRODUCT_DEFINITION_FORMATION('',$,#98390);
#98385=APPLICATION_CONTEXT(
'Core Data for Automotive Mechanical Design Process');
#98386=PRODUCT_CONTEXT('part definition',#98385,'mechanical');
#98390=PRODUCT('Inner Gasket','Inner Gasket',$,(#98386));
#98399=PRESENTATION_STYLE_ASSIGNMENT((#98401));
#98401=SURFACE_STYLE_USAGE(.BOTH.,#98403);
#98403=SURFACE_SIDE_STYLE('',(#98405));
#98405=SURFACE_STYLE_FILL_AREA(#98407);
#98407=FILL_AREA_STYLE('Opaque(202,209,238)',(#98409));
#98409=FILL_AREA_STYLE_COLOUR('Opaque(202,209,238)',#98411);
#98411=COLOUR_RGB('Opaque(202,209,238)', 0.31764706, 0.68627451, 0.89019608);
ENDSEC;
END-ISO-10303-21;
